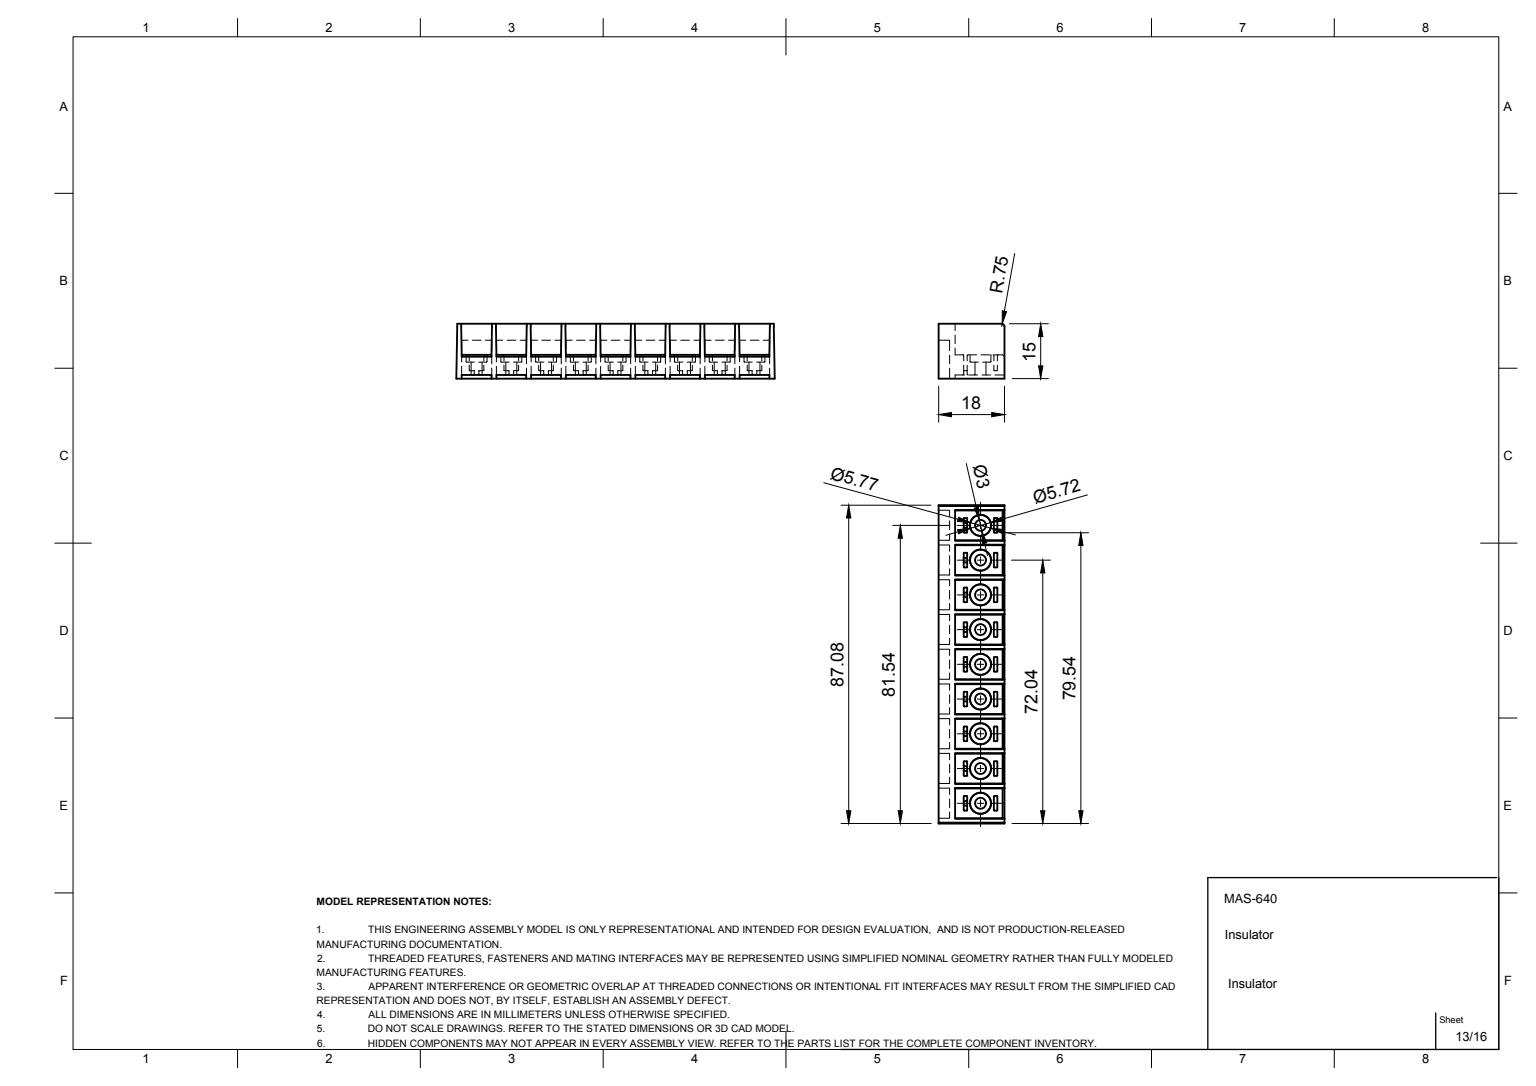
ISO-10303-21;
HEADER;
FILE_DESCRIPTION((''),'2;1');
FILE_NAME('Insulator.step','2026-10-09T10:33:02-07:00',(''),(''),'','','');
FILE_SCHEMA (('AUTOMOTIVE_DESIGN { 1 0 10303 214 3 1 1 }'));
ENDSEC;
DATA;
#10=MECHANICAL_DESIGN_GEOMETRIC_PRESENTATION_REPRESENTATION('',(#842),#86330);
#11=SPHERICAL_SURFACE('',#34725,0.125) ;
#12=SPHERICAL_SURFACE('',#34726,0.125) ;
#13=SPHERICAL_SURFACE('',#34730,0.125) ;
#14=SPHERICAL_SURFACE('',#34731,0.125) ;
#15=SPHERICAL_SURFACE('',#34736,0.125) ;
#16=SPHERICAL_SURFACE('',#34739,0.125) ;
#17=SPHERICAL_SURFACE('',#34750,0.124999999999993) ;
#18=SPHERICAL_SURFACE('',#34751,0.125000000000011) ;
#19=SPHERICAL_SURFACE('',#34781,0.125) ;
#20=SPHERICAL_SURFACE('',#34783,0.125) ;
#21=SPHERICAL_SURFACE('',#34787,0.125) ;
#22=SPHERICAL_SURFACE('',#34789,0.125) ;
#23=SPHERICAL_SURFACE('',#34794,0.125) ;
#24=SPHERICAL_SURFACE('',#34798,0.125) ;
#25=SPHERICAL_SURFACE('',#34810,0.124999999999993) ;
#26=SPHERICAL_SURFACE('',#34811,0.125000000000011) ;
#27=SPHERICAL_SURFACE('',#34841,0.125) ;
#28=SPHERICAL_SURFACE('',#34843,0.125) ;
#29=SPHERICAL_SURFACE('',#34847,0.125) ;
#30=SPHERICAL_SURFACE('',#34849,0.125) ;
#31=SPHERICAL_SURFACE('',#34854,0.125) ;
#32=SPHERICAL_SURFACE('',#34858,0.125) ;
#33=SPHERICAL_SURFACE('',#34870,0.124999999999993) ;
#34=SPHERICAL_SURFACE('',#34871,0.125000000000011) ;
#35=SPHERICAL_SURFACE('',#34901,0.125) ;
#36=SPHERICAL_SURFACE('',#34903,0.125) ;
#37=SPHERICAL_SURFACE('',#34907,0.125) ;
#38=SPHERICAL_SURFACE('',#34909,0.125) ;
#39=SPHERICAL_SURFACE('',#34914,0.125) ;
#40=SPHERICAL_SURFACE('',#34918,0.125) ;
#41=SPHERICAL_SURFACE('',#34930,0.124999999999993) ;
#42=SPHERICAL_SURFACE('',#34931,0.125000000000011) ;
#43=SPHERICAL_SURFACE('',#34961,0.125) ;
#44=SPHERICAL_SURFACE('',#34963,0.125) ;
#45=SPHERICAL_SURFACE('',#34967,0.125) ;
#46=SPHERICAL_SURFACE('',#34969,0.125) ;
#47=SPHERICAL_SURFACE('',#34974,0.125) ;
#48=SPHERICAL_SURFACE('',#34978,0.125) ;
#49=SPHERICAL_SURFACE('',#34990,0.124999999999993) ;
#50=SPHERICAL_SURFACE('',#34991,0.125000000000011) ;
#51=SPHERICAL_SURFACE('',#35021,0.125) ;
#52=SPHERICAL_SURFACE('',#35023,0.125) ;
#53=SPHERICAL_SURFACE('',#35027,0.125) ;
#54=SPHERICAL_SURFACE('',#35029,0.125) ;
#55=SPHERICAL_SURFACE('',#35034,0.125) ;
#56=SPHERICAL_SURFACE('',#35038,0.125) ;
#57=SPHERICAL_SURFACE('',#35050,0.124999999999993) ;
#58=SPHERICAL_SURFACE('',#35051,0.125000000000011) ;
#59=SPHERICAL_SURFACE('',#35081,0.125) ;
#60=SPHERICAL_SURFACE('',#35083,0.125) ;
#61=SPHERICAL_SURFACE('',#35087,0.125) ;
#62=SPHERICAL_SURFACE('',#35089,0.125) ;
#63=SPHERICAL_SURFACE('',#35094,0.125) ;
#64=SPHERICAL_SURFACE('',#35098,0.125) ;
#65=SPHERICAL_SURFACE('',#35110,0.124999999999993) ;
#66=SPHERICAL_SURFACE('',#35111,0.125000000000011) ;
#67=SPHERICAL_SURFACE('',#35141,0.125) ;
#68=SPHERICAL_SURFACE('',#35143,0.125) ;
#69=SPHERICAL_SURFACE('',#35147,0.125) ;
#70=SPHERICAL_SURFACE('',#35149,0.125) ;
#71=SPHERICAL_SURFACE('',#35154,0.125) ;
#72=SPHERICAL_SURFACE('',#35158,0.125) ;
#73=SPHERICAL_SURFACE('',#35170,0.124999999999993) ;
#74=SPHERICAL_SURFACE('',#35171,0.125000000000011) ;
#75=SPHERICAL_SURFACE('',#35201,0.125) ;
#76=SPHERICAL_SURFACE('',#35203,0.125) ;
#77=SPHERICAL_SURFACE('',#35207,0.125) ;
#78=SPHERICAL_SURFACE('',#35209,0.125) ;
#79=SPHERICAL_SURFACE('',#35214,0.125) ;
#80=SPHERICAL_SURFACE('',#35218,0.125) ;
#81=SPHERICAL_SURFACE('',#35230,0.124999999999993) ;
#82=SPHERICAL_SURFACE('',#35231,0.125000000000011) ;
#130=ELLIPSE('',#35261,0.75011424965518,0.750000004857936) ;
#131=ELLIPSE('',#35262,0.750114249654022,0.750000004857117) ;
#132=ELLIPSE('',#35265,0.750114249653564,0.750000004856577) ;
#133=ELLIPSE('',#35266,0.75011424965434,0.750000004857177) ;
#134=ELLIPSE('',#35268,0.750114249655181,0.750000004857937) ;
#135=ELLIPSE('',#35269,0.750114249654116,0.750000004857023) ;
#136=ELLIPSE('',#35271,0.75011424965372,0.750000004856674) ;
#137=ELLIPSE('',#35272,0.75011424965532,0.750000004858217) ;
#138=ELLIPSE('',#35274,0.750114249654022,0.750000004857117) ;
#139=ELLIPSE('',#35275,0.750114249656223,0.750000004858968) ;
#140=ELLIPSE('',#35277,0.750114249654019,0.750000004856718) ;
#141=ELLIPSE('',#35278,0.750114249655222,0.750000004857992) ;
#142=ELLIPSE('',#35280,0.750114249654021,0.750000004856918) ;
#143=ELLIPSE('',#35281,0.750114249656024,0.750000004858698) ;
#144=ELLIPSE('',#35283,0.750114249655273,0.75000000485804) ;
#145=ELLIPSE('',#35284,0.750114249653565,0.75000000485638) ;
#146=ELLIPSE('',#35286,0.750114249654481,0.750000004857962) ;
#147=ELLIPSE('',#35287,0.750114249650677,0.750000004854032) ;
#148=ELLIPSE('',#35289,0.750114249654021,0.750000004856918) ;
#149=ELLIPSE('',#35291,0.750114249654338,0.750000004857176) ;
#239=TOROIDAL_SURFACE('',#33756,1.625,0.125) ;
#240=TOROIDAL_SURFACE('',#33767,1.625,0.125) ;
#241=TOROIDAL_SURFACE('',#33778,1.625,0.125) ;
#242=TOROIDAL_SURFACE('',#33789,1.625,0.125) ;
#243=TOROIDAL_SURFACE('',#33800,1.625,0.125) ;
#244=TOROIDAL_SURFACE('',#33811,1.625,0.125) ;
#245=TOROIDAL_SURFACE('',#33822,1.625,0.125) ;
#246=TOROIDAL_SURFACE('',#33833,1.625,0.125) ;
#247=TOROIDAL_SURFACE('',#33844,1.625,0.125) ;
#248=TOROIDAL_SURFACE('',#33874,0.375,0.25) ;
#249=TOROIDAL_SURFACE('',#33879,0.375,0.25) ;
#250=TOROIDAL_SURFACE('',#33884,0.375,0.25) ;
#251=TOROIDAL_SURFACE('',#33889,0.375,0.25) ;
#252=TOROIDAL_SURFACE('',#33902,0.375,0.25) ;
#253=TOROIDAL_SURFACE('',#33907,0.375,0.25) ;
#254=TOROIDAL_SURFACE('',#33912,0.375,0.25) ;
#255=TOROIDAL_SURFACE('',#33917,0.375,0.25) ;
#256=TOROIDAL_SURFACE('',#33930,0.375,0.25) ;
#257=TOROIDAL_SURFACE('',#33935,0.375,0.25) ;
#258=TOROIDAL_SURFACE('',#33940,0.375,0.25) ;
#259=TOROIDAL_SURFACE('',#33945,0.375,0.25) ;
#260=TOROIDAL_SURFACE('',#33958,0.375,0.25) ;
#261=TOROIDAL_SURFACE('',#33963,0.375,0.25) ;
#262=TOROIDAL_SURFACE('',#33968,0.375,0.25) ;
#263=TOROIDAL_SURFACE('',#33973,0.375,0.25) ;
#264=TOROIDAL_SURFACE('',#33986,0.375,0.25) ;
#265=TOROIDAL_SURFACE('',#33991,0.375,0.25) ;
#266=TOROIDAL_SURFACE('',#33996,0.375,0.25) ;
#267=TOROIDAL_SURFACE('',#34001,0.375,0.25) ;
#268=TOROIDAL_SURFACE('',#34014,0.375,0.25) ;
#269=TOROIDAL_SURFACE('',#34019,0.375,0.25) ;
#270=TOROIDAL_SURFACE('',#34024,0.375,0.25) ;
#271=TOROIDAL_SURFACE('',#34029,0.375,0.25) ;
#272=TOROIDAL_SURFACE('',#34042,0.375,0.25) ;
#273=TOROIDAL_SURFACE('',#34047,0.375,0.25) ;
#274=TOROIDAL_SURFACE('',#34052,0.375,0.25) ;
#275=TOROIDAL_SURFACE('',#34057,0.375,0.25) ;
#276=TOROIDAL_SURFACE('',#34070,0.375,0.25) ;
#277=TOROIDAL_SURFACE('',#34075,0.375,0.25) ;
#278=TOROIDAL_SURFACE('',#34080,0.375,0.25) ;
#279=TOROIDAL_SURFACE('',#34085,0.375,0.25) ;
#280=TOROIDAL_SURFACE('',#34098,0.375,0.25) ;
#281=TOROIDAL_SURFACE('',#34103,0.375,0.25) ;
#282=TOROIDAL_SURFACE('',#34108,0.375,0.25) ;
#283=TOROIDAL_SURFACE('',#34113,0.375,0.25) ;
#284=TOROIDAL_SURFACE('',#34126,0.375,0.25) ;
#285=TOROIDAL_SURFACE('',#34132,0.375,0.25) ;
#286=TOROIDAL_SURFACE('',#34138,0.375,0.25) ;
#287=TOROIDAL_SURFACE('',#34144,0.375,0.25) ;
#288=TOROIDAL_SURFACE('',#34156,0.375,0.25) ;
#289=TOROIDAL_SURFACE('',#34162,0.375,0.25) ;
#290=TOROIDAL_SURFACE('',#34168,0.375,0.25) ;
#291=TOROIDAL_SURFACE('',#34174,0.375,0.25) ;
#292=TOROIDAL_SURFACE('',#34186,0.375,0.25) ;
#293=TOROIDAL_SURFACE('',#34192,0.375,0.25) ;
#294=TOROIDAL_SURFACE('',#34198,0.375,0.25) ;
#295=TOROIDAL_SURFACE('',#34204,0.375,0.25) ;
#296=TOROIDAL_SURFACE('',#34216,0.375,0.25) ;
#297=TOROIDAL_SURFACE('',#34222,0.375,0.25) ;
#298=TOROIDAL_SURFACE('',#34228,0.375,0.25) ;
#299=TOROIDAL_SURFACE('',#34234,0.375,0.25) ;
#300=TOROIDAL_SURFACE('',#34246,0.375,0.25) ;
#301=TOROIDAL_SURFACE('',#34252,0.375,0.25) ;
#302=TOROIDAL_SURFACE('',#34258,0.375,0.25) ;
#303=TOROIDAL_SURFACE('',#34264,0.375,0.25) ;
#304=TOROIDAL_SURFACE('',#34276,0.375,0.25) ;
#305=TOROIDAL_SURFACE('',#34282,0.375,0.25) ;
#306=TOROIDAL_SURFACE('',#34288,0.375,0.25) ;
#307=TOROIDAL_SURFACE('',#34294,0.375,0.25) ;
#308=TOROIDAL_SURFACE('',#34306,0.375,0.25) ;
#309=TOROIDAL_SURFACE('',#34312,0.375,0.25) ;
#310=TOROIDAL_SURFACE('',#34318,0.375,0.25) ;
#311=TOROIDAL_SURFACE('',#34324,0.375,0.25) ;
#312=TOROIDAL_SURFACE('',#34336,0.375,0.25) ;
#313=TOROIDAL_SURFACE('',#34342,0.375,0.25) ;
#314=TOROIDAL_SURFACE('',#34348,0.375,0.25) ;
#315=TOROIDAL_SURFACE('',#34354,0.375,0.25) ;
#316=TOROIDAL_SURFACE('',#34366,0.375,0.25) ;
#317=TOROIDAL_SURFACE('',#34372,0.375,0.25) ;
#318=TOROIDAL_SURFACE('',#34378,0.375,0.25) ;
#319=TOROIDAL_SURFACE('',#34384,0.375,0.25) ;
#320=TOROIDAL_SURFACE('',#34398,0.375,0.25) ;
#321=TOROIDAL_SURFACE('',#34404,0.375,0.25) ;
#322=TOROIDAL_SURFACE('',#34410,0.375,0.25) ;
#323=TOROIDAL_SURFACE('',#34416,0.375,0.25) ;
#324=TOROIDAL_SURFACE('',#34430,0.375,0.25) ;
#325=TOROIDAL_SURFACE('',#34436,0.375,0.25) ;
#326=TOROIDAL_SURFACE('',#34442,0.375,0.25) ;
#327=TOROIDAL_SURFACE('',#34448,0.375,0.25) ;
#328=TOROIDAL_SURFACE('',#34462,0.375,0.25) ;
#329=TOROIDAL_SURFACE('',#34468,0.375,0.25) ;
#330=TOROIDAL_SURFACE('',#34474,0.375,0.25) ;
#331=TOROIDAL_SURFACE('',#34480,0.375,0.25) ;
#332=TOROIDAL_SURFACE('',#34494,0.375,0.25) ;
#333=TOROIDAL_SURFACE('',#34500,0.375,0.25) ;
#334=TOROIDAL_SURFACE('',#34506,0.375,0.25) ;
#335=TOROIDAL_SURFACE('',#34512,0.375,0.25) ;
#336=TOROIDAL_SURFACE('',#34526,0.375,0.25) ;
#337=TOROIDAL_SURFACE('',#34532,0.375,0.25) ;
#338=TOROIDAL_SURFACE('',#34538,0.375,0.25) ;
#339=TOROIDAL_SURFACE('',#34544,0.375,0.25) ;
#340=TOROIDAL_SURFACE('',#34558,0.375,0.25) ;
#341=TOROIDAL_SURFACE('',#34564,0.375,0.25) ;
#342=TOROIDAL_SURFACE('',#34570,0.375,0.25) ;
#343=TOROIDAL_SURFACE('',#34576,0.375,0.25) ;
#344=TOROIDAL_SURFACE('',#34590,0.375,0.25) ;
#345=TOROIDAL_SURFACE('',#34596,0.375,0.25) ;
#346=TOROIDAL_SURFACE('',#34602,0.375,0.25) ;
#347=TOROIDAL_SURFACE('',#34608,0.375,0.25) ;
#348=TOROIDAL_SURFACE('',#34622,0.375,0.25) ;
#349=TOROIDAL_SURFACE('',#34628,0.375,0.25) ;
#350=TOROIDAL_SURFACE('',#34634,0.375,0.25) ;
#351=TOROIDAL_SURFACE('',#34640,0.375,0.25) ;
#352=TOROIDAL_SURFACE('',#34658,0.375,0.25) ;
#353=TOROIDAL_SURFACE('',#34663,0.375,0.25) ;
#354=TOROIDAL_SURFACE('',#34668,0.375,0.25) ;
#355=TOROIDAL_SURFACE('',#34673,0.375,0.25) ;
#356=TOROIDAL_SURFACE('',#34701,0.188499999999969,0.124999999999993) ;
#357=TOROIDAL_SURFACE('',#34706,0.188499999999987,0.124999999999993) ;
#358=TOROIDAL_SURFACE('',#34709,0.188499999999987,0.124999999999993) ;
#359=TOROIDAL_SURFACE('',#34716,0.188499999999987,0.124999999999993) ;
#360=TOROIDAL_SURFACE('',#34757,0.188499999999969,0.124999999999993) ;
#361=TOROIDAL_SURFACE('',#34762,0.188499999999987,0.124999999999993) ;
#362=TOROIDAL_SURFACE('',#34765,0.188499999999987,0.124999999999993) ;
#363=TOROIDAL_SURFACE('',#34772,0.188499999999987,0.124999999999993) ;
#364=TOROIDAL_SURFACE('',#34817,0.188499999999969,0.124999999999993) ;
#365=TOROIDAL_SURFACE('',#34822,0.188499999999987,0.124999999999993) ;
#366=TOROIDAL_SURFACE('',#34825,0.188499999999987,0.124999999999993) ;
#367=TOROIDAL_SURFACE('',#34832,0.188499999999987,0.124999999999993) ;
#368=TOROIDAL_SURFACE('',#34877,0.188499999999969,0.124999999999993) ;
#369=TOROIDAL_SURFACE('',#34882,0.188499999999987,0.124999999999993) ;
#370=TOROIDAL_SURFACE('',#34885,0.188499999999987,0.124999999999993) ;
#371=TOROIDAL_SURFACE('',#34892,0.188499999999987,0.124999999999993) ;
#372=TOROIDAL_SURFACE('',#34937,0.188499999999969,0.124999999999993) ;
#373=TOROIDAL_SURFACE('',#34942,0.188499999999987,0.124999999999993) ;
#374=TOROIDAL_SURFACE('',#34945,0.188499999999987,0.124999999999993) ;
#375=TOROIDAL_SURFACE('',#34952,0.188499999999987,0.124999999999993) ;
#376=TOROIDAL_SURFACE('',#34997,0.188499999999969,0.124999999999993) ;
#377=TOROIDAL_SURFACE('',#35002,0.188499999999987,0.124999999999993) ;
#378=TOROIDAL_SURFACE('',#35005,0.188499999999987,0.124999999999993) ;
#379=TOROIDAL_SURFACE('',#35012,0.188499999999987,0.124999999999993) ;
#380=TOROIDAL_SURFACE('',#35057,0.188499999999969,0.124999999999993) ;
#381=TOROIDAL_SURFACE('',#35062,0.188499999999987,0.124999999999993) ;
#382=TOROIDAL_SURFACE('',#35065,0.188499999999987,0.124999999999993) ;
#383=TOROIDAL_SURFACE('',#35072,0.188499999999987,0.124999999999993) ;
#384=TOROIDAL_SURFACE('',#35117,0.188499999999969,0.124999999999993) ;
#385=TOROIDAL_SURFACE('',#35122,0.188499999999987,0.124999999999993) ;
#386=TOROIDAL_SURFACE('',#35125,0.188499999999987,0.124999999999993) ;
#387=TOROIDAL_SURFACE('',#35132,0.188499999999987,0.124999999999993) ;
#388=TOROIDAL_SURFACE('',#35177,0.188499999999969,0.124999999999993) ;
#389=TOROIDAL_SURFACE('',#35182,0.188499999999987,0.124999999999993) ;
#390=TOROIDAL_SURFACE('',#35185,0.188499999999987,0.124999999999993) ;
#391=TOROIDAL_SURFACE('',#35192,0.188499999999987,0.124999999999993) ;
#392=TOROIDAL_SURFACE('',#35330,2.9825,0.125) ;
#393=TOROIDAL_SURFACE('',#35336,2.7325,0.125) ;
#394=TOROIDAL_SURFACE('',#35342,2.9825,0.125) ;
#395=TOROIDAL_SURFACE('',#35348,2.7325,0.125) ;
#396=TOROIDAL_SURFACE('',#35354,2.9825,0.125) ;
#397=TOROIDAL_SURFACE('',#35360,2.7325,0.125) ;
#398=TOROIDAL_SURFACE('',#35366,2.9825,0.125) ;
#399=TOROIDAL_SURFACE('',#35372,2.7325,0.125) ;
#400=TOROIDAL_SURFACE('',#35378,2.9825,0.125) ;
#401=TOROIDAL_SURFACE('',#35384,2.7325,0.125) ;
#402=TOROIDAL_SURFACE('',#35390,2.9825,0.125) ;
#403=TOROIDAL_SURFACE('',#35396,2.7325,0.125) ;
#404=TOROIDAL_SURFACE('',#35402,2.9825,0.125) ;
#405=TOROIDAL_SURFACE('',#35408,2.7325,0.125) ;
#406=TOROIDAL_SURFACE('',#35414,2.9825,0.125) ;
#407=TOROIDAL_SURFACE('',#35420,2.7325,0.125) ;
#408=TOROIDAL_SURFACE('',#35424,2.9825,0.125) ;
#409=TOROIDAL_SURFACE('',#35430,2.7325,0.125) ;
#818=SHAPE_REPRESENTATION_RELATIONSHIP('SRR','None',#86461,#830) ;
#830=ADVANCED_BREP_SHAPE_REPRESENTATION('',(#854),#86315) ;
#842=STYLED_ITEM('',(#86583),#854) ;
#854=MANIFOLD_SOLID_BREP('Body1',#32641) ;
#1115=FACE_BOUND('',#4823,.T.) ;
#1116=FACE_BOUND('',#4824,.T.) ;
#1117=FACE_BOUND('',#4828,.T.) ;
#1118=FACE_BOUND('',#4829,.T.) ;
#1119=FACE_BOUND('',#4833,.T.) ;
#1120=FACE_BOUND('',#4834,.T.) ;
#1121=FACE_BOUND('',#4838,.T.) ;
#1122=FACE_BOUND('',#4839,.T.) ;
#1123=FACE_BOUND('',#4843,.T.) ;
#1124=FACE_BOUND('',#4844,.T.) ;
#1125=FACE_BOUND('',#4848,.T.) ;
#1126=FACE_BOUND('',#4849,.T.) ;
#1127=FACE_BOUND('',#4853,.T.) ;
#1128=FACE_BOUND('',#4854,.T.) ;
#1129=FACE_BOUND('',#4858,.T.) ;
#1130=FACE_BOUND('',#4859,.T.) ;
#1131=FACE_BOUND('',#4862,.T.) ;
#1132=FACE_BOUND('',#4863,.T.) ;
#1133=FACE_BOUND('',#4866,.T.) ;
#1134=FACE_BOUND('',#4868,.T.) ;
#1135=FACE_BOUND('',#4870,.T.) ;
#1136=FACE_BOUND('',#4872,.T.) ;
#1137=FACE_BOUND('',#4874,.T.) ;
#1138=FACE_BOUND('',#4876,.T.) ;
#1139=FACE_BOUND('',#4878,.T.) ;
#1140=FACE_BOUND('',#4880,.T.) ;
#1141=FACE_BOUND('',#5194,.T.) ;
#1142=FACE_BOUND('',#5195,.T.) ;
#1143=FACE_BOUND('',#5196,.T.) ;
#1144=FACE_BOUND('',#5217,.T.) ;
#1145=FACE_BOUND('',#5565,.T.) ;
#1146=FACE_BOUND('',#5566,.T.) ;
#1147=FACE_BOUND('',#5567,.T.) ;
#1148=FACE_BOUND('',#5574,.T.) ;
#1149=FACE_BOUND('',#5575,.T.) ;
#1150=FACE_BOUND('',#5576,.T.) ;
#1151=FACE_BOUND('',#5583,.T.) ;
#1152=FACE_BOUND('',#5584,.T.) ;
#1153=FACE_BOUND('',#5585,.T.) ;
#1154=FACE_BOUND('',#5592,.T.) ;
#1155=FACE_BOUND('',#5593,.T.) ;
#1156=FACE_BOUND('',#5594,.T.) ;
#1157=FACE_BOUND('',#5601,.T.) ;
#1158=FACE_BOUND('',#5602,.T.) ;
#1159=FACE_BOUND('',#5603,.T.) ;
#1160=FACE_BOUND('',#5610,.T.) ;
#1161=FACE_BOUND('',#5611,.T.) ;
#1162=FACE_BOUND('',#5612,.T.) ;
#1163=FACE_BOUND('',#5619,.T.) ;
#1164=FACE_BOUND('',#5620,.T.) ;
#1165=FACE_BOUND('',#5621,.T.) ;
#1166=FACE_BOUND('',#5628,.T.) ;
#1167=FACE_BOUND('',#5629,.T.) ;
#1168=FACE_BOUND('',#5630,.T.) ;
#1899=PLANE('',#33719) ;
#1900=PLANE('',#33720) ;
#1901=PLANE('',#33721) ;
#1902=PLANE('',#33722) ;
#1903=PLANE('',#33723) ;
#1904=PLANE('',#33724) ;
#1905=PLANE('',#33725) ;
#1906=PLANE('',#33726) ;
#1907=PLANE('',#33727) ;
#1908=PLANE('',#33728) ;
#1909=PLANE('',#33729) ;
#1910=PLANE('',#33730) ;
#1911=PLANE('',#33731) ;
#1912=PLANE('',#33732) ;
#1913=PLANE('',#33733) ;
#1914=PLANE('',#33734) ;
#1915=PLANE('',#33735) ;
#1916=PLANE('',#33736) ;
#1917=PLANE('',#33737) ;
#1918=PLANE('',#33738) ;
#1919=PLANE('',#33739) ;
#1920=PLANE('',#33740) ;
#1921=PLANE('',#33741) ;
#1922=PLANE('',#33742) ;
#1923=PLANE('',#33743) ;
#1924=PLANE('',#33744) ;
#1925=PLANE('',#33745) ;
#1926=PLANE('',#33746) ;
#1927=PLANE('',#33747) ;
#1928=PLANE('',#33748) ;
#1929=PLANE('',#33749) ;
#1930=PLANE('',#33750) ;
#1931=PLANE('',#33751) ;
#1932=PLANE('',#33752) ;
#1933=PLANE('',#33753) ;
#1934=PLANE('',#33754) ;
#1935=PLANE('',#33755) ;
#1936=PLANE('',#33762) ;
#1937=PLANE('',#33773) ;
#1938=PLANE('',#33784) ;
#1939=PLANE('',#33795) ;
#1940=PLANE('',#33806) ;
#1941=PLANE('',#33817) ;
#1942=PLANE('',#33828) ;
#1943=PLANE('',#33839) ;
#1944=PLANE('',#33848) ;
#1945=PLANE('',#33855) ;
#1946=PLANE('',#33857) ;
#1947=PLANE('',#33859) ;
#1948=PLANE('',#33861) ;
#1949=PLANE('',#33863) ;
#1950=PLANE('',#33865) ;
#1951=PLANE('',#33867) ;
#1952=PLANE('',#33869) ;
#1953=PLANE('',#33893) ;
#1954=PLANE('',#33898) ;
#1955=PLANE('',#33921) ;
#1956=PLANE('',#33926) ;
#1957=PLANE('',#33949) ;
#1958=PLANE('',#33954) ;
#1959=PLANE('',#33977) ;
#1960=PLANE('',#33982) ;
#1961=PLANE('',#34005) ;
#1962=PLANE('',#34010) ;
#1963=PLANE('',#34033) ;
#1964=PLANE('',#34038) ;
#1965=PLANE('',#34061) ;
#1966=PLANE('',#34066) ;
#1967=PLANE('',#34089) ;
#1968=PLANE('',#34094) ;
#1969=PLANE('',#34117) ;
#1970=PLANE('',#34122) ;
#1971=PLANE('',#34149) ;
#1972=PLANE('',#34152) ;
#1973=PLANE('',#34179) ;
#1974=PLANE('',#34182) ;
#1975=PLANE('',#34209) ;
#1976=PLANE('',#34212) ;
#1977=PLANE('',#34239) ;
#1978=PLANE('',#34242) ;
#1979=PLANE('',#34269) ;
#1980=PLANE('',#34272) ;
#1981=PLANE('',#34299) ;
#1982=PLANE('',#34302) ;
#1983=PLANE('',#34329) ;
#1984=PLANE('',#34332) ;
#1985=PLANE('',#34359) ;
#1986=PLANE('',#34362) ;
#1987=PLANE('',#34389) ;
#1988=PLANE('',#34394) ;
#1989=PLANE('',#34421) ;
#1990=PLANE('',#34426) ;
#1991=PLANE('',#34453) ;
#1992=PLANE('',#34458) ;
#1993=PLANE('',#34485) ;
#1994=PLANE('',#34490) ;
#1995=PLANE('',#34517) ;
#1996=PLANE('',#34522) ;
#1997=PLANE('',#34549) ;
#1998=PLANE('',#34554) ;
#1999=PLANE('',#34581) ;
#2000=PLANE('',#34586) ;
#2001=PLANE('',#34613) ;
#2002=PLANE('',#34618) ;
#2003=PLANE('',#34645) ;
#2004=PLANE('',#34648) ;
#2005=PLANE('',#34649) ;
#2006=PLANE('',#34677) ;
#2007=PLANE('',#34682) ;
#2008=PLANE('',#34683) ;
#2009=PLANE('',#34688) ;
#2010=PLANE('',#34693) ;
#2011=PLANE('',#34694) ;
#2012=PLANE('',#34732) ;
#2013=PLANE('',#34733) ;
#2014=PLANE('',#34734) ;
#2015=PLANE('',#34735) ;
#2016=PLANE('',#34790) ;
#2017=PLANE('',#34791) ;
#2018=PLANE('',#34792) ;
#2019=PLANE('',#34793) ;
#2020=PLANE('',#34850) ;
#2021=PLANE('',#34851) ;
#2022=PLANE('',#34852) ;
#2023=PLANE('',#34853) ;
#2024=PLANE('',#34910) ;
#2025=PLANE('',#34911) ;
#2026=PLANE('',#34912) ;
#2027=PLANE('',#34913) ;
#2028=PLANE('',#34970) ;
#2029=PLANE('',#34971) ;
#2030=PLANE('',#34972) ;
#2031=PLANE('',#34973) ;
#2032=PLANE('',#35030) ;
#2033=PLANE('',#35031) ;
#2034=PLANE('',#35032) ;
#2035=PLANE('',#35033) ;
#2036=PLANE('',#35090) ;
#2037=PLANE('',#35091) ;
#2038=PLANE('',#35092) ;
#2039=PLANE('',#35093) ;
#2040=PLANE('',#35150) ;
#2041=PLANE('',#35151) ;
#2042=PLANE('',#35152) ;
#2043=PLANE('',#35153) ;
#2044=PLANE('',#35210) ;
#2045=PLANE('',#35211) ;
#2046=PLANE('',#35212) ;
#2047=PLANE('',#35213) ;
#2048=PLANE('',#35232) ;
#2049=PLANE('',#35233) ;
#2050=PLANE('',#35234) ;
#2051=PLANE('',#35235) ;
#2052=PLANE('',#35236) ;
#2053=PLANE('',#35237) ;
#2054=PLANE('',#35238) ;
#2055=PLANE('',#35239) ;
#2056=PLANE('',#35240) ;
#2057=PLANE('',#35241) ;
#2058=PLANE('',#35242) ;
#2059=PLANE('',#35243) ;
#2060=PLANE('',#35244) ;
#2061=PLANE('',#35245) ;
#2062=PLANE('',#35246) ;
#2063=PLANE('',#35247) ;
#2064=PLANE('',#35248) ;
#2065=PLANE('',#35249) ;
#2066=PLANE('',#35250) ;
#2067=PLANE('',#35251) ;
#2068=PLANE('',#35252) ;
#2069=PLANE('',#35253) ;
#2070=PLANE('',#35254) ;
#2071=PLANE('',#35255) ;
#2072=PLANE('',#35256) ;
#2073=PLANE('',#35257) ;
#2074=PLANE('',#35258) ;
#2075=PLANE('',#35259) ;
#2076=PLANE('',#35263) ;
#2077=PLANE('',#35288) ;
#2078=PLANE('',#35292) ;
#2079=PLANE('',#35293) ;
#2080=PLANE('',#35294) ;
#2081=PLANE('',#35295) ;
#2082=PLANE('',#35296) ;
#2083=PLANE('',#35297) ;
#2084=PLANE('',#35298) ;
#2085=PLANE('',#35299) ;
#2086=PLANE('',#35300) ;
#2087=PLANE('',#35301) ;
#2088=PLANE('',#35302) ;
#2089=PLANE('',#35303) ;
#2090=PLANE('',#35304) ;
#2091=PLANE('',#35305) ;
#2092=PLANE('',#35306) ;
#2093=PLANE('',#35307) ;
#2094=PLANE('',#35308) ;
#2095=PLANE('',#35309) ;
#2096=PLANE('',#35310) ;
#2097=PLANE('',#35311) ;
#2098=PLANE('',#35312) ;
#2099=PLANE('',#35313) ;
#2100=PLANE('',#35314) ;
#2101=PLANE('',#35315) ;
#2102=PLANE('',#35316) ;
#2103=PLANE('',#35317) ;
#2104=PLANE('',#35318) ;
#2105=PLANE('',#35319) ;
#2106=PLANE('',#35320) ;
#2107=PLANE('',#35321) ;
#2108=PLANE('',#35322) ;
#2109=PLANE('',#35323) ;
#2110=PLANE('',#35324) ;
#2111=PLANE('',#35325) ;
#2112=PLANE('',#35326) ;
#2113=PLANE('',#35327) ;
#2114=PLANE('',#35328) ;
#2115=PLANE('',#35338) ;
#2116=PLANE('',#35340) ;
#2117=PLANE('',#35350) ;
#2118=PLANE('',#35352) ;
#2119=PLANE('',#35362) ;
#2120=PLANE('',#35364) ;
#2121=PLANE('',#35374) ;
#2122=PLANE('',#35376) ;
#2123=PLANE('',#35386) ;
#2124=PLANE('',#35388) ;
#2125=PLANE('',#35398) ;
#2126=PLANE('',#35400) ;
#2127=PLANE('',#35410) ;
#2128=PLANE('',#35412) ;
#2129=PLANE('',#35422) ;
#2130=PLANE('',#35432) ;
#2131=PLANE('',#35433) ;
#2132=PLANE('',#35435) ;
#2133=PLANE('',#35437) ;
#2134=PLANE('',#35440) ;
#2135=PLANE('',#35442) ;
#2136=PLANE('',#35445) ;
#2137=PLANE('',#35447) ;
#2138=PLANE('',#35450) ;
#2139=PLANE('',#35452) ;
#2140=PLANE('',#35455) ;
#2141=PLANE('',#35457) ;
#2142=PLANE('',#35460) ;
#2143=PLANE('',#35462) ;
#2144=PLANE('',#35465) ;
#2145=PLANE('',#35467) ;
#2146=PLANE('',#35470) ;
#2147=PLANE('',#35472) ;
#2780=FACE_OUTER_BOUND('',#4783,.T.) ;
#2781=FACE_OUTER_BOUND('',#4784,.T.) ;
#2782=FACE_OUTER_BOUND('',#4785,.T.) ;
#2783=FACE_OUTER_BOUND('',#4786,.T.) ;
#2784=FACE_OUTER_BOUND('',#4787,.T.) ;
#2785=FACE_OUTER_BOUND('',#4788,.T.) ;
#2786=FACE_OUTER_BOUND('',#4789,.T.) ;
#2787=FACE_OUTER_BOUND('',#4790,.T.) ;
#2788=FACE_OUTER_BOUND('',#4791,.T.) ;
#2789=FACE_OUTER_BOUND('',#4792,.T.) ;
#2790=FACE_OUTER_BOUND('',#4793,.T.) ;
#2791=FACE_OUTER_BOUND('',#4794,.T.) ;
#2792=FACE_OUTER_BOUND('',#4795,.T.) ;
#2793=FACE_OUTER_BOUND('',#4796,.T.) ;
#2794=FACE_OUTER_BOUND('',#4797,.T.) ;
#2795=FACE_OUTER_BOUND('',#4798,.T.) ;
#2796=FACE_OUTER_BOUND('',#4799,.T.) ;
#2797=FACE_OUTER_BOUND('',#4800,.T.) ;
#2798=FACE_OUTER_BOUND('',#4801,.T.) ;
#2799=FACE_OUTER_BOUND('',#4802,.T.) ;
#2800=FACE_OUTER_BOUND('',#4803,.T.) ;
#2801=FACE_OUTER_BOUND('',#4804,.T.) ;
#2802=FACE_OUTER_BOUND('',#4805,.T.) ;
#2803=FACE_OUTER_BOUND('',#4806,.T.) ;
#2804=FACE_OUTER_BOUND('',#4807,.T.) ;
#2805=FACE_OUTER_BOUND('',#4808,.T.) ;
#2806=FACE_OUTER_BOUND('',#4809,.T.) ;
#2807=FACE_OUTER_BOUND('',#4810,.T.) ;
#2808=FACE_OUTER_BOUND('',#4811,.T.) ;
#2809=FACE_OUTER_BOUND('',#4812,.T.) ;
#2810=FACE_OUTER_BOUND('',#4813,.T.) ;
#2811=FACE_OUTER_BOUND('',#4814,.T.) ;
#2812=FACE_OUTER_BOUND('',#4815,.T.) ;
#2813=FACE_OUTER_BOUND('',#4816,.T.) ;
#2814=FACE_OUTER_BOUND('',#4817,.T.) ;
#2815=FACE_OUTER_BOUND('',#4818,.T.) ;
#2816=FACE_OUTER_BOUND('',#4819,.T.) ;
#2817=FACE_OUTER_BOUND('',#4820,.T.) ;
#2818=FACE_OUTER_BOUND('',#4821,.T.) ;
#2819=FACE_OUTER_BOUND('',#4822,.T.) ;
#2820=FACE_OUTER_BOUND('',#4825,.T.) ;
#2821=FACE_OUTER_BOUND('',#4826,.T.) ;
#2822=FACE_OUTER_BOUND('',#4827,.T.) ;
#2823=FACE_OUTER_BOUND('',#4830,.T.) ;
#2824=FACE_OUTER_BOUND('',#4831,.T.) ;
#2825=FACE_OUTER_BOUND('',#4832,.T.) ;
#2826=FACE_OUTER_BOUND('',#4835,.T.) ;
#2827=FACE_OUTER_BOUND('',#4836,.T.) ;
#2828=FACE_OUTER_BOUND('',#4837,.T.) ;
#2829=FACE_OUTER_BOUND('',#4840,.T.) ;
#2830=FACE_OUTER_BOUND('',#4841,.T.) ;
#2831=FACE_OUTER_BOUND('',#4842,.T.) ;
#2832=FACE_OUTER_BOUND('',#4845,.T.) ;
#2833=FACE_OUTER_BOUND('',#4846,.T.) ;
#2834=FACE_OUTER_BOUND('',#4847,.T.) ;
#2835=FACE_OUTER_BOUND('',#4850,.T.) ;
#2836=FACE_OUTER_BOUND('',#4851,.T.) ;
#2837=FACE_OUTER_BOUND('',#4852,.T.) ;
#2838=FACE_OUTER_BOUND('',#4855,.T.) ;
#2839=FACE_OUTER_BOUND('',#4856,.T.) ;
#2840=FACE_OUTER_BOUND('',#4857,.T.) ;
#2841=FACE_OUTER_BOUND('',#4860,.T.) ;
#2842=FACE_OUTER_BOUND('',#4861,.T.) ;
#2843=FACE_OUTER_BOUND('',#4864,.T.) ;
#2844=FACE_OUTER_BOUND('',#4865,.T.) ;
#2845=FACE_OUTER_BOUND('',#4867,.T.) ;
#2846=FACE_OUTER_BOUND('',#4869,.T.) ;
#2847=FACE_OUTER_BOUND('',#4871,.T.) ;
#2848=FACE_OUTER_BOUND('',#4873,.T.) ;
#2849=FACE_OUTER_BOUND('',#4875,.T.) ;
#2850=FACE_OUTER_BOUND('',#4877,.T.) ;
#2851=FACE_OUTER_BOUND('',#4879,.T.) ;
#2852=FACE_OUTER_BOUND('',#4881,.T.) ;
#2853=FACE_OUTER_BOUND('',#4882,.T.) ;
#2854=FACE_OUTER_BOUND('',#4883,.T.) ;
#2855=FACE_OUTER_BOUND('',#4884,.T.) ;
#2856=FACE_OUTER_BOUND('',#4885,.T.) ;
#2857=FACE_OUTER_BOUND('',#4886,.T.) ;
#2858=FACE_OUTER_BOUND('',#4887,.T.) ;
#2859=FACE_OUTER_BOUND('',#4888,.T.) ;
#2860=FACE_OUTER_BOUND('',#4889,.T.) ;
#2861=FACE_OUTER_BOUND('',#4890,.T.) ;
#2862=FACE_OUTER_BOUND('',#4891,.T.) ;
#2863=FACE_OUTER_BOUND('',#4892,.T.) ;
#2864=FACE_OUTER_BOUND('',#4893,.T.) ;
#2865=FACE_OUTER_BOUND('',#4894,.T.) ;
#2866=FACE_OUTER_BOUND('',#4895,.T.) ;
#2867=FACE_OUTER_BOUND('',#4896,.T.) ;
#2868=FACE_OUTER_BOUND('',#4897,.T.) ;
#2869=FACE_OUTER_BOUND('',#4898,.T.) ;
#2870=FACE_OUTER_BOUND('',#4899,.T.) ;
#2871=FACE_OUTER_BOUND('',#4900,.T.) ;
#2872=FACE_OUTER_BOUND('',#4901,.T.) ;
#2873=FACE_OUTER_BOUND('',#4902,.T.) ;
#2874=FACE_OUTER_BOUND('',#4903,.T.) ;
#2875=FACE_OUTER_BOUND('',#4904,.T.) ;
#2876=FACE_OUTER_BOUND('',#4905,.T.) ;
#2877=FACE_OUTER_BOUND('',#4906,.T.) ;
#2878=FACE_OUTER_BOUND('',#4907,.T.) ;
#2879=FACE_OUTER_BOUND('',#4908,.T.) ;
#2880=FACE_OUTER_BOUND('',#4909,.T.) ;
#2881=FACE_OUTER_BOUND('',#4910,.T.) ;
#2882=FACE_OUTER_BOUND('',#4911,.T.) ;
#2883=FACE_OUTER_BOUND('',#4912,.T.) ;
#2884=FACE_OUTER_BOUND('',#4913,.T.) ;
#2885=FACE_OUTER_BOUND('',#4914,.T.) ;
#2886=FACE_OUTER_BOUND('',#4915,.T.) ;
#2887=FACE_OUTER_BOUND('',#4916,.T.) ;
#2888=FACE_OUTER_BOUND('',#4917,.T.) ;
#2889=FACE_OUTER_BOUND('',#4918,.T.) ;
#2890=FACE_OUTER_BOUND('',#4919,.T.) ;
#2891=FACE_OUTER_BOUND('',#4920,.T.) ;
#2892=FACE_OUTER_BOUND('',#4921,.T.) ;
#2893=FACE_OUTER_BOUND('',#4922,.T.) ;
#2894=FACE_OUTER_BOUND('',#4923,.T.) ;
#2895=FACE_OUTER_BOUND('',#4924,.T.) ;
#2896=FACE_OUTER_BOUND('',#4925,.T.) ;
#2897=FACE_OUTER_BOUND('',#4926,.T.) ;
#2898=FACE_OUTER_BOUND('',#4927,.T.) ;
#2899=FACE_OUTER_BOUND('',#4928,.T.) ;
#2900=FACE_OUTER_BOUND('',#4929,.T.) ;
#2901=FACE_OUTER_BOUND('',#4930,.T.) ;
#2902=FACE_OUTER_BOUND('',#4931,.T.) ;
#2903=FACE_OUTER_BOUND('',#4932,.T.) ;
#2904=FACE_OUTER_BOUND('',#4933,.T.) ;
#2905=FACE_OUTER_BOUND('',#4934,.T.) ;
#2906=FACE_OUTER_BOUND('',#4935,.T.) ;
#2907=FACE_OUTER_BOUND('',#4936,.T.) ;
#2908=FACE_OUTER_BOUND('',#4937,.T.) ;
#2909=FACE_OUTER_BOUND('',#4938,.T.) ;
#2910=FACE_OUTER_BOUND('',#4939,.T.) ;
#2911=FACE_OUTER_BOUND('',#4940,.T.) ;
#2912=FACE_OUTER_BOUND('',#4941,.T.) ;
#2913=FACE_OUTER_BOUND('',#4942,.T.) ;
#2914=FACE_OUTER_BOUND('',#4943,.T.) ;
#2915=FACE_OUTER_BOUND('',#4944,.T.) ;
#2916=FACE_OUTER_BOUND('',#4945,.T.) ;
#2917=FACE_OUTER_BOUND('',#4946,.T.) ;
#2918=FACE_OUTER_BOUND('',#4947,.T.) ;
#2919=FACE_OUTER_BOUND('',#4948,.T.) ;
#2920=FACE_OUTER_BOUND('',#4949,.T.) ;
#2921=FACE_OUTER_BOUND('',#4950,.T.) ;
#2922=FACE_OUTER_BOUND('',#4951,.T.) ;
#2923=FACE_OUTER_BOUND('',#4952,.T.) ;
#2924=FACE_OUTER_BOUND('',#4953,.T.) ;
#2925=FACE_OUTER_BOUND('',#4954,.T.) ;
#2926=FACE_OUTER_BOUND('',#4955,.T.) ;
#2927=FACE_OUTER_BOUND('',#4956,.T.) ;
#2928=FACE_OUTER_BOUND('',#4957,.T.) ;
#2929=FACE_OUTER_BOUND('',#4958,.T.) ;
#2930=FACE_OUTER_BOUND('',#4959,.T.) ;
#2931=FACE_OUTER_BOUND('',#4960,.T.) ;
#2932=FACE_OUTER_BOUND('',#4961,.T.) ;
#2933=FACE_OUTER_BOUND('',#4962,.T.) ;
#2934=FACE_OUTER_BOUND('',#4963,.T.) ;
#2935=FACE_OUTER_BOUND('',#4964,.T.) ;
#2936=FACE_OUTER_BOUND('',#4965,.T.) ;
#2937=FACE_OUTER_BOUND('',#4966,.T.) ;
#2938=FACE_OUTER_BOUND('',#4967,.T.) ;
#2939=FACE_OUTER_BOUND('',#4968,.T.) ;
#2940=FACE_OUTER_BOUND('',#4969,.T.) ;
#2941=FACE_OUTER_BOUND('',#4970,.T.) ;
#2942=FACE_OUTER_BOUND('',#4971,.T.) ;
#2943=FACE_OUTER_BOUND('',#4972,.T.) ;
#2944=FACE_OUTER_BOUND('',#4973,.T.) ;
#2945=FACE_OUTER_BOUND('',#4974,.T.) ;
#2946=FACE_OUTER_BOUND('',#4975,.T.) ;
#2947=FACE_OUTER_BOUND('',#4976,.T.) ;
#2948=FACE_OUTER_BOUND('',#4977,.T.) ;
#2949=FACE_OUTER_BOUND('',#4978,.T.) ;
#2950=FACE_OUTER_BOUND('',#4979,.T.) ;
#2951=FACE_OUTER_BOUND('',#4980,.T.) ;
#2952=FACE_OUTER_BOUND('',#4981,.T.) ;
#2953=FACE_OUTER_BOUND('',#4982,.T.) ;
#2954=FACE_OUTER_BOUND('',#4983,.T.) ;
#2955=FACE_OUTER_BOUND('',#4984,.T.) ;
#2956=FACE_OUTER_BOUND('',#4985,.T.) ;
#2957=FACE_OUTER_BOUND('',#4986,.T.) ;
#2958=FACE_OUTER_BOUND('',#4987,.T.) ;
#2959=FACE_OUTER_BOUND('',#4988,.T.) ;
#2960=FACE_OUTER_BOUND('',#4989,.T.) ;
#2961=FACE_OUTER_BOUND('',#4990,.T.) ;
#2962=FACE_OUTER_BOUND('',#4991,.T.) ;
#2963=FACE_OUTER_BOUND('',#4992,.T.) ;
#2964=FACE_OUTER_BOUND('',#4993,.T.) ;
#2965=FACE_OUTER_BOUND('',#4994,.T.) ;
#2966=FACE_OUTER_BOUND('',#4995,.T.) ;
#2967=FACE_OUTER_BOUND('',#4996,.T.) ;
#2968=FACE_OUTER_BOUND('',#4997,.T.) ;
#2969=FACE_OUTER_BOUND('',#4998,.T.) ;
#2970=FACE_OUTER_BOUND('',#4999,.T.) ;
#2971=FACE_OUTER_BOUND('',#5000,.T.) ;
#2972=FACE_OUTER_BOUND('',#5001,.T.) ;
#2973=FACE_OUTER_BOUND('',#5002,.T.) ;
#2974=FACE_OUTER_BOUND('',#5003,.T.) ;
#2975=FACE_OUTER_BOUND('',#5004,.T.) ;
#2976=FACE_OUTER_BOUND('',#5005,.T.) ;
#2977=FACE_OUTER_BOUND('',#5006,.T.) ;
#2978=FACE_OUTER_BOUND('',#5007,.T.) ;
#2979=FACE_OUTER_BOUND('',#5008,.T.) ;
#2980=FACE_OUTER_BOUND('',#5009,.T.) ;
#2981=FACE_OUTER_BOUND('',#5010,.T.) ;
#2982=FACE_OUTER_BOUND('',#5011,.T.) ;
#2983=FACE_OUTER_BOUND('',#5012,.T.) ;
#2984=FACE_OUTER_BOUND('',#5013,.T.) ;
#2985=FACE_OUTER_BOUND('',#5014,.T.) ;
#2986=FACE_OUTER_BOUND('',#5015,.T.) ;
#2987=FACE_OUTER_BOUND('',#5016,.T.) ;
#2988=FACE_OUTER_BOUND('',#5017,.T.) ;
#2989=FACE_OUTER_BOUND('',#5018,.T.) ;
#2990=FACE_OUTER_BOUND('',#5019,.T.) ;
#2991=FACE_OUTER_BOUND('',#5020,.T.) ;
#2992=FACE_OUTER_BOUND('',#5021,.T.) ;
#2993=FACE_OUTER_BOUND('',#5022,.T.) ;
#2994=FACE_OUTER_BOUND('',#5023,.T.) ;
#2995=FACE_OUTER_BOUND('',#5024,.T.) ;
#2996=FACE_OUTER_BOUND('',#5025,.T.) ;
#2997=FACE_OUTER_BOUND('',#5026,.T.) ;
#2998=FACE_OUTER_BOUND('',#5027,.T.) ;
#2999=FACE_OUTER_BOUND('',#5028,.T.) ;
#3000=FACE_OUTER_BOUND('',#5029,.T.) ;
#3001=FACE_OUTER_BOUND('',#5030,.T.) ;
#3002=FACE_OUTER_BOUND('',#5031,.T.) ;
#3003=FACE_OUTER_BOUND('',#5032,.T.) ;
#3004=FACE_OUTER_BOUND('',#5033,.T.) ;
#3005=FACE_OUTER_BOUND('',#5034,.T.) ;
#3006=FACE_OUTER_BOUND('',#5035,.T.) ;
#3007=FACE_OUTER_BOUND('',#5036,.T.) ;
#3008=FACE_OUTER_BOUND('',#5037,.T.) ;
#3009=FACE_OUTER_BOUND('',#5038,.T.) ;
#3010=FACE_OUTER_BOUND('',#5039,.T.) ;
#3011=FACE_OUTER_BOUND('',#5040,.T.) ;
#3012=FACE_OUTER_BOUND('',#5041,.T.) ;
#3013=FACE_OUTER_BOUND('',#5042,.T.) ;
#3014=FACE_OUTER_BOUND('',#5043,.T.) ;
#3015=FACE_OUTER_BOUND('',#5044,.T.) ;
#3016=FACE_OUTER_BOUND('',#5045,.T.) ;
#3017=FACE_OUTER_BOUND('',#5046,.T.) ;
#3018=FACE_OUTER_BOUND('',#5047,.T.) ;
#3019=FACE_OUTER_BOUND('',#5048,.T.) ;
#3020=FACE_OUTER_BOUND('',#5049,.T.) ;
#3021=FACE_OUTER_BOUND('',#5050,.T.) ;
#3022=FACE_OUTER_BOUND('',#5051,.T.) ;
#3023=FACE_OUTER_BOUND('',#5052,.T.) ;
#3024=FACE_OUTER_BOUND('',#5053,.T.) ;
#3025=FACE_OUTER_BOUND('',#5054,.T.) ;
#3026=FACE_OUTER_BOUND('',#5055,.T.) ;
#3027=FACE_OUTER_BOUND('',#5056,.T.) ;
#3028=FACE_OUTER_BOUND('',#5057,.T.) ;
#3029=FACE_OUTER_BOUND('',#5058,.T.) ;
#3030=FACE_OUTER_BOUND('',#5059,.T.) ;
#3031=FACE_OUTER_BOUND('',#5060,.T.) ;
#3032=FACE_OUTER_BOUND('',#5061,.T.) ;
#3033=FACE_OUTER_BOUND('',#5062,.T.) ;
#3034=FACE_OUTER_BOUND('',#5063,.T.) ;
#3035=FACE_OUTER_BOUND('',#5064,.T.) ;
#3036=FACE_OUTER_BOUND('',#5065,.T.) ;
#3037=FACE_OUTER_BOUND('',#5066,.T.) ;
#3038=FACE_OUTER_BOUND('',#5067,.T.) ;
#3039=FACE_OUTER_BOUND('',#5068,.T.) ;
#3040=FACE_OUTER_BOUND('',#5069,.T.) ;
#3041=FACE_OUTER_BOUND('',#5070,.T.) ;
#3042=FACE_OUTER_BOUND('',#5071,.T.) ;
#3043=FACE_OUTER_BOUND('',#5072,.T.) ;
#3044=FACE_OUTER_BOUND('',#5073,.T.) ;
#3045=FACE_OUTER_BOUND('',#5074,.T.) ;
#3046=FACE_OUTER_BOUND('',#5075,.T.) ;
#3047=FACE_OUTER_BOUND('',#5076,.T.) ;
#3048=FACE_OUTER_BOUND('',#5077,.T.) ;
#3049=FACE_OUTER_BOUND('',#5078,.T.) ;
#3050=FACE_OUTER_BOUND('',#5079,.T.) ;
#3051=FACE_OUTER_BOUND('',#5080,.T.) ;
#3052=FACE_OUTER_BOUND('',#5081,.T.) ;
#3053=FACE_OUTER_BOUND('',#5082,.T.) ;
#3054=FACE_OUTER_BOUND('',#5083,.T.) ;
#3055=FACE_OUTER_BOUND('',#5084,.T.) ;
#3056=FACE_OUTER_BOUND('',#5085,.T.) ;
#3057=FACE_OUTER_BOUND('',#5086,.T.) ;
#3058=FACE_OUTER_BOUND('',#5087,.T.) ;
#3059=FACE_OUTER_BOUND('',#5088,.T.) ;
#3060=FACE_OUTER_BOUND('',#5089,.T.) ;
#3061=FACE_OUTER_BOUND('',#5090,.T.) ;
#3062=FACE_OUTER_BOUND('',#5091,.T.) ;
#3063=FACE_OUTER_BOUND('',#5092,.T.) ;
#3064=FACE_OUTER_BOUND('',#5093,.T.) ;
#3065=FACE_OUTER_BOUND('',#5094,.T.) ;
#3066=FACE_OUTER_BOUND('',#5095,.T.) ;
#3067=FACE_OUTER_BOUND('',#5096,.T.) ;
#3068=FACE_OUTER_BOUND('',#5097,.T.) ;
#3069=FACE_OUTER_BOUND('',#5098,.T.) ;
#3070=FACE_OUTER_BOUND('',#5099,.T.) ;
#3071=FACE_OUTER_BOUND('',#5100,.T.) ;
#3072=FACE_OUTER_BOUND('',#5101,.T.) ;
#3073=FACE_OUTER_BOUND('',#5102,.T.) ;
#3074=FACE_OUTER_BOUND('',#5103,.T.) ;
#3075=FACE_OUTER_BOUND('',#5104,.T.) ;
#3076=FACE_OUTER_BOUND('',#5105,.T.) ;
#3077=FACE_OUTER_BOUND('',#5106,.T.) ;
#3078=FACE_OUTER_BOUND('',#5107,.T.) ;
#3079=FACE_OUTER_BOUND('',#5108,.T.) ;
#3080=FACE_OUTER_BOUND('',#5109,.T.) ;
#3081=FACE_OUTER_BOUND('',#5110,.T.) ;
#3082=FACE_OUTER_BOUND('',#5111,.T.) ;
#3083=FACE_OUTER_BOUND('',#5112,.T.) ;
#3084=FACE_OUTER_BOUND('',#5113,.T.) ;
#3085=FACE_OUTER_BOUND('',#5114,.T.) ;
#3086=FACE_OUTER_BOUND('',#5115,.T.) ;
#3087=FACE_OUTER_BOUND('',#5116,.T.) ;
#3088=FACE_OUTER_BOUND('',#5117,.T.) ;
#3089=FACE_OUTER_BOUND('',#5118,.T.) ;
#3090=FACE_OUTER_BOUND('',#5119,.T.) ;
#3091=FACE_OUTER_BOUND('',#5120,.T.) ;
#3092=FACE_OUTER_BOUND('',#5121,.T.) ;
#3093=FACE_OUTER_BOUND('',#5122,.T.) ;
#3094=FACE_OUTER_BOUND('',#5123,.T.) ;
#3095=FACE_OUTER_BOUND('',#5124,.T.) ;
#3096=FACE_OUTER_BOUND('',#5125,.T.) ;
#3097=FACE_OUTER_BOUND('',#5126,.T.) ;
#3098=FACE_OUTER_BOUND('',#5127,.T.) ;
#3099=FACE_OUTER_BOUND('',#5128,.T.) ;
#3100=FACE_OUTER_BOUND('',#5129,.T.) ;
#3101=FACE_OUTER_BOUND('',#5130,.T.) ;
#3102=FACE_OUTER_BOUND('',#5131,.T.) ;
#3103=FACE_OUTER_BOUND('',#5132,.T.) ;
#3104=FACE_OUTER_BOUND('',#5133,.T.) ;
#3105=FACE_OUTER_BOUND('',#5134,.T.) ;
#3106=FACE_OUTER_BOUND('',#5135,.T.) ;
#3107=FACE_OUTER_BOUND('',#5136,.T.) ;
#3108=FACE_OUTER_BOUND('',#5137,.T.) ;
#3109=FACE_OUTER_BOUND('',#5138,.T.) ;
#3110=FACE_OUTER_BOUND('',#5139,.T.) ;
#3111=FACE_OUTER_BOUND('',#5140,.T.) ;
#3112=FACE_OUTER_BOUND('',#5141,.T.) ;
#3113=FACE_OUTER_BOUND('',#5142,.T.) ;
#3114=FACE_OUTER_BOUND('',#5143,.T.) ;
#3115=FACE_OUTER_BOUND('',#5144,.T.) ;
#3116=FACE_OUTER_BOUND('',#5145,.T.) ;
#3117=FACE_OUTER_BOUND('',#5146,.T.) ;
#3118=FACE_OUTER_BOUND('',#5147,.T.) ;
#3119=FACE_OUTER_BOUND('',#5148,.T.) ;
#3120=FACE_OUTER_BOUND('',#5149,.T.) ;
#3121=FACE_OUTER_BOUND('',#5150,.T.) ;
#3122=FACE_OUTER_BOUND('',#5151,.T.) ;
#3123=FACE_OUTER_BOUND('',#5152,.T.) ;
#3124=FACE_OUTER_BOUND('',#5153,.T.) ;
#3125=FACE_OUTER_BOUND('',#5154,.T.) ;
#3126=FACE_OUTER_BOUND('',#5155,.T.) ;
#3127=FACE_OUTER_BOUND('',#5156,.T.) ;
#3128=FACE_OUTER_BOUND('',#5157,.T.) ;
#3129=FACE_OUTER_BOUND('',#5158,.T.) ;
#3130=FACE_OUTER_BOUND('',#5159,.T.) ;
#3131=FACE_OUTER_BOUND('',#5160,.T.) ;
#3132=FACE_OUTER_BOUND('',#5161,.T.) ;
#3133=FACE_OUTER_BOUND('',#5162,.T.) ;
#3134=FACE_OUTER_BOUND('',#5163,.T.) ;
#3135=FACE_OUTER_BOUND('',#5164,.T.) ;
#3136=FACE_OUTER_BOUND('',#5165,.T.) ;
#3137=FACE_OUTER_BOUND('',#5166,.T.) ;
#3138=FACE_OUTER_BOUND('',#5167,.T.) ;
#3139=FACE_OUTER_BOUND('',#5168,.T.) ;
#3140=FACE_OUTER_BOUND('',#5169,.T.) ;
#3141=FACE_OUTER_BOUND('',#5170,.T.) ;
#3142=FACE_OUTER_BOUND('',#5171,.T.) ;
#3143=FACE_OUTER_BOUND('',#5172,.T.) ;
#3144=FACE_OUTER_BOUND('',#5173,.T.) ;
#3145=FACE_OUTER_BOUND('',#5174,.T.) ;
#3146=FACE_OUTER_BOUND('',#5175,.T.) ;
#3147=FACE_OUTER_BOUND('',#5176,.T.) ;
#3148=FACE_OUTER_BOUND('',#5177,.T.) ;
#3149=FACE_OUTER_BOUND('',#5178,.T.) ;
#3150=FACE_OUTER_BOUND('',#5179,.T.) ;
#3151=FACE_OUTER_BOUND('',#5180,.T.) ;
#3152=FACE_OUTER_BOUND('',#5181,.T.) ;
#3153=FACE_OUTER_BOUND('',#5182,.T.) ;
#3154=FACE_OUTER_BOUND('',#5183,.T.) ;
#3155=FACE_OUTER_BOUND('',#5184,.T.) ;
#3156=FACE_OUTER_BOUND('',#5185,.T.) ;
#3157=FACE_OUTER_BOUND('',#5186,.T.) ;
#3158=FACE_OUTER_BOUND('',#5187,.T.) ;
#3159=FACE_OUTER_BOUND('',#5188,.T.) ;
#3160=FACE_OUTER_BOUND('',#5189,.T.) ;
#3161=FACE_OUTER_BOUND('',#5190,.T.) ;
#3162=FACE_OUTER_BOUND('',#5191,.T.) ;
#3163=FACE_OUTER_BOUND('',#5192,.T.) ;
#3164=FACE_OUTER_BOUND('',#5193,.T.) ;
#3165=FACE_OUTER_BOUND('',#5197,.T.) ;
#3166=FACE_OUTER_BOUND('',#5198,.T.) ;
#3167=FACE_OUTER_BOUND('',#5199,.T.) ;
#3168=FACE_OUTER_BOUND('',#5200,.T.) ;
#3169=FACE_OUTER_BOUND('',#5201,.T.) ;
#3170=FACE_OUTER_BOUND('',#5202,.T.) ;
#3171=FACE_OUTER_BOUND('',#5203,.T.) ;
#3172=FACE_OUTER_BOUND('',#5204,.T.) ;
#3173=FACE_OUTER_BOUND('',#5205,.T.) ;
#3174=FACE_OUTER_BOUND('',#5206,.T.) ;
#3175=FACE_OUTER_BOUND('',#5207,.T.) ;
#3176=FACE_OUTER_BOUND('',#5208,.T.) ;
#3177=FACE_OUTER_BOUND('',#5209,.T.) ;
#3178=FACE_OUTER_BOUND('',#5210,.T.) ;
#3179=FACE_OUTER_BOUND('',#5211,.T.) ;
#3180=FACE_OUTER_BOUND('',#5212,.T.) ;
#3181=FACE_OUTER_BOUND('',#5213,.T.) ;
#3182=FACE_OUTER_BOUND('',#5214,.T.) ;
#3183=FACE_OUTER_BOUND('',#5215,.T.) ;
#3184=FACE_OUTER_BOUND('',#5216,.T.) ;
#3185=FACE_OUTER_BOUND('',#5218,.T.) ;
#3186=FACE_OUTER_BOUND('',#5219,.T.) ;
#3187=FACE_OUTER_BOUND('',#5220,.T.) ;
#3188=FACE_OUTER_BOUND('',#5221,.T.) ;
#3189=FACE_OUTER_BOUND('',#5222,.T.) ;
#3190=FACE_OUTER_BOUND('',#5223,.T.) ;
#3191=FACE_OUTER_BOUND('',#5224,.T.) ;
#3192=FACE_OUTER_BOUND('',#5225,.T.) ;
#3193=FACE_OUTER_BOUND('',#5226,.T.) ;
#3194=FACE_OUTER_BOUND('',#5227,.T.) ;
#3195=FACE_OUTER_BOUND('',#5228,.T.) ;
#3196=FACE_OUTER_BOUND('',#5229,.T.) ;
#3197=FACE_OUTER_BOUND('',#5230,.T.) ;
#3198=FACE_OUTER_BOUND('',#5231,.T.) ;
#3199=FACE_OUTER_BOUND('',#5232,.T.) ;
#3200=FACE_OUTER_BOUND('',#5233,.T.) ;
#3201=FACE_OUTER_BOUND('',#5234,.T.) ;
#3202=FACE_OUTER_BOUND('',#5235,.T.) ;
#3203=FACE_OUTER_BOUND('',#5236,.T.) ;
#3204=FACE_OUTER_BOUND('',#5237,.T.) ;
#3205=FACE_OUTER_BOUND('',#5238,.T.) ;
#3206=FACE_OUTER_BOUND('',#5239,.T.) ;
#3207=FACE_OUTER_BOUND('',#5240,.T.) ;
#3208=FACE_OUTER_BOUND('',#5241,.T.) ;
#3209=FACE_OUTER_BOUND('',#5242,.T.) ;
#3210=FACE_OUTER_BOUND('',#5243,.T.) ;
#3211=FACE_OUTER_BOUND('',#5244,.T.) ;
#3212=FACE_OUTER_BOUND('',#5245,.T.) ;
#3213=FACE_OUTER_BOUND('',#5246,.T.) ;
#3214=FACE_OUTER_BOUND('',#5247,.T.) ;
#3215=FACE_OUTER_BOUND('',#5248,.T.) ;
#3216=FACE_OUTER_BOUND('',#5249,.T.) ;
#3217=FACE_OUTER_BOUND('',#5250,.T.) ;
#3218=FACE_OUTER_BOUND('',#5251,.T.) ;
#3219=FACE_OUTER_BOUND('',#5252,.T.) ;
#3220=FACE_OUTER_BOUND('',#5253,.T.) ;
#3221=FACE_OUTER_BOUND('',#5254,.T.) ;
#3222=FACE_OUTER_BOUND('',#5255,.T.) ;
#3223=FACE_OUTER_BOUND('',#5256,.T.) ;
#3224=FACE_OUTER_BOUND('',#5257,.T.) ;
#3225=FACE_OUTER_BOUND('',#5258,.T.) ;
#3226=FACE_OUTER_BOUND('',#5259,.T.) ;
#3227=FACE_OUTER_BOUND('',#5260,.T.) ;
#3228=FACE_OUTER_BOUND('',#5261,.T.) ;
#3229=FACE_OUTER_BOUND('',#5262,.T.) ;
#3230=FACE_OUTER_BOUND('',#5263,.T.) ;
#3231=FACE_OUTER_BOUND('',#5264,.T.) ;
#3232=FACE_OUTER_BOUND('',#5265,.T.) ;
#3233=FACE_OUTER_BOUND('',#5266,.T.) ;
#3234=FACE_OUTER_BOUND('',#5267,.T.) ;
#3235=FACE_OUTER_BOUND('',#5268,.T.) ;
#3236=FACE_OUTER_BOUND('',#5269,.T.) ;
#3237=FACE_OUTER_BOUND('',#5270,.T.) ;
#3238=FACE_OUTER_BOUND('',#5271,.T.) ;
#3239=FACE_OUTER_BOUND('',#5272,.T.) ;
#3240=FACE_OUTER_BOUND('',#5273,.T.) ;
#3241=FACE_OUTER_BOUND('',#5274,.T.) ;
#3242=FACE_OUTER_BOUND('',#5275,.T.) ;
#3243=FACE_OUTER_BOUND('',#5276,.T.) ;
#3244=FACE_OUTER_BOUND('',#5277,.T.) ;
#3245=FACE_OUTER_BOUND('',#5278,.T.) ;
#3246=FACE_OUTER_BOUND('',#5279,.T.) ;
#3247=FACE_OUTER_BOUND('',#5280,.T.) ;
#3248=FACE_OUTER_BOUND('',#5281,.T.) ;
#3249=FACE_OUTER_BOUND('',#5282,.T.) ;
#3250=FACE_OUTER_BOUND('',#5283,.T.) ;
#3251=FACE_OUTER_BOUND('',#5284,.T.) ;
#3252=FACE_OUTER_BOUND('',#5285,.T.) ;
#3253=FACE_OUTER_BOUND('',#5286,.T.) ;
#3254=FACE_OUTER_BOUND('',#5287,.T.) ;
#3255=FACE_OUTER_BOUND('',#5288,.T.) ;
#3256=FACE_OUTER_BOUND('',#5289,.T.) ;
#3257=FACE_OUTER_BOUND('',#5290,.T.) ;
#3258=FACE_OUTER_BOUND('',#5291,.T.) ;
#3259=FACE_OUTER_BOUND('',#5292,.T.) ;
#3260=FACE_OUTER_BOUND('',#5293,.T.) ;
#3261=FACE_OUTER_BOUND('',#5294,.T.) ;
#3262=FACE_OUTER_BOUND('',#5295,.T.) ;
#3263=FACE_OUTER_BOUND('',#5296,.T.) ;
#3264=FACE_OUTER_BOUND('',#5297,.T.) ;
#3265=FACE_OUTER_BOUND('',#5298,.T.) ;
#3266=FACE_OUTER_BOUND('',#5299,.T.) ;
#3267=FACE_OUTER_BOUND('',#5300,.T.) ;
#3268=FACE_OUTER_BOUND('',#5301,.T.) ;
#3269=FACE_OUTER_BOUND('',#5302,.T.) ;
#3270=FACE_OUTER_BOUND('',#5303,.T.) ;
#3271=FACE_OUTER_BOUND('',#5304,.T.) ;
#3272=FACE_OUTER_BOUND('',#5305,.T.) ;
#3273=FACE_OUTER_BOUND('',#5306,.T.) ;
#3274=FACE_OUTER_BOUND('',#5307,.T.) ;
#3275=FACE_OUTER_BOUND('',#5308,.T.) ;
#3276=FACE_OUTER_BOUND('',#5309,.T.) ;
#3277=FACE_OUTER_BOUND('',#5310,.T.) ;
#3278=FACE_OUTER_BOUND('',#5311,.T.) ;
#3279=FACE_OUTER_BOUND('',#5312,.T.) ;
#3280=FACE_OUTER_BOUND('',#5313,.T.) ;
#3281=FACE_OUTER_BOUND('',#5314,.T.) ;
#3282=FACE_OUTER_BOUND('',#5315,.T.) ;
#3283=FACE_OUTER_BOUND('',#5316,.T.) ;
#3284=FACE_OUTER_BOUND('',#5317,.T.) ;
#3285=FACE_OUTER_BOUND('',#5318,.T.) ;
#3286=FACE_OUTER_BOUND('',#5319,.T.) ;
#3287=FACE_OUTER_BOUND('',#5320,.T.) ;
#3288=FACE_OUTER_BOUND('',#5321,.T.) ;
#3289=FACE_OUTER_BOUND('',#5322,.T.) ;
#3290=FACE_OUTER_BOUND('',#5323,.T.) ;
#3291=FACE_OUTER_BOUND('',#5324,.T.) ;
#3292=FACE_OUTER_BOUND('',#5325,.T.) ;
#3293=FACE_OUTER_BOUND('',#5326,.T.) ;
#3294=FACE_OUTER_BOUND('',#5327,.T.) ;
#3295=FACE_OUTER_BOUND('',#5328,.T.) ;
#3296=FACE_OUTER_BOUND('',#5329,.T.) ;
#3297=FACE_OUTER_BOUND('',#5330,.T.) ;
#3298=FACE_OUTER_BOUND('',#5331,.T.) ;
#3299=FACE_OUTER_BOUND('',#5332,.T.) ;
#3300=FACE_OUTER_BOUND('',#5333,.T.) ;
#3301=FACE_OUTER_BOUND('',#5334,.T.) ;
#3302=FACE_OUTER_BOUND('',#5335,.T.) ;
#3303=FACE_OUTER_BOUND('',#5336,.T.) ;
#3304=FACE_OUTER_BOUND('',#5337,.T.) ;
#3305=FACE_OUTER_BOUND('',#5338,.T.) ;
#3306=FACE_OUTER_BOUND('',#5339,.T.) ;
#3307=FACE_OUTER_BOUND('',#5340,.T.) ;
#3308=FACE_OUTER_BOUND('',#5341,.T.) ;
#3309=FACE_OUTER_BOUND('',#5342,.T.) ;
#3310=FACE_OUTER_BOUND('',#5343,.T.) ;
#3311=FACE_OUTER_BOUND('',#5344,.T.) ;
#3312=FACE_OUTER_BOUND('',#5345,.T.) ;
#3313=FACE_OUTER_BOUND('',#5346,.T.) ;
#3314=FACE_OUTER_BOUND('',#5347,.T.) ;
#3315=FACE_OUTER_BOUND('',#5348,.T.) ;
#3316=FACE_OUTER_BOUND('',#5349,.T.) ;
#3317=FACE_OUTER_BOUND('',#5350,.T.) ;
#3318=FACE_OUTER_BOUND('',#5351,.T.) ;
#3319=FACE_OUTER_BOUND('',#5352,.T.) ;
#3320=FACE_OUTER_BOUND('',#5353,.T.) ;
#3321=FACE_OUTER_BOUND('',#5354,.T.) ;
#3322=FACE_OUTER_BOUND('',#5355,.T.) ;
#3323=FACE_OUTER_BOUND('',#5356,.T.) ;
#3324=FACE_OUTER_BOUND('',#5357,.T.) ;
#3325=FACE_OUTER_BOUND('',#5358,.T.) ;
#3326=FACE_OUTER_BOUND('',#5359,.T.) ;
#3327=FACE_OUTER_BOUND('',#5360,.T.) ;
#3328=FACE_OUTER_BOUND('',#5361,.T.) ;
#3329=FACE_OUTER_BOUND('',#5362,.T.) ;
#3330=FACE_OUTER_BOUND('',#5363,.T.) ;
#3331=FACE_OUTER_BOUND('',#5364,.T.) ;
#3332=FACE_OUTER_BOUND('',#5365,.T.) ;
#3333=FACE_OUTER_BOUND('',#5366,.T.) ;
#3334=FACE_OUTER_BOUND('',#5367,.T.) ;
#3335=FACE_OUTER_BOUND('',#5368,.T.) ;
#3336=FACE_OUTER_BOUND('',#5369,.T.) ;
#3337=FACE_OUTER_BOUND('',#5370,.T.) ;
#3338=FACE_OUTER_BOUND('',#5371,.T.) ;
#3339=FACE_OUTER_BOUND('',#5372,.T.) ;
#3340=FACE_OUTER_BOUND('',#5373,.T.) ;
#3341=FACE_OUTER_BOUND('',#5374,.T.) ;
#3342=FACE_OUTER_BOUND('',#5375,.T.) ;
#3343=FACE_OUTER_BOUND('',#5376,.T.) ;
#3344=FACE_OUTER_BOUND('',#5377,.T.) ;
#3345=FACE_OUTER_BOUND('',#5378,.T.) ;
#3346=FACE_OUTER_BOUND('',#5379,.T.) ;
#3347=FACE_OUTER_BOUND('',#5380,.T.) ;
#3348=FACE_OUTER_BOUND('',#5381,.T.) ;
#3349=FACE_OUTER_BOUND('',#5382,.T.) ;
#3350=FACE_OUTER_BOUND('',#5383,.T.) ;
#3351=FACE_OUTER_BOUND('',#5384,.T.) ;
#3352=FACE_OUTER_BOUND('',#5385,.T.) ;
#3353=FACE_OUTER_BOUND('',#5386,.T.) ;
#3354=FACE_OUTER_BOUND('',#5387,.T.) ;
#3355=FACE_OUTER_BOUND('',#5388,.T.) ;
#3356=FACE_OUTER_BOUND('',#5389,.T.) ;
#3357=FACE_OUTER_BOUND('',#5390,.T.) ;
#3358=FACE_OUTER_BOUND('',#5391,.T.) ;
#3359=FACE_OUTER_BOUND('',#5392,.T.) ;
#3360=FACE_OUTER_BOUND('',#5393,.T.) ;
#3361=FACE_OUTER_BOUND('',#5394,.T.) ;
#3362=FACE_OUTER_BOUND('',#5395,.T.) ;
#3363=FACE_OUTER_BOUND('',#5396,.T.) ;
#3364=FACE_OUTER_BOUND('',#5397,.T.) ;
#3365=FACE_OUTER_BOUND('',#5398,.T.) ;
#3366=FACE_OUTER_BOUND('',#5399,.T.) ;
#3367=FACE_OUTER_BOUND('',#5400,.T.) ;
#3368=FACE_OUTER_BOUND('',#5401,.T.) ;
#3369=FACE_OUTER_BOUND('',#5402,.T.) ;
#3370=FACE_OUTER_BOUND('',#5403,.T.) ;
#3371=FACE_OUTER_BOUND('',#5404,.T.) ;
#3372=FACE_OUTER_BOUND('',#5405,.T.) ;
#3373=FACE_OUTER_BOUND('',#5406,.T.) ;
#3374=FACE_OUTER_BOUND('',#5407,.T.) ;
#3375=FACE_OUTER_BOUND('',#5408,.T.) ;
#3376=FACE_OUTER_BOUND('',#5409,.T.) ;
#3377=FACE_OUTER_BOUND('',#5410,.T.) ;
#3378=FACE_OUTER_BOUND('',#5411,.T.) ;
#3379=FACE_OUTER_BOUND('',#5412,.T.) ;
#3380=FACE_OUTER_BOUND('',#5413,.T.) ;
#3381=FACE_OUTER_BOUND('',#5414,.T.) ;
#3382=FACE_OUTER_BOUND('',#5415,.T.) ;
#3383=FACE_OUTER_BOUND('',#5416,.T.) ;
#3384=FACE_OUTER_BOUND('',#5417,.T.) ;
#3385=FACE_OUTER_BOUND('',#5418,.T.) ;
#3386=FACE_OUTER_BOUND('',#5419,.T.) ;
#3387=FACE_OUTER_BOUND('',#5420,.T.) ;
#3388=FACE_OUTER_BOUND('',#5421,.T.) ;
#3389=FACE_OUTER_BOUND('',#5422,.T.) ;
#3390=FACE_OUTER_BOUND('',#5423,.T.) ;
#3391=FACE_OUTER_BOUND('',#5424,.T.) ;
#3392=FACE_OUTER_BOUND('',#5425,.T.) ;
#3393=FACE_OUTER_BOUND('',#5426,.T.) ;
#3394=FACE_OUTER_BOUND('',#5427,.T.) ;
#3395=FACE_OUTER_BOUND('',#5428,.T.) ;
#3396=FACE_OUTER_BOUND('',#5429,.T.) ;
#3397=FACE_OUTER_BOUND('',#5430,.T.) ;
#3398=FACE_OUTER_BOUND('',#5431,.T.) ;
#3399=FACE_OUTER_BOUND('',#5432,.T.) ;
#3400=FACE_OUTER_BOUND('',#5433,.T.) ;
#3401=FACE_OUTER_BOUND('',#5434,.T.) ;
#3402=FACE_OUTER_BOUND('',#5435,.T.) ;
#3403=FACE_OUTER_BOUND('',#5436,.T.) ;
#3404=FACE_OUTER_BOUND('',#5437,.T.) ;
#3405=FACE_OUTER_BOUND('',#5438,.T.) ;
#3406=FACE_OUTER_BOUND('',#5439,.T.) ;
#3407=FACE_OUTER_BOUND('',#5440,.T.) ;
#3408=FACE_OUTER_BOUND('',#5441,.T.) ;
#3409=FACE_OUTER_BOUND('',#5442,.T.) ;
#3410=FACE_OUTER_BOUND('',#5443,.T.) ;
#3411=FACE_OUTER_BOUND('',#5444,.T.) ;
#3412=FACE_OUTER_BOUND('',#5445,.T.) ;
#3413=FACE_OUTER_BOUND('',#5446,.T.) ;
#3414=FACE_OUTER_BOUND('',#5447,.T.) ;
#3415=FACE_OUTER_BOUND('',#5448,.T.) ;
#3416=FACE_OUTER_BOUND('',#5449,.T.) ;
#3417=FACE_OUTER_BOUND('',#5450,.T.) ;
#3418=FACE_OUTER_BOUND('',#5451,.T.) ;
#3419=FACE_OUTER_BOUND('',#5452,.T.) ;
#3420=FACE_OUTER_BOUND('',#5453,.T.) ;
#3421=FACE_OUTER_BOUND('',#5454,.T.) ;
#3422=FACE_OUTER_BOUND('',#5455,.T.) ;
#3423=FACE_OUTER_BOUND('',#5456,.T.) ;
#3424=FACE_OUTER_BOUND('',#5457,.T.) ;
#3425=FACE_OUTER_BOUND('',#5458,.T.) ;
#3426=FACE_OUTER_BOUND('',#5459,.T.) ;
#3427=FACE_OUTER_BOUND('',#5460,.T.) ;
#3428=FACE_OUTER_BOUND('',#5461,.T.) ;
#3429=FACE_OUTER_BOUND('',#5462,.T.) ;
#3430=FACE_OUTER_BOUND('',#5463,.T.) ;
#3431=FACE_OUTER_BOUND('',#5464,.T.) ;
#3432=FACE_OUTER_BOUND('',#5465,.T.) ;
#3433=FACE_OUTER_BOUND('',#5466,.T.) ;
#3434=FACE_OUTER_BOUND('',#5467,.T.) ;
#3435=FACE_OUTER_BOUND('',#5468,.T.) ;
#3436=FACE_OUTER_BOUND('',#5469,.T.) ;
#3437=FACE_OUTER_BOUND('',#5470,.T.) ;
#3438=FACE_OUTER_BOUND('',#5471,.T.) ;
#3439=FACE_OUTER_BOUND('',#5472,.T.) ;
#3440=FACE_OUTER_BOUND('',#5473,.T.) ;
#3441=FACE_OUTER_BOUND('',#5474,.T.) ;
#3442=FACE_OUTER_BOUND('',#5475,.T.) ;
#3443=FACE_OUTER_BOUND('',#5476,.T.) ;
#3444=FACE_OUTER_BOUND('',#5477,.T.) ;
#3445=FACE_OUTER_BOUND('',#5478,.T.) ;
#3446=FACE_OUTER_BOUND('',#5479,.T.) ;
#3447=FACE_OUTER_BOUND('',#5480,.T.) ;
#3448=FACE_OUTER_BOUND('',#5481,.T.) ;
#3449=FACE_OUTER_BOUND('',#5482,.T.) ;
#3450=FACE_OUTER_BOUND('',#5483,.T.) ;
#3451=FACE_OUTER_BOUND('',#5484,.T.) ;
#3452=FACE_OUTER_BOUND('',#5485,.T.) ;
#3453=FACE_OUTER_BOUND('',#5486,.T.) ;
#3454=FACE_OUTER_BOUND('',#5487,.T.) ;
#3455=FACE_OUTER_BOUND('',#5488,.T.) ;
#3456=FACE_OUTER_BOUND('',#5489,.T.) ;
#3457=FACE_OUTER_BOUND('',#5490,.T.) ;
#3458=FACE_OUTER_BOUND('',#5491,.T.) ;
#3459=FACE_OUTER_BOUND('',#5492,.T.) ;
#3460=FACE_OUTER_BOUND('',#5493,.T.) ;
#3461=FACE_OUTER_BOUND('',#5494,.T.) ;
#3462=FACE_OUTER_BOUND('',#5495,.T.) ;
#3463=FACE_OUTER_BOUND('',#5496,.T.) ;
#3464=FACE_OUTER_BOUND('',#5497,.T.) ;
#3465=FACE_OUTER_BOUND('',#5498,.T.) ;
#3466=FACE_OUTER_BOUND('',#5499,.T.) ;
#3467=FACE_OUTER_BOUND('',#5500,.T.) ;
#3468=FACE_OUTER_BOUND('',#5501,.T.) ;
#3469=FACE_OUTER_BOUND('',#5502,.T.) ;
#3470=FACE_OUTER_BOUND('',#5503,.T.) ;
#3471=FACE_OUTER_BOUND('',#5504,.T.) ;
#3472=FACE_OUTER_BOUND('',#5505,.T.) ;
#3473=FACE_OUTER_BOUND('',#5506,.T.) ;
#3474=FACE_OUTER_BOUND('',#5507,.T.) ;
#3475=FACE_OUTER_BOUND('',#5508,.T.) ;
#3476=FACE_OUTER_BOUND('',#5509,.T.) ;
#3477=FACE_OUTER_BOUND('',#5510,.T.) ;
#3478=FACE_OUTER_BOUND('',#5511,.T.) ;
#3479=FACE_OUTER_BOUND('',#5512,.T.) ;
#3480=FACE_OUTER_BOUND('',#5513,.T.) ;
#3481=FACE_OUTER_BOUND('',#5514,.T.) ;
#3482=FACE_OUTER_BOUND('',#5515,.T.) ;
#3483=FACE_OUTER_BOUND('',#5516,.T.) ;
#3484=FACE_OUTER_BOUND('',#5517,.T.) ;
#3485=FACE_OUTER_BOUND('',#5518,.T.) ;
#3486=FACE_OUTER_BOUND('',#5519,.T.) ;
#3487=FACE_OUTER_BOUND('',#5520,.T.) ;
#3488=FACE_OUTER_BOUND('',#5521,.T.) ;
#3489=FACE_OUTER_BOUND('',#5522,.T.) ;
#3490=FACE_OUTER_BOUND('',#5523,.T.) ;
#3491=FACE_OUTER_BOUND('',#5524,.T.) ;
#3492=FACE_OUTER_BOUND('',#5525,.T.) ;
#3493=FACE_OUTER_BOUND('',#5526,.T.) ;
#3494=FACE_OUTER_BOUND('',#5527,.T.) ;
#3495=FACE_OUTER_BOUND('',#5528,.T.) ;
#3496=FACE_OUTER_BOUND('',#5529,.T.) ;
#3497=FACE_OUTER_BOUND('',#5530,.T.) ;
#3498=FACE_OUTER_BOUND('',#5531,.T.) ;
#3499=FACE_OUTER_BOUND('',#5532,.T.) ;
#3500=FACE_OUTER_BOUND('',#5533,.T.) ;
#3501=FACE_OUTER_BOUND('',#5534,.T.) ;
#3502=FACE_OUTER_BOUND('',#5535,.T.) ;
#3503=FACE_OUTER_BOUND('',#5536,.T.) ;
#3504=FACE_OUTER_BOUND('',#5537,.T.) ;
#3505=FACE_OUTER_BOUND('',#5538,.T.) ;
#3506=FACE_OUTER_BOUND('',#5539,.T.) ;
#3507=FACE_OUTER_BOUND('',#5540,.T.) ;
#3508=FACE_OUTER_BOUND('',#5541,.T.) ;
#3509=FACE_OUTER_BOUND('',#5542,.T.) ;
#3510=FACE_OUTER_BOUND('',#5543,.T.) ;
#3511=FACE_OUTER_BOUND('',#5544,.T.) ;
#3512=FACE_OUTER_BOUND('',#5545,.T.) ;
#3513=FACE_OUTER_BOUND('',#5546,.T.) ;
#3514=FACE_OUTER_BOUND('',#5547,.T.) ;
#3515=FACE_OUTER_BOUND('',#5548,.T.) ;
#3516=FACE_OUTER_BOUND('',#5549,.T.) ;
#3517=FACE_OUTER_BOUND('',#5550,.T.) ;
#3518=FACE_OUTER_BOUND('',#5551,.T.) ;
#3519=FACE_OUTER_BOUND('',#5552,.T.) ;
#3520=FACE_OUTER_BOUND('',#5553,.T.) ;
#3521=FACE_OUTER_BOUND('',#5554,.T.) ;
#3522=FACE_OUTER_BOUND('',#5555,.T.) ;
#3523=FACE_OUTER_BOUND('',#5556,.T.) ;
#3524=FACE_OUTER_BOUND('',#5557,.T.) ;
#3525=FACE_OUTER_BOUND('',#5558,.T.) ;
#3526=FACE_OUTER_BOUND('',#5559,.T.) ;
#3527=FACE_OUTER_BOUND('',#5560,.T.) ;
#3528=FACE_OUTER_BOUND('',#5561,.T.) ;
#3529=FACE_OUTER_BOUND('',#5562,.T.) ;
#3530=FACE_OUTER_BOUND('',#5563,.T.) ;
#3531=FACE_OUTER_BOUND('',#5564,.T.) ;
#3532=FACE_OUTER_BOUND('',#5568,.T.) ;
#3533=FACE_OUTER_BOUND('',#5569,.T.) ;
#3534=FACE_OUTER_BOUND('',#5570,.T.) ;
#3535=FACE_OUTER_BOUND('',#5571,.T.) ;
#3536=FACE_OUTER_BOUND('',#5572,.T.) ;
#3537=FACE_OUTER_BOUND('',#5573,.T.) ;
#3538=FACE_OUTER_BOUND('',#5577,.T.) ;
#3539=FACE_OUTER_BOUND('',#5578,.T.) ;
#3540=FACE_OUTER_BOUND('',#5579,.T.) ;
#3541=FACE_OUTER_BOUND('',#5580,.T.) ;
#3542=FACE_OUTER_BOUND('',#5581,.T.) ;
#3543=FACE_OUTER_BOUND('',#5582,.T.) ;
#3544=FACE_OUTER_BOUND('',#5586,.T.) ;
#3545=FACE_OUTER_BOUND('',#5587,.T.) ;
#3546=FACE_OUTER_BOUND('',#5588,.T.) ;
#3547=FACE_OUTER_BOUND('',#5589,.T.) ;
#3548=FACE_OUTER_BOUND('',#5590,.T.) ;
#3549=FACE_OUTER_BOUND('',#5591,.T.) ;
#3550=FACE_OUTER_BOUND('',#5595,.T.) ;
#3551=FACE_OUTER_BOUND('',#5596,.T.) ;
#3552=FACE_OUTER_BOUND('',#5597,.T.) ;
#3553=FACE_OUTER_BOUND('',#5598,.T.) ;
#3554=FACE_OUTER_BOUND('',#5599,.T.) ;
#3555=FACE_OUTER_BOUND('',#5600,.T.) ;
#3556=FACE_OUTER_BOUND('',#5604,.T.) ;
#3557=FACE_OUTER_BOUND('',#5605,.T.) ;
#3558=FACE_OUTER_BOUND('',#5606,.T.) ;
#3559=FACE_OUTER_BOUND('',#5607,.T.) ;
#3560=FACE_OUTER_BOUND('',#5608,.T.) ;
#3561=FACE_OUTER_BOUND('',#5609,.T.) ;
#3562=FACE_OUTER_BOUND('',#5613,.T.) ;
#3563=FACE_OUTER_BOUND('',#5614,.T.) ;
#3564=FACE_OUTER_BOUND('',#5615,.T.) ;
#3565=FACE_OUTER_BOUND('',#5616,.T.) ;
#3566=FACE_OUTER_BOUND('',#5617,.T.) ;
#3567=FACE_OUTER_BOUND('',#5618,.T.) ;
#3568=FACE_OUTER_BOUND('',#5622,.T.) ;
#3569=FACE_OUTER_BOUND('',#5623,.T.) ;
#3570=FACE_OUTER_BOUND('',#5624,.T.) ;
#3571=FACE_OUTER_BOUND('',#5625,.T.) ;
#3572=FACE_OUTER_BOUND('',#5626,.T.) ;
#3573=FACE_OUTER_BOUND('',#5627,.T.) ;
#3574=FACE_OUTER_BOUND('',#5631,.T.) ;
#3575=FACE_OUTER_BOUND('',#5632,.T.) ;
#3576=FACE_OUTER_BOUND('',#5633,.T.) ;
#3577=FACE_OUTER_BOUND('',#5634,.T.) ;
#3578=FACE_OUTER_BOUND('',#5635,.T.) ;
#3579=FACE_OUTER_BOUND('',#5636,.T.) ;
#3580=FACE_OUTER_BOUND('',#5637,.T.) ;
#3581=FACE_OUTER_BOUND('',#5638,.T.) ;
#3582=FACE_OUTER_BOUND('',#5639,.T.) ;
#3583=FACE_OUTER_BOUND('',#5640,.T.) ;
#3584=FACE_OUTER_BOUND('',#5641,.T.) ;
#3585=FACE_OUTER_BOUND('',#5642,.T.) ;
#3586=FACE_OUTER_BOUND('',#5643,.T.) ;
#3587=FACE_OUTER_BOUND('',#5644,.T.) ;
#3588=FACE_OUTER_BOUND('',#5645,.T.) ;
#3589=FACE_OUTER_BOUND('',#5646,.T.) ;
#3590=FACE_OUTER_BOUND('',#5647,.T.) ;
#3591=FACE_OUTER_BOUND('',#5648,.T.) ;
#3592=FACE_OUTER_BOUND('',#5649,.T.) ;
#3593=FACE_OUTER_BOUND('',#5650,.T.) ;
#3594=FACE_OUTER_BOUND('',#5651,.T.) ;
#3595=FACE_OUTER_BOUND('',#5652,.T.) ;
#3596=FACE_OUTER_BOUND('',#5653,.T.) ;
#3597=FACE_OUTER_BOUND('',#5654,.T.) ;
#3598=FACE_OUTER_BOUND('',#5655,.T.) ;
#3599=FACE_OUTER_BOUND('',#5656,.T.) ;
#3600=FACE_OUTER_BOUND('',#5657,.T.) ;
#3601=FACE_OUTER_BOUND('',#5658,.T.) ;
#3602=FACE_OUTER_BOUND('',#5659,.T.) ;
#3603=FACE_OUTER_BOUND('',#5660,.T.) ;
#3604=FACE_OUTER_BOUND('',#5661,.T.) ;
#3605=FACE_OUTER_BOUND('',#5662,.T.) ;
#3606=FACE_OUTER_BOUND('',#5663,.T.) ;
#3607=FACE_OUTER_BOUND('',#5664,.T.) ;
#3608=FACE_OUTER_BOUND('',#5665,.T.) ;
#3609=FACE_OUTER_BOUND('',#5666,.T.) ;
#3610=FACE_OUTER_BOUND('',#5667,.T.) ;
#3611=FACE_OUTER_BOUND('',#5668,.T.) ;
#3612=FACE_OUTER_BOUND('',#5669,.T.) ;
#3613=FACE_OUTER_BOUND('',#5670,.T.) ;
#3614=FACE_OUTER_BOUND('',#5671,.T.) ;
#3615=FACE_OUTER_BOUND('',#5672,.T.) ;
#3616=FACE_OUTER_BOUND('',#5673,.T.) ;
#3617=FACE_OUTER_BOUND('',#5674,.T.) ;
#3618=FACE_OUTER_BOUND('',#5675,.T.) ;
#3619=FACE_OUTER_BOUND('',#5676,.T.) ;
#3620=FACE_OUTER_BOUND('',#5677,.T.) ;
#3621=FACE_OUTER_BOUND('',#5678,.T.) ;
#3622=FACE_OUTER_BOUND('',#5679,.T.) ;
#3623=FACE_OUTER_BOUND('',#5680,.T.) ;
#4783=EDGE_LOOP('',(#23464,#23465,#23466,#23467)) ;
#4784=EDGE_LOOP('',(#23468,#23469,#23470,#23471)) ;
#4785=EDGE_LOOP('',(#23472,#23473,#23474,#23475)) ;
#4786=EDGE_LOOP('',(#23476,#23477,#23478,#23479)) ;
#4787=EDGE_LOOP('',(#23480,#23481,#23482,#23483)) ;
#4788=EDGE_LOOP('',(#23484,#23485,#23486,#23487)) ;
#4789=EDGE_LOOP('',(#23488,#23489,#23490,#23491)) ;
#4790=EDGE_LOOP('',(#23492,#23493,#23494,#23495)) ;
#4791=EDGE_LOOP('',(#23496,#23497,#23498,#23499)) ;
#4792=EDGE_LOOP('',(#23500,#23501,#23502,#23503)) ;
#4793=EDGE_LOOP('',(#23504,#23505,#23506,#23507)) ;
#4794=EDGE_LOOP('',(#23508,#23509,#23510,#23511)) ;
#4795=EDGE_LOOP('',(#23512,#23513,#23514,#23515)) ;
#4796=EDGE_LOOP('',(#23516,#23517,#23518,#23519)) ;
#4797=EDGE_LOOP('',(#23520,#23521,#23522,#23523)) ;
#4798=EDGE_LOOP('',(#23524,#23525,#23526,#23527)) ;
#4799=EDGE_LOOP('',(#23528,#23529,#23530,#23531)) ;
#4800=EDGE_LOOP('',(#23532,#23533,#23534,#23535)) ;
#4801=EDGE_LOOP('',(#23536,#23537,#23538,#23539)) ;
#4802=EDGE_LOOP('',(#23540,#23541,#23542,#23543)) ;
#4803=EDGE_LOOP('',(#23544,#23545,#23546,#23547)) ;
#4804=EDGE_LOOP('',(#23548,#23549,#23550,#23551)) ;
#4805=EDGE_LOOP('',(#23552,#23553,#23554,#23555)) ;
#4806=EDGE_LOOP('',(#23556,#23557,#23558,#23559)) ;
#4807=EDGE_LOOP('',(#23560,#23561,#23562,#23563)) ;
#4808=EDGE_LOOP('',(#23564,#23565,#23566,#23567)) ;
#4809=EDGE_LOOP('',(#23568,#23569,#23570,#23571)) ;
#4810=EDGE_LOOP('',(#23572,#23573,#23574,#23575)) ;
#4811=EDGE_LOOP('',(#23576,#23577,#23578,#23579)) ;
#4812=EDGE_LOOP('',(#23580,#23581,#23582,#23583)) ;
#4813=EDGE_LOOP('',(#23584,#23585,#23586,#23587)) ;
#4814=EDGE_LOOP('',(#23588,#23589,#23590,#23591)) ;
#4815=EDGE_LOOP('',(#23592,#23593,#23594,#23595)) ;
#4816=EDGE_LOOP('',(#23596,#23597,#23598,#23599)) ;
#4817=EDGE_LOOP('',(#23600,#23601,#23602,#23603)) ;
#4818=EDGE_LOOP('',(#23604,#23605,#23606,#23607)) ;
#4819=EDGE_LOOP('',(#23608,#23609,#23610,#23611,#23612,#23613,#23614,#23615,
#23616,#23617,#23618,#23619,#23620,#23621,#23622,#23623,#23624,#23625,#23626,
#23627,#23628,#23629,#23630,#23631,#23632,#23633,#23634,#23635,#23636,#23637,
#23638,#23639,#23640,#23641,#23642,#23643,#23644,#23645,#23646,#23647,#23648,
#23649,#23650,#23651,#23652,#23653,#23654,#23655,#23656,#23657,#23658,#23659,
#23660,#23661,#23662,#23663,#23664,#23665,#23666,#23667,#23668,#23669,#23670,
#23671,#23672,#23673,#23674,#23675,#23676,#23677,#23678,#23679,#23680,#23681,
#23682,#23683)) ;
#4820=EDGE_LOOP('',(#23684,#23685,#23686,#23687)) ;
#4821=EDGE_LOOP('',(#23688,#23689,#23690,#23691)) ;
#4822=EDGE_LOOP('',(#23692,#23693,#23694,#23695)) ;
#4823=EDGE_LOOP('',(#23696,#23697,#23698,#23699,#23700,#23701,#23702,#23703)) ;
#4824=EDGE_LOOP('',(#23704)) ;
#4825=EDGE_LOOP('',(#23705,#23706,#23707,#23708)) ;
#4826=EDGE_LOOP('',(#23709,#23710,#23711,#23712)) ;
#4827=EDGE_LOOP('',(#23713,#23714,#23715,#23716)) ;
#4828=EDGE_LOOP('',(#23717,#23718,#23719,#23720,#23721,#23722,#23723,#23724)) ;
#4829=EDGE_LOOP('',(#23725)) ;
#4830=EDGE_LOOP('',(#23726,#23727,#23728,#23729)) ;
#4831=EDGE_LOOP('',(#23730,#23731,#23732,#23733)) ;
#4832=EDGE_LOOP('',(#23734,#23735,#23736,#23737)) ;
#4833=EDGE_LOOP('',(#23738,#23739,#23740,#23741,#23742,#23743,#23744,#23745)) ;
#4834=EDGE_LOOP('',(#23746)) ;
#4835=EDGE_LOOP('',(#23747,#23748,#23749,#23750)) ;
#4836=EDGE_LOOP('',(#23751,#23752,#23753,#23754)) ;
#4837=EDGE_LOOP('',(#23755,#23756,#23757,#23758)) ;
#4838=EDGE_LOOP('',(#23759,#23760,#23761,#23762,#23763,#23764,#23765,#23766)) ;
#4839=EDGE_LOOP('',(#23767)) ;
#4840=EDGE_LOOP('',(#23768,#23769,#23770,#23771)) ;
#4841=EDGE_LOOP('',(#23772,#23773,#23774,#23775)) ;
#4842=EDGE_LOOP('',(#23776,#23777,#23778,#23779)) ;
#4843=EDGE_LOOP('',(#23780,#23781,#23782,#23783,#23784,#23785,#23786,#23787)) ;
#4844=EDGE_LOOP('',(#23788)) ;
#4845=EDGE_LOOP('',(#23789,#23790,#23791,#23792)) ;
#4846=EDGE_LOOP('',(#23793,#23794,#23795,#23796)) ;
#4847=EDGE_LOOP('',(#23797,#23798,#23799,#23800)) ;
#4848=EDGE_LOOP('',(#23801,#23802,#23803,#23804,#23805,#23806,#23807,#23808)) ;
#4849=EDGE_LOOP('',(#23809)) ;
#4850=EDGE_LOOP('',(#23810,#23811,#23812,#23813)) ;
#4851=EDGE_LOOP('',(#23814,#23815,#23816,#23817)) ;
#4852=EDGE_LOOP('',(#23818,#23819,#23820,#23821)) ;
#4853=EDGE_LOOP('',(#23822,#23823,#23824,#23825,#23826,#23827,#23828,#23829)) ;
#4854=EDGE_LOOP('',(#23830)) ;
#4855=EDGE_LOOP('',(#23831,#23832,#23833,#23834)) ;
#4856=EDGE_LOOP('',(#23835,#23836,#23837,#23838)) ;
#4857=EDGE_LOOP('',(#23839,#23840,#23841,#23842)) ;
#4858=EDGE_LOOP('',(#23843,#23844,#23845,#23846,#23847,#23848,#23849,#23850)) ;
#4859=EDGE_LOOP('',(#23851)) ;
#4860=EDGE_LOOP('',(#23852,#23853,#23854,#23855)) ;
#4861=EDGE_LOOP('',(#23856,#23857,#23858,#23859)) ;
#4862=EDGE_LOOP('',(#23860,#23861,#23862,#23863,#23864,#23865,#23866,#23867)) ;
#4863=EDGE_LOOP('',(#23868)) ;
#4864=EDGE_LOOP('',(#23869,#23870,#23871,#23872)) ;
#4865=EDGE_LOOP('',(#23873)) ;
#4866=EDGE_LOOP('',(#23874)) ;
#4867=EDGE_LOOP('',(#23875)) ;
#4868=EDGE_LOOP('',(#23876)) ;
#4869=EDGE_LOOP('',(#23877)) ;
#4870=EDGE_LOOP('',(#23878)) ;
#4871=EDGE_LOOP('',(#23879)) ;
#4872=EDGE_LOOP('',(#23880)) ;
#4873=EDGE_LOOP('',(#23881)) ;
#4874=EDGE_LOOP('',(#23882)) ;
#4875=EDGE_LOOP('',(#23883)) ;
#4876=EDGE_LOOP('',(#23884)) ;
#4877=EDGE_LOOP('',(#23885)) ;
#4878=EDGE_LOOP('',(#23886)) ;
#4879=EDGE_LOOP('',(#23887)) ;
#4880=EDGE_LOOP('',(#23888)) ;
#4881=EDGE_LOOP('',(#23889,#23890,#23891,#23892)) ;
#4882=EDGE_LOOP('',(#23893,#23894,#23895,#23896)) ;
#4883=EDGE_LOOP('',(#23897,#23898,#23899,#23900)) ;
#4884=EDGE_LOOP('',(#23901,#23902,#23903,#23904)) ;
#4885=EDGE_LOOP('',(#23905,#23906,#23907,#23908)) ;
#4886=EDGE_LOOP('',(#23909,#23910,#23911,#23912)) ;
#4887=EDGE_LOOP('',(#23913,#23914,#23915,#23916)) ;
#4888=EDGE_LOOP('',(#23917,#23918,#23919,#23920)) ;
#4889=EDGE_LOOP('',(#23921,#23922,#23923,#23924)) ;
#4890=EDGE_LOOP('',(#23925,#23926,#23927,#23928,#23929,#23930,#23931,#23932,
#23933,#23934)) ;
#4891=EDGE_LOOP('',(#23935,#23936,#23937,#23938)) ;
#4892=EDGE_LOOP('',(#23939,#23940,#23941,#23942)) ;
#4893=EDGE_LOOP('',(#23943,#23944,#23945,#23946)) ;
#4894=EDGE_LOOP('',(#23947,#23948,#23949,#23950)) ;
#4895=EDGE_LOOP('',(#23951,#23952,#23953,#23954)) ;
#4896=EDGE_LOOP('',(#23955,#23956,#23957,#23958)) ;
#4897=EDGE_LOOP('',(#23959,#23960,#23961,#23962)) ;
#4898=EDGE_LOOP('',(#23963,#23964,#23965,#23966)) ;
#4899=EDGE_LOOP('',(#23967,#23968,#23969,#23970)) ;
#4900=EDGE_LOOP('',(#23971,#23972,#23973,#23974)) ;
#4901=EDGE_LOOP('',(#23975,#23976,#23977,#23978)) ;
#4902=EDGE_LOOP('',(#23979,#23980,#23981,#23982,#23983,#23984,#23985,#23986,
#23987,#23988)) ;
#4903=EDGE_LOOP('',(#23989,#23990,#23991,#23992)) ;
#4904=EDGE_LOOP('',(#23993,#23994,#23995,#23996)) ;
#4905=EDGE_LOOP('',(#23997,#23998,#23999,#24000)) ;
#4906=EDGE_LOOP('',(#24001,#24002,#24003,#24004)) ;
#4907=EDGE_LOOP('',(#24005,#24006,#24007,#24008)) ;
#4908=EDGE_LOOP('',(#24009,#24010,#24011,#24012)) ;
#4909=EDGE_LOOP('',(#24013,#24014,#24015,#24016)) ;
#4910=EDGE_LOOP('',(#24017,#24018,#24019,#24020)) ;
#4911=EDGE_LOOP('',(#24021,#24022,#24023,#24024)) ;
#4912=EDGE_LOOP('',(#24025,#24026,#24027,#24028)) ;
#4913=EDGE_LOOP('',(#24029,#24030,#24031,#24032)) ;
#4914=EDGE_LOOP('',(#24033,#24034,#24035,#24036,#24037,#24038,#24039,#24040,
#24041,#24042)) ;
#4915=EDGE_LOOP('',(#24043,#24044,#24045,#24046)) ;
#4916=EDGE_LOOP('',(#24047,#24048,#24049,#24050)) ;
#4917=EDGE_LOOP('',(#24051,#24052,#24053,#24054)) ;
#4918=EDGE_LOOP('',(#24055,#24056,#24057,#24058)) ;
#4919=EDGE_LOOP('',(#24059,#24060,#24061,#24062)) ;
#4920=EDGE_LOOP('',(#24063,#24064,#24065,#24066)) ;
#4921=EDGE_LOOP('',(#24067,#24068,#24069,#24070)) ;
#4922=EDGE_LOOP('',(#24071,#24072,#24073,#24074)) ;
#4923=EDGE_LOOP('',(#24075,#24076,#24077,#24078)) ;
#4924=EDGE_LOOP('',(#24079,#24080,#24081,#24082)) ;
#4925=EDGE_LOOP('',(#24083,#24084,#24085,#24086)) ;
#4926=EDGE_LOOP('',(#24087,#24088,#24089,#24090,#24091,#24092,#24093,#24094,
#24095,#24096)) ;
#4927=EDGE_LOOP('',(#24097,#24098,#24099,#24100)) ;
#4928=EDGE_LOOP('',(#24101,#24102,#24103,#24104)) ;
#4929=EDGE_LOOP('',(#24105,#24106,#24107,#24108)) ;
#4930=EDGE_LOOP('',(#24109,#24110,#24111,#24112)) ;
#4931=EDGE_LOOP('',(#24113,#24114,#24115,#24116)) ;
#4932=EDGE_LOOP('',(#24117,#24118,#24119,#24120)) ;
#4933=EDGE_LOOP('',(#24121,#24122,#24123,#24124)) ;
#4934=EDGE_LOOP('',(#24125,#24126,#24127,#24128)) ;
#4935=EDGE_LOOP('',(#24129,#24130,#24131,#24132)) ;
#4936=EDGE_LOOP('',(#24133,#24134,#24135,#24136)) ;
#4937=EDGE_LOOP('',(#24137,#24138,#24139,#24140)) ;
#4938=EDGE_LOOP('',(#24141,#24142,#24143,#24144,#24145,#24146,#24147,#24148,
#24149,#24150)) ;
#4939=EDGE_LOOP('',(#24151,#24152,#24153,#24154)) ;
#4940=EDGE_LOOP('',(#24155,#24156,#24157,#24158)) ;
#4941=EDGE_LOOP('',(#24159,#24160,#24161,#24162)) ;
#4942=EDGE_LOOP('',(#24163,#24164,#24165,#24166)) ;
#4943=EDGE_LOOP('',(#24167,#24168,#24169,#24170)) ;
#4944=EDGE_LOOP('',(#24171,#24172,#24173,#24174)) ;
#4945=EDGE_LOOP('',(#24175,#24176,#24177,#24178)) ;
#4946=EDGE_LOOP('',(#24179,#24180,#24181,#24182)) ;
#4947=EDGE_LOOP('',(#24183,#24184,#24185,#24186)) ;
#4948=EDGE_LOOP('',(#24187,#24188,#24189,#24190)) ;
#4949=EDGE_LOOP('',(#24191,#24192,#24193,#24194)) ;
#4950=EDGE_LOOP('',(#24195,#24196,#24197,#24198,#24199,#24200,#24201,#24202,
#24203,#24204)) ;
#4951=EDGE_LOOP('',(#24205,#24206,#24207,#24208)) ;
#4952=EDGE_LOOP('',(#24209,#24210,#24211,#24212)) ;
#4953=EDGE_LOOP('',(#24213,#24214,#24215,#24216)) ;
#4954=EDGE_LOOP('',(#24217,#24218,#24219,#24220)) ;
#4955=EDGE_LOOP('',(#24221,#24222,#24223,#24224)) ;
#4956=EDGE_LOOP('',(#24225,#24226,#24227,#24228)) ;
#4957=EDGE_LOOP('',(#24229,#24230,#24231,#24232)) ;
#4958=EDGE_LOOP('',(#24233,#24234,#24235,#24236)) ;
#4959=EDGE_LOOP('',(#24237,#24238,#24239,#24240)) ;
#4960=EDGE_LOOP('',(#24241,#24242,#24243,#24244)) ;
#4961=EDGE_LOOP('',(#24245,#24246,#24247,#24248)) ;
#4962=EDGE_LOOP('',(#24249,#24250,#24251,#24252,#24253,#24254,#24255,#24256,
#24257,#24258)) ;
#4963=EDGE_LOOP('',(#24259,#24260,#24261,#24262)) ;
#4964=EDGE_LOOP('',(#24263,#24264,#24265,#24266)) ;
#4965=EDGE_LOOP('',(#24267,#24268,#24269,#24270)) ;
#4966=EDGE_LOOP('',(#24271,#24272,#24273,#24274)) ;
#4967=EDGE_LOOP('',(#24275,#24276,#24277,#24278)) ;
#4968=EDGE_LOOP('',(#24279,#24280,#24281,#24282)) ;
#4969=EDGE_LOOP('',(#24283,#24284,#24285,#24286)) ;
#4970=EDGE_LOOP('',(#24287,#24288,#24289,#24290)) ;
#4971=EDGE_LOOP('',(#24291,#24292,#24293,#24294)) ;
#4972=EDGE_LOOP('',(#24295,#24296,#24297,#24298)) ;
#4973=EDGE_LOOP('',(#24299,#24300,#24301,#24302)) ;
#4974=EDGE_LOOP('',(#24303,#24304,#24305,#24306,#24307,#24308,#24309,#24310,
#24311,#24312)) ;
#4975=EDGE_LOOP('',(#24313,#24314,#24315,#24316)) ;
#4976=EDGE_LOOP('',(#24317,#24318,#24319,#24320)) ;
#4977=EDGE_LOOP('',(#24321,#24322,#24323,#24324)) ;
#4978=EDGE_LOOP('',(#24325,#24326,#24327,#24328)) ;
#4979=EDGE_LOOP('',(#24329,#24330,#24331,#24332)) ;
#4980=EDGE_LOOP('',(#24333,#24334,#24335,#24336)) ;
#4981=EDGE_LOOP('',(#24337,#24338,#24339,#24340)) ;
#4982=EDGE_LOOP('',(#24341,#24342,#24343,#24344)) ;
#4983=EDGE_LOOP('',(#24345,#24346,#24347,#24348)) ;
#4984=EDGE_LOOP('',(#24349,#24350,#24351,#24352)) ;
#4985=EDGE_LOOP('',(#24353,#24354,#24355,#24356)) ;
#4986=EDGE_LOOP('',(#24357,#24358,#24359,#24360,#24361,#24362,#24363,#24364,
#24365,#24366)) ;
#4987=EDGE_LOOP('',(#24367,#24368,#24369,#24370)) ;
#4988=EDGE_LOOP('',(#24371,#24372,#24373,#24374)) ;
#4989=EDGE_LOOP('',(#24375,#24376,#24377,#24378)) ;
#4990=EDGE_LOOP('',(#24379,#24380,#24381,#24382)) ;
#4991=EDGE_LOOP('',(#24383,#24384,#24385,#24386)) ;
#4992=EDGE_LOOP('',(#24387,#24388,#24389,#24390)) ;
#4993=EDGE_LOOP('',(#24391,#24392,#24393,#24394)) ;
#4994=EDGE_LOOP('',(#24395,#24396,#24397,#24398)) ;
#4995=EDGE_LOOP('',(#24399,#24400,#24401,#24402)) ;
#4996=EDGE_LOOP('',(#24403,#24404,#24405,#24406)) ;
#4997=EDGE_LOOP('',(#24407,#24408,#24409,#24410)) ;
#4998=EDGE_LOOP('',(#24411,#24412,#24413,#24414)) ;
#4999=EDGE_LOOP('',(#24415,#24416,#24417,#24418)) ;
#5000=EDGE_LOOP('',(#24419,#24420,#24421,#24422)) ;
#5001=EDGE_LOOP('',(#24423,#24424,#24425,#24426)) ;
#5002=EDGE_LOOP('',(#24427,#24428,#24429,#24430)) ;
#5003=EDGE_LOOP('',(#24431,#24432,#24433,#24434)) ;
#5004=EDGE_LOOP('',(#24435,#24436,#24437,#24438)) ;
#5005=EDGE_LOOP('',(#24439,#24440,#24441,#24442)) ;
#5006=EDGE_LOOP('',(#24443,#24444,#24445,#24446)) ;
#5007=EDGE_LOOP('',(#24447,#24448,#24449,#24450)) ;
#5008=EDGE_LOOP('',(#24451,#24452,#24453,#24454)) ;
#5009=EDGE_LOOP('',(#24455,#24456,#24457,#24458)) ;
#5010=EDGE_LOOP('',(#24459,#24460,#24461,#24462)) ;
#5011=EDGE_LOOP('',(#24463,#24464,#24465,#24466)) ;
#5012=EDGE_LOOP('',(#24467,#24468,#24469,#24470)) ;
#5013=EDGE_LOOP('',(#24471,#24472,#24473,#24474)) ;
#5014=EDGE_LOOP('',(#24475,#24476,#24477,#24478)) ;
#5015=EDGE_LOOP('',(#24479,#24480,#24481,#24482)) ;
#5016=EDGE_LOOP('',(#24483,#24484,#24485,#24486)) ;
#5017=EDGE_LOOP('',(#24487,#24488,#24489,#24490)) ;
#5018=EDGE_LOOP('',(#24491,#24492,#24493,#24494)) ;
#5019=EDGE_LOOP('',(#24495,#24496,#24497,#24498)) ;
#5020=EDGE_LOOP('',(#24499,#24500,#24501,#24502)) ;
#5021=EDGE_LOOP('',(#24503,#24504,#24505,#24506)) ;
#5022=EDGE_LOOP('',(#24507,#24508,#24509,#24510)) ;
#5023=EDGE_LOOP('',(#24511,#24512,#24513,#24514)) ;
#5024=EDGE_LOOP('',(#24515,#24516,#24517,#24518)) ;
#5025=EDGE_LOOP('',(#24519,#24520,#24521,#24522)) ;
#5026=EDGE_LOOP('',(#24523,#24524,#24525,#24526)) ;
#5027=EDGE_LOOP('',(#24527,#24528,#24529,#24530)) ;
#5028=EDGE_LOOP('',(#24531,#24532,#24533,#24534)) ;
#5029=EDGE_LOOP('',(#24535,#24536,#24537,#24538)) ;
#5030=EDGE_LOOP('',(#24539,#24540,#24541,#24542)) ;
#5031=EDGE_LOOP('',(#24543,#24544,#24545,#24546)) ;
#5032=EDGE_LOOP('',(#24547,#24548,#24549,#24550)) ;
#5033=EDGE_LOOP('',(#24551,#24552,#24553,#24554)) ;
#5034=EDGE_LOOP('',(#24555,#24556,#24557,#24558)) ;
#5035=EDGE_LOOP('',(#24559,#24560,#24561,#24562)) ;
#5036=EDGE_LOOP('',(#24563,#24564,#24565,#24566)) ;
#5037=EDGE_LOOP('',(#24567,#24568,#24569,#24570)) ;
#5038=EDGE_LOOP('',(#24571,#24572,#24573,#24574)) ;
#5039=EDGE_LOOP('',(#24575,#24576,#24577,#24578)) ;
#5040=EDGE_LOOP('',(#24579,#24580,#24581,#24582)) ;
#5041=EDGE_LOOP('',(#24583,#24584,#24585,#24586)) ;
#5042=EDGE_LOOP('',(#24587,#24588,#24589,#24590)) ;
#5043=EDGE_LOOP('',(#24591,#24592,#24593,#24594)) ;
#5044=EDGE_LOOP('',(#24595,#24596,#24597,#24598)) ;
#5045=EDGE_LOOP('',(#24599,#24600,#24601,#24602)) ;
#5046=EDGE_LOOP('',(#24603,#24604,#24605,#24606)) ;
#5047=EDGE_LOOP('',(#24607,#24608,#24609,#24610)) ;
#5048=EDGE_LOOP('',(#24611,#24612,#24613,#24614)) ;
#5049=EDGE_LOOP('',(#24615,#24616,#24617,#24618)) ;
#5050=EDGE_LOOP('',(#24619,#24620,#24621,#24622)) ;
#5051=EDGE_LOOP('',(#24623,#24624,#24625,#24626)) ;
#5052=EDGE_LOOP('',(#24627,#24628,#24629,#24630)) ;
#5053=EDGE_LOOP('',(#24631,#24632,#24633,#24634)) ;
#5054=EDGE_LOOP('',(#24635,#24636,#24637,#24638)) ;
#5055=EDGE_LOOP('',(#24639,#24640,#24641,#24642)) ;
#5056=EDGE_LOOP('',(#24643,#24644,#24645,#24646)) ;
#5057=EDGE_LOOP('',(#24647,#24648,#24649,#24650)) ;
#5058=EDGE_LOOP('',(#24651,#24652,#24653,#24654)) ;
#5059=EDGE_LOOP('',(#24655,#24656,#24657,#24658)) ;
#5060=EDGE_LOOP('',(#24659,#24660,#24661,#24662)) ;
#5061=EDGE_LOOP('',(#24663,#24664,#24665,#24666)) ;
#5062=EDGE_LOOP('',(#24667,#24668,#24669,#24670)) ;
#5063=EDGE_LOOP('',(#24671,#24672,#24673,#24674)) ;
#5064=EDGE_LOOP('',(#24675,#24676,#24677,#24678)) ;
#5065=EDGE_LOOP('',(#24679,#24680,#24681,#24682)) ;
#5066=EDGE_LOOP('',(#24683,#24684,#24685,#24686)) ;
#5067=EDGE_LOOP('',(#24687,#24688,#24689,#24690)) ;
#5068=EDGE_LOOP('',(#24691,#24692,#24693,#24694)) ;
#5069=EDGE_LOOP('',(#24695,#24696,#24697,#24698)) ;
#5070=EDGE_LOOP('',(#24699,#24700,#24701,#24702)) ;
#5071=EDGE_LOOP('',(#24703,#24704,#24705,#24706)) ;
#5072=EDGE_LOOP('',(#24707,#24708,#24709,#24710)) ;
#5073=EDGE_LOOP('',(#24711,#24712,#24713,#24714)) ;
#5074=EDGE_LOOP('',(#24715,#24716,#24717,#24718)) ;
#5075=EDGE_LOOP('',(#24719,#24720,#24721,#24722)) ;
#5076=EDGE_LOOP('',(#24723,#24724,#24725,#24726)) ;
#5077=EDGE_LOOP('',(#24727,#24728,#24729,#24730)) ;
#5078=EDGE_LOOP('',(#24731,#24732,#24733,#24734)) ;
#5079=EDGE_LOOP('',(#24735,#24736,#24737,#24738)) ;
#5080=EDGE_LOOP('',(#24739,#24740,#24741,#24742)) ;
#5081=EDGE_LOOP('',(#24743,#24744,#24745,#24746)) ;
#5082=EDGE_LOOP('',(#24747,#24748,#24749,#24750)) ;
#5083=EDGE_LOOP('',(#24751,#24752,#24753,#24754)) ;
#5084=EDGE_LOOP('',(#24755,#24756,#24757,#24758)) ;
#5085=EDGE_LOOP('',(#24759,#24760,#24761,#24762)) ;
#5086=EDGE_LOOP('',(#24763,#24764,#24765,#24766)) ;
#5087=EDGE_LOOP('',(#24767,#24768,#24769,#24770)) ;
#5088=EDGE_LOOP('',(#24771,#24772,#24773,#24774)) ;
#5089=EDGE_LOOP('',(#24775,#24776,#24777,#24778)) ;
#5090=EDGE_LOOP('',(#24779,#24780,#24781,#24782)) ;
#5091=EDGE_LOOP('',(#24783,#24784,#24785,#24786)) ;
#5092=EDGE_LOOP('',(#24787,#24788,#24789,#24790)) ;
#5093=EDGE_LOOP('',(#24791,#24792,#24793,#24794)) ;
#5094=EDGE_LOOP('',(#24795,#24796,#24797,#24798,#24799,#24800,#24801,#24802,
#24803,#24804)) ;
#5095=EDGE_LOOP('',(#24805,#24806,#24807,#24808)) ;
#5096=EDGE_LOOP('',(#24809,#24810,#24811,#24812)) ;
#5097=EDGE_LOOP('',(#24813,#24814,#24815,#24816)) ;
#5098=EDGE_LOOP('',(#24817,#24818,#24819,#24820)) ;
#5099=EDGE_LOOP('',(#24821,#24822,#24823,#24824)) ;
#5100=EDGE_LOOP('',(#24825,#24826,#24827,#24828)) ;
#5101=EDGE_LOOP('',(#24829,#24830,#24831,#24832)) ;
#5102=EDGE_LOOP('',(#24833,#24834,#24835,#24836)) ;
#5103=EDGE_LOOP('',(#24837,#24838,#24839,#24840)) ;
#5104=EDGE_LOOP('',(#24841,#24842,#24843,#24844)) ;
#5105=EDGE_LOOP('',(#24845,#24846,#24847,#24848)) ;
#5106=EDGE_LOOP('',(#24849,#24850,#24851,#24852,#24853,#24854,#24855,#24856,
#24857,#24858)) ;
#5107=EDGE_LOOP('',(#24859,#24860,#24861,#24862)) ;
#5108=EDGE_LOOP('',(#24863,#24864,#24865,#24866)) ;
#5109=EDGE_LOOP('',(#24867,#24868,#24869,#24870)) ;
#5110=EDGE_LOOP('',(#24871,#24872,#24873,#24874)) ;
#5111=EDGE_LOOP('',(#24875,#24876,#24877,#24878)) ;
#5112=EDGE_LOOP('',(#24879,#24880,#24881,#24882)) ;
#5113=EDGE_LOOP('',(#24883,#24884,#24885,#24886)) ;
#5114=EDGE_LOOP('',(#24887,#24888,#24889,#24890)) ;
#5115=EDGE_LOOP('',(#24891,#24892,#24893,#24894)) ;
#5116=EDGE_LOOP('',(#24895,#24896,#24897,#24898)) ;
#5117=EDGE_LOOP('',(#24899,#24900,#24901,#24902)) ;
#5118=EDGE_LOOP('',(#24903,#24904,#24905,#24906,#24907,#24908,#24909,#24910,
#24911,#24912)) ;
#5119=EDGE_LOOP('',(#24913,#24914,#24915,#24916)) ;
#5120=EDGE_LOOP('',(#24917,#24918,#24919,#24920)) ;
#5121=EDGE_LOOP('',(#24921,#24922,#24923,#24924)) ;
#5122=EDGE_LOOP('',(#24925,#24926,#24927,#24928)) ;
#5123=EDGE_LOOP('',(#24929,#24930,#24931,#24932)) ;
#5124=EDGE_LOOP('',(#24933,#24934,#24935,#24936)) ;
#5125=EDGE_LOOP('',(#24937,#24938,#24939,#24940)) ;
#5126=EDGE_LOOP('',(#24941,#24942,#24943,#24944)) ;
#5127=EDGE_LOOP('',(#24945,#24946,#24947,#24948)) ;
#5128=EDGE_LOOP('',(#24949,#24950,#24951,#24952)) ;
#5129=EDGE_LOOP('',(#24953,#24954,#24955,#24956)) ;
#5130=EDGE_LOOP('',(#24957,#24958,#24959,#24960,#24961,#24962,#24963,#24964,
#24965,#24966)) ;
#5131=EDGE_LOOP('',(#24967,#24968,#24969,#24970)) ;
#5132=EDGE_LOOP('',(#24971,#24972,#24973,#24974)) ;
#5133=EDGE_LOOP('',(#24975,#24976,#24977,#24978)) ;
#5134=EDGE_LOOP('',(#24979,#24980,#24981,#24982)) ;
#5135=EDGE_LOOP('',(#24983,#24984,#24985,#24986)) ;
#5136=EDGE_LOOP('',(#24987,#24988,#24989,#24990)) ;
#5137=EDGE_LOOP('',(#24991,#24992,#24993,#24994)) ;
#5138=EDGE_LOOP('',(#24995,#24996,#24997,#24998)) ;
#5139=EDGE_LOOP('',(#24999,#25000,#25001,#25002)) ;
#5140=EDGE_LOOP('',(#25003,#25004,#25005,#25006)) ;
#5141=EDGE_LOOP('',(#25007,#25008,#25009,#25010)) ;
#5142=EDGE_LOOP('',(#25011,#25012,#25013,#25014,#25015,#25016,#25017,#25018,
#25019,#25020)) ;
#5143=EDGE_LOOP('',(#25021,#25022,#25023,#25024)) ;
#5144=EDGE_LOOP('',(#25025,#25026,#25027,#25028)) ;
#5145=EDGE_LOOP('',(#25029,#25030,#25031,#25032)) ;
#5146=EDGE_LOOP('',(#25033,#25034,#25035,#25036)) ;
#5147=EDGE_LOOP('',(#25037,#25038,#25039,#25040)) ;
#5148=EDGE_LOOP('',(#25041,#25042,#25043,#25044)) ;
#5149=EDGE_LOOP('',(#25045,#25046,#25047,#25048)) ;
#5150=EDGE_LOOP('',(#25049,#25050,#25051,#25052)) ;
#5151=EDGE_LOOP('',(#25053,#25054,#25055,#25056)) ;
#5152=EDGE_LOOP('',(#25057,#25058,#25059,#25060)) ;
#5153=EDGE_LOOP('',(#25061,#25062,#25063,#25064)) ;
#5154=EDGE_LOOP('',(#25065,#25066,#25067,#25068,#25069,#25070,#25071,#25072,
#25073,#25074)) ;
#5155=EDGE_LOOP('',(#25075,#25076,#25077,#25078)) ;
#5156=EDGE_LOOP('',(#25079,#25080,#25081,#25082)) ;
#5157=EDGE_LOOP('',(#25083,#25084,#25085,#25086)) ;
#5158=EDGE_LOOP('',(#25087,#25088,#25089,#25090)) ;
#5159=EDGE_LOOP('',(#25091,#25092,#25093,#25094)) ;
#5160=EDGE_LOOP('',(#25095,#25096,#25097,#25098)) ;
#5161=EDGE_LOOP('',(#25099,#25100,#25101,#25102)) ;
#5162=EDGE_LOOP('',(#25103,#25104,#25105,#25106)) ;
#5163=EDGE_LOOP('',(#25107,#25108,#25109,#25110)) ;
#5164=EDGE_LOOP('',(#25111,#25112,#25113,#25114)) ;
#5165=EDGE_LOOP('',(#25115,#25116,#25117,#25118)) ;
#5166=EDGE_LOOP('',(#25119,#25120,#25121,#25122,#25123,#25124,#25125,#25126,
#25127,#25128)) ;
#5167=EDGE_LOOP('',(#25129,#25130,#25131,#25132)) ;
#5168=EDGE_LOOP('',(#25133,#25134,#25135,#25136)) ;
#5169=EDGE_LOOP('',(#25137,#25138,#25139,#25140)) ;
#5170=EDGE_LOOP('',(#25141,#25142,#25143,#25144)) ;
#5171=EDGE_LOOP('',(#25145,#25146,#25147,#25148)) ;
#5172=EDGE_LOOP('',(#25149,#25150,#25151,#25152)) ;
#5173=EDGE_LOOP('',(#25153,#25154,#25155,#25156)) ;
#5174=EDGE_LOOP('',(#25157,#25158,#25159,#25160)) ;
#5175=EDGE_LOOP('',(#25161,#25162,#25163,#25164)) ;
#5176=EDGE_LOOP('',(#25165,#25166,#25167,#25168)) ;
#5177=EDGE_LOOP('',(#25169,#25170,#25171,#25172)) ;
#5178=EDGE_LOOP('',(#25173,#25174,#25175,#25176,#25177,#25178,#25179,#25180,
#25181,#25182)) ;
#5179=EDGE_LOOP('',(#25183,#25184,#25185,#25186)) ;
#5180=EDGE_LOOP('',(#25187,#25188,#25189,#25190)) ;
#5181=EDGE_LOOP('',(#25191,#25192,#25193,#25194)) ;
#5182=EDGE_LOOP('',(#25195,#25196,#25197,#25198)) ;
#5183=EDGE_LOOP('',(#25199,#25200,#25201,#25202)) ;
#5184=EDGE_LOOP('',(#25203,#25204,#25205,#25206)) ;
#5185=EDGE_LOOP('',(#25207,#25208,#25209,#25210)) ;
#5186=EDGE_LOOP('',(#25211,#25212,#25213,#25214)) ;
#5187=EDGE_LOOP('',(#25215,#25216,#25217,#25218)) ;
#5188=EDGE_LOOP('',(#25219,#25220,#25221,#25222)) ;
#5189=EDGE_LOOP('',(#25223,#25224,#25225,#25226)) ;
#5190=EDGE_LOOP('',(#25227,#25228,#25229,#25230)) ;
#5191=EDGE_LOOP('',(#25231,#25232,#25233,#25234)) ;
#5192=EDGE_LOOP('',(#25235,#25236,#25237,#25238)) ;
#5193=EDGE_LOOP('',(#25239,#25240,#25241,#25242)) ;
#5194=EDGE_LOOP('',(#25243,#25244,#25245,#25246,#25247,#25248,#25249,#25250)) ;
#5195=EDGE_LOOP('',(#25251)) ;
#5196=EDGE_LOOP('',(#25252,#25253,#25254,#25255,#25256,#25257,#25258,#25259)) ;
#5197=EDGE_LOOP('',(#25260,#25261,#25262,#25263)) ;
#5198=EDGE_LOOP('',(#25264,#25265,#25266,#25267)) ;
#5199=EDGE_LOOP('',(#25268,#25269,#25270,#25271)) ;
#5200=EDGE_LOOP('',(#25272,#25273,#25274,#25275)) ;
#5201=EDGE_LOOP('',(#25276,#25277,#25278,#25279)) ;
#5202=EDGE_LOOP('',(#25280,#25281,#25282,#25283)) ;
#5203=EDGE_LOOP('',(#25284,#25285,#25286,#25287)) ;
#5204=EDGE_LOOP('',(#25288,#25289,#25290,#25291)) ;
#5205=EDGE_LOOP('',(#25292,#25293,#25294,#25295)) ;
#5206=EDGE_LOOP('',(#25296,#25297,#25298,#25299,#25300,#25301,#25302,#25303,
#25304,#25305)) ;
#5207=EDGE_LOOP('',(#25306,#25307,#25308,#25309)) ;
#5208=EDGE_LOOP('',(#25310,#25311,#25312,#25313)) ;
#5209=EDGE_LOOP('',(#25314,#25315,#25316,#25317)) ;
#5210=EDGE_LOOP('',(#25318,#25319,#25320,#25321)) ;
#5211=EDGE_LOOP('',(#25322,#25323,#25324,#25325)) ;
#5212=EDGE_LOOP('',(#25326,#25327,#25328,#25329)) ;
#5213=EDGE_LOOP('',(#25330,#25331,#25332,#25333)) ;
#5214=EDGE_LOOP('',(#25334,#25335,#25336,#25337)) ;
#5215=EDGE_LOOP('',(#25338,#25339,#25340,#25341)) ;
#5216=EDGE_LOOP('',(#25342)) ;
#5217=EDGE_LOOP('',(#25343)) ;
#5218=EDGE_LOOP('',(#25344,#25345,#25346,#25347)) ;
#5219=EDGE_LOOP('',(#25348,#25349,#25350,#25351)) ;
#5220=EDGE_LOOP('',(#25352,#25353,#25354,#25355)) ;
#5221=EDGE_LOOP('',(#25356,#25357,#25358,#25359)) ;
#5222=EDGE_LOOP('',(#25360,#25361,#25362,#25363)) ;
#5223=EDGE_LOOP('',(#25364,#25365,#25366,#25367)) ;
#5224=EDGE_LOOP('',(#25368,#25369,#25370,#25371)) ;
#5225=EDGE_LOOP('',(#25372,#25373,#25374,#25375)) ;
#5226=EDGE_LOOP('',(#25376,#25377,#25378,#25379)) ;
#5227=EDGE_LOOP('',(#25380,#25381,#25382,#25383)) ;
#5228=EDGE_LOOP('',(#25384,#25385,#25386,#25387)) ;
#5229=EDGE_LOOP('',(#25388,#25389,#25390,#25391)) ;
#5230=EDGE_LOOP('',(#25392,#25393,#25394,#25395)) ;
#5231=EDGE_LOOP('',(#25396,#25397,#25398)) ;
#5232=EDGE_LOOP('',(#25399,#25400,#25401)) ;
#5233=EDGE_LOOP('',(#25402,#25403,#25404,#25405)) ;
#5234=EDGE_LOOP('',(#25406,#25407,#25408)) ;
#5235=EDGE_LOOP('',(#25409,#25410,#25411)) ;
#5236=EDGE_LOOP('',(#25412,#25413,#25414,#25415)) ;
#5237=EDGE_LOOP('',(#25416,#25417,#25418,#25419)) ;
#5238=EDGE_LOOP('',(#25420,#25421,#25422,#25423)) ;
#5239=EDGE_LOOP('',(#25424,#25425,#25426,#25427)) ;
#5240=EDGE_LOOP('',(#25428,#25429,#25430)) ;
#5241=EDGE_LOOP('',(#25431,#25432,#25433)) ;
#5242=EDGE_LOOP('',(#25434,#25435,#25436,#25437)) ;
#5243=EDGE_LOOP('',(#25438,#25439,#25440,#25441)) ;
#5244=EDGE_LOOP('',(#25442,#25443,#25444,#25445)) ;
#5245=EDGE_LOOP('',(#25446,#25447,#25448,#25449)) ;
#5246=EDGE_LOOP('',(#25450,#25451,#25452)) ;
#5247=EDGE_LOOP('',(#25453,#25454,#25455)) ;
#5248=EDGE_LOOP('',(#25456,#25457,#25458,#25459)) ;
#5249=EDGE_LOOP('',(#25460,#25461,#25462,#25463)) ;
#5250=EDGE_LOOP('',(#25464,#25465,#25466,#25467)) ;
#5251=EDGE_LOOP('',(#25468,#25469,#25470,#25471)) ;
#5252=EDGE_LOOP('',(#25472,#25473,#25474,#25475)) ;
#5253=EDGE_LOOP('',(#25476,#25477,#25478,#25479)) ;
#5254=EDGE_LOOP('',(#25480,#25481,#25482,#25483)) ;
#5255=EDGE_LOOP('',(#25484,#25485,#25486,#25487)) ;
#5256=EDGE_LOOP('',(#25488,#25489,#25490,#25491)) ;
#5257=EDGE_LOOP('',(#25492,#25493,#25494,#25495)) ;
#5258=EDGE_LOOP('',(#25496,#25497,#25498,#25499)) ;
#5259=EDGE_LOOP('',(#25500,#25501,#25502,#25503)) ;
#5260=EDGE_LOOP('',(#25504,#25505,#25506,#25507)) ;
#5261=EDGE_LOOP('',(#25508,#25509,#25510)) ;
#5262=EDGE_LOOP('',(#25511,#25512,#25513)) ;
#5263=EDGE_LOOP('',(#25514,#25515,#25516,#25517)) ;
#5264=EDGE_LOOP('',(#25518,#25519,#25520)) ;
#5265=EDGE_LOOP('',(#25521,#25522,#25523)) ;
#5266=EDGE_LOOP('',(#25524,#25525,#25526,#25527)) ;
#5267=EDGE_LOOP('',(#25528,#25529,#25530,#25531)) ;
#5268=EDGE_LOOP('',(#25532,#25533,#25534,#25535)) ;
#5269=EDGE_LOOP('',(#25536,#25537,#25538,#25539)) ;
#5270=EDGE_LOOP('',(#25540,#25541,#25542)) ;
#5271=EDGE_LOOP('',(#25543,#25544,#25545)) ;
#5272=EDGE_LOOP('',(#25546,#25547,#25548,#25549)) ;
#5273=EDGE_LOOP('',(#25550,#25551,#25552,#25553)) ;
#5274=EDGE_LOOP('',(#25554,#25555,#25556,#25557)) ;
#5275=EDGE_LOOP('',(#25558,#25559,#25560,#25561)) ;
#5276=EDGE_LOOP('',(#25562,#25563,#25564)) ;
#5277=EDGE_LOOP('',(#25565,#25566,#25567)) ;
#5278=EDGE_LOOP('',(#25568,#25569,#25570,#25571)) ;
#5279=EDGE_LOOP('',(#25572,#25573,#25574,#25575)) ;
#5280=EDGE_LOOP('',(#25576,#25577,#25578,#25579)) ;
#5281=EDGE_LOOP('',(#25580,#25581,#25582,#25583)) ;
#5282=EDGE_LOOP('',(#25584,#25585,#25586,#25587)) ;
#5283=EDGE_LOOP('',(#25588,#25589,#25590,#25591)) ;
#5284=EDGE_LOOP('',(#25592,#25593,#25594,#25595)) ;
#5285=EDGE_LOOP('',(#25596,#25597,#25598,#25599)) ;
#5286=EDGE_LOOP('',(#25600,#25601,#25602,#25603)) ;
#5287=EDGE_LOOP('',(#25604,#25605,#25606,#25607)) ;
#5288=EDGE_LOOP('',(#25608,#25609,#25610,#25611)) ;
#5289=EDGE_LOOP('',(#25612,#25613,#25614,#25615)) ;
#5290=EDGE_LOOP('',(#25616,#25617,#25618,#25619)) ;
#5291=EDGE_LOOP('',(#25620,#25621,#25622)) ;
#5292=EDGE_LOOP('',(#25623,#25624,#25625)) ;
#5293=EDGE_LOOP('',(#25626,#25627,#25628,#25629)) ;
#5294=EDGE_LOOP('',(#25630,#25631,#25632)) ;
#5295=EDGE_LOOP('',(#25633,#25634,#25635)) ;
#5296=EDGE_LOOP('',(#25636,#25637,#25638,#25639)) ;
#5297=EDGE_LOOP('',(#25640,#25641,#25642,#25643)) ;
#5298=EDGE_LOOP('',(#25644,#25645,#25646,#25647)) ;
#5299=EDGE_LOOP('',(#25648,#25649,#25650,#25651)) ;
#5300=EDGE_LOOP('',(#25652,#25653,#25654)) ;
#5301=EDGE_LOOP('',(#25655,#25656,#25657)) ;
#5302=EDGE_LOOP('',(#25658,#25659,#25660,#25661)) ;
#5303=EDGE_LOOP('',(#25662,#25663,#25664,#25665)) ;
#5304=EDGE_LOOP('',(#25666,#25667,#25668,#25669)) ;
#5305=EDGE_LOOP('',(#25670,#25671,#25672,#25673)) ;
#5306=EDGE_LOOP('',(#25674,#25675,#25676)) ;
#5307=EDGE_LOOP('',(#25677,#25678,#25679)) ;
#5308=EDGE_LOOP('',(#25680,#25681,#25682,#25683)) ;
#5309=EDGE_LOOP('',(#25684,#25685,#25686,#25687)) ;
#5310=EDGE_LOOP('',(#25688,#25689,#25690,#25691)) ;
#5311=EDGE_LOOP('',(#25692,#25693,#25694,#25695)) ;
#5312=EDGE_LOOP('',(#25696,#25697,#25698,#25699)) ;
#5313=EDGE_LOOP('',(#25700,#25701,#25702,#25703)) ;
#5314=EDGE_LOOP('',(#25704,#25705,#25706,#25707)) ;
#5315=EDGE_LOOP('',(#25708,#25709,#25710,#25711)) ;
#5316=EDGE_LOOP('',(#25712,#25713,#25714,#25715)) ;
#5317=EDGE_LOOP('',(#25716,#25717,#25718,#25719)) ;
#5318=EDGE_LOOP('',(#25720,#25721,#25722,#25723)) ;
#5319=EDGE_LOOP('',(#25724,#25725,#25726,#25727)) ;
#5320=EDGE_LOOP('',(#25728,#25729,#25730,#25731)) ;
#5321=EDGE_LOOP('',(#25732,#25733,#25734)) ;
#5322=EDGE_LOOP('',(#25735,#25736,#25737)) ;
#5323=EDGE_LOOP('',(#25738,#25739,#25740,#25741)) ;
#5324=EDGE_LOOP('',(#25742,#25743,#25744)) ;
#5325=EDGE_LOOP('',(#25745,#25746,#25747)) ;
#5326=EDGE_LOOP('',(#25748,#25749,#25750,#25751)) ;
#5327=EDGE_LOOP('',(#25752,#25753,#25754,#25755)) ;
#5328=EDGE_LOOP('',(#25756,#25757,#25758,#25759)) ;
#5329=EDGE_LOOP('',(#25760,#25761,#25762,#25763)) ;
#5330=EDGE_LOOP('',(#25764,#25765,#25766)) ;
#5331=EDGE_LOOP('',(#25767,#25768,#25769)) ;
#5332=EDGE_LOOP('',(#25770,#25771,#25772,#25773)) ;
#5333=EDGE_LOOP('',(#25774,#25775,#25776,#25777)) ;
#5334=EDGE_LOOP('',(#25778,#25779,#25780,#25781)) ;
#5335=EDGE_LOOP('',(#25782,#25783,#25784,#25785)) ;
#5336=EDGE_LOOP('',(#25786,#25787,#25788)) ;
#5337=EDGE_LOOP('',(#25789,#25790,#25791)) ;
#5338=EDGE_LOOP('',(#25792,#25793,#25794,#25795)) ;
#5339=EDGE_LOOP('',(#25796,#25797,#25798,#25799)) ;
#5340=EDGE_LOOP('',(#25800,#25801,#25802,#25803)) ;
#5341=EDGE_LOOP('',(#25804,#25805,#25806,#25807)) ;
#5342=EDGE_LOOP('',(#25808,#25809,#25810,#25811)) ;
#5343=EDGE_LOOP('',(#25812,#25813,#25814,#25815)) ;
#5344=EDGE_LOOP('',(#25816,#25817,#25818,#25819)) ;
#5345=EDGE_LOOP('',(#25820,#25821,#25822,#25823)) ;
#5346=EDGE_LOOP('',(#25824,#25825,#25826,#25827)) ;
#5347=EDGE_LOOP('',(#25828,#25829,#25830,#25831)) ;
#5348=EDGE_LOOP('',(#25832,#25833,#25834,#25835)) ;
#5349=EDGE_LOOP('',(#25836,#25837,#25838,#25839)) ;
#5350=EDGE_LOOP('',(#25840,#25841,#25842,#25843)) ;
#5351=EDGE_LOOP('',(#25844,#25845,#25846)) ;
#5352=EDGE_LOOP('',(#25847,#25848,#25849)) ;
#5353=EDGE_LOOP('',(#25850,#25851,#25852,#25853)) ;
#5354=EDGE_LOOP('',(#25854,#25855,#25856)) ;
#5355=EDGE_LOOP('',(#25857,#25858,#25859)) ;
#5356=EDGE_LOOP('',(#25860,#25861,#25862,#25863)) ;
#5357=EDGE_LOOP('',(#25864,#25865,#25866,#25867)) ;
#5358=EDGE_LOOP('',(#25868,#25869,#25870,#25871)) ;
#5359=EDGE_LOOP('',(#25872,#25873,#25874,#25875)) ;
#5360=EDGE_LOOP('',(#25876,#25877,#25878)) ;
#5361=EDGE_LOOP('',(#25879,#25880,#25881)) ;
#5362=EDGE_LOOP('',(#25882,#25883,#25884,#25885)) ;
#5363=EDGE_LOOP('',(#25886,#25887,#25888,#25889)) ;
#5364=EDGE_LOOP('',(#25890,#25891,#25892,#25893)) ;
#5365=EDGE_LOOP('',(#25894,#25895,#25896,#25897)) ;
#5366=EDGE_LOOP('',(#25898,#25899,#25900)) ;
#5367=EDGE_LOOP('',(#25901,#25902,#25903)) ;
#5368=EDGE_LOOP('',(#25904,#25905,#25906,#25907)) ;
#5369=EDGE_LOOP('',(#25908,#25909,#25910,#25911)) ;
#5370=EDGE_LOOP('',(#25912,#25913,#25914,#25915)) ;
#5371=EDGE_LOOP('',(#25916,#25917,#25918,#25919)) ;
#5372=EDGE_LOOP('',(#25920,#25921,#25922,#25923)) ;
#5373=EDGE_LOOP('',(#25924,#25925,#25926,#25927)) ;
#5374=EDGE_LOOP('',(#25928,#25929,#25930,#25931)) ;
#5375=EDGE_LOOP('',(#25932,#25933,#25934,#25935)) ;
#5376=EDGE_LOOP('',(#25936,#25937,#25938,#25939)) ;
#5377=EDGE_LOOP('',(#25940,#25941,#25942,#25943)) ;
#5378=EDGE_LOOP('',(#25944,#25945,#25946,#25947)) ;
#5379=EDGE_LOOP('',(#25948,#25949,#25950,#25951)) ;
#5380=EDGE_LOOP('',(#25952,#25953,#25954,#25955)) ;
#5381=EDGE_LOOP('',(#25956,#25957,#25958)) ;
#5382=EDGE_LOOP('',(#25959,#25960,#25961)) ;
#5383=EDGE_LOOP('',(#25962,#25963,#25964,#25965)) ;
#5384=EDGE_LOOP('',(#25966,#25967,#25968)) ;
#5385=EDGE_LOOP('',(#25969,#25970,#25971)) ;
#5386=EDGE_LOOP('',(#25972,#25973,#25974,#25975)) ;
#5387=EDGE_LOOP('',(#25976,#25977,#25978,#25979)) ;
#5388=EDGE_LOOP('',(#25980,#25981,#25982,#25983)) ;
#5389=EDGE_LOOP('',(#25984,#25985,#25986,#25987)) ;
#5390=EDGE_LOOP('',(#25988,#25989,#25990)) ;
#5391=EDGE_LOOP('',(#25991,#25992,#25993)) ;
#5392=EDGE_LOOP('',(#25994,#25995,#25996,#25997)) ;
#5393=EDGE_LOOP('',(#25998,#25999,#26000,#26001)) ;
#5394=EDGE_LOOP('',(#26002,#26003,#26004,#26005)) ;
#5395=EDGE_LOOP('',(#26006,#26007,#26008,#26009)) ;
#5396=EDGE_LOOP('',(#26010,#26011,#26012)) ;
#5397=EDGE_LOOP('',(#26013,#26014,#26015)) ;
#5398=EDGE_LOOP('',(#26016,#26017,#26018,#26019)) ;
#5399=EDGE_LOOP('',(#26020,#26021,#26022,#26023)) ;
#5400=EDGE_LOOP('',(#26024,#26025,#26026,#26027)) ;
#5401=EDGE_LOOP('',(#26028,#26029,#26030,#26031)) ;
#5402=EDGE_LOOP('',(#26032,#26033,#26034,#26035)) ;
#5403=EDGE_LOOP('',(#26036,#26037,#26038,#26039)) ;
#5404=EDGE_LOOP('',(#26040,#26041,#26042,#26043)) ;
#5405=EDGE_LOOP('',(#26044,#26045,#26046,#26047)) ;
#5406=EDGE_LOOP('',(#26048,#26049,#26050,#26051)) ;
#5407=EDGE_LOOP('',(#26052,#26053,#26054,#26055)) ;
#5408=EDGE_LOOP('',(#26056,#26057,#26058,#26059)) ;
#5409=EDGE_LOOP('',(#26060,#26061,#26062,#26063)) ;
#5410=EDGE_LOOP('',(#26064,#26065,#26066,#26067)) ;
#5411=EDGE_LOOP('',(#26068,#26069,#26070)) ;
#5412=EDGE_LOOP('',(#26071,#26072,#26073)) ;
#5413=EDGE_LOOP('',(#26074,#26075,#26076,#26077)) ;
#5414=EDGE_LOOP('',(#26078,#26079,#26080)) ;
#5415=EDGE_LOOP('',(#26081,#26082,#26083)) ;
#5416=EDGE_LOOP('',(#26084,#26085,#26086,#26087)) ;
#5417=EDGE_LOOP('',(#26088,#26089,#26090,#26091)) ;
#5418=EDGE_LOOP('',(#26092,#26093,#26094,#26095)) ;
#5419=EDGE_LOOP('',(#26096,#26097,#26098,#26099)) ;
#5420=EDGE_LOOP('',(#26100,#26101,#26102)) ;
#5421=EDGE_LOOP('',(#26103,#26104,#26105)) ;
#5422=EDGE_LOOP('',(#26106,#26107,#26108,#26109)) ;
#5423=EDGE_LOOP('',(#26110,#26111,#26112,#26113)) ;
#5424=EDGE_LOOP('',(#26114,#26115,#26116,#26117)) ;
#5425=EDGE_LOOP('',(#26118,#26119,#26120,#26121)) ;
#5426=EDGE_LOOP('',(#26122,#26123,#26124)) ;
#5427=EDGE_LOOP('',(#26125,#26126,#26127)) ;
#5428=EDGE_LOOP('',(#26128,#26129,#26130,#26131)) ;
#5429=EDGE_LOOP('',(#26132,#26133,#26134,#26135)) ;
#5430=EDGE_LOOP('',(#26136,#26137,#26138,#26139)) ;
#5431=EDGE_LOOP('',(#26140,#26141,#26142,#26143)) ;
#5432=EDGE_LOOP('',(#26144,#26145,#26146,#26147)) ;
#5433=EDGE_LOOP('',(#26148,#26149,#26150,#26151)) ;
#5434=EDGE_LOOP('',(#26152,#26153,#26154,#26155)) ;
#5435=EDGE_LOOP('',(#26156,#26157,#26158,#26159)) ;
#5436=EDGE_LOOP('',(#26160,#26161,#26162,#26163)) ;
#5437=EDGE_LOOP('',(#26164,#26165,#26166,#26167)) ;
#5438=EDGE_LOOP('',(#26168,#26169,#26170,#26171)) ;
#5439=EDGE_LOOP('',(#26172,#26173,#26174,#26175)) ;
#5440=EDGE_LOOP('',(#26176,#26177,#26178,#26179)) ;
#5441=EDGE_LOOP('',(#26180,#26181,#26182)) ;
#5442=EDGE_LOOP('',(#26183,#26184,#26185)) ;
#5443=EDGE_LOOP('',(#26186,#26187,#26188,#26189)) ;
#5444=EDGE_LOOP('',(#26190,#26191,#26192)) ;
#5445=EDGE_LOOP('',(#26193,#26194,#26195)) ;
#5446=EDGE_LOOP('',(#26196,#26197,#26198,#26199)) ;
#5447=EDGE_LOOP('',(#26200,#26201,#26202,#26203)) ;
#5448=EDGE_LOOP('',(#26204,#26205,#26206,#26207)) ;
#5449=EDGE_LOOP('',(#26208,#26209,#26210,#26211)) ;
#5450=EDGE_LOOP('',(#26212,#26213,#26214)) ;
#5451=EDGE_LOOP('',(#26215,#26216,#26217)) ;
#5452=EDGE_LOOP('',(#26218,#26219,#26220,#26221)) ;
#5453=EDGE_LOOP('',(#26222,#26223,#26224,#26225)) ;
#5454=EDGE_LOOP('',(#26226,#26227,#26228,#26229)) ;
#5455=EDGE_LOOP('',(#26230,#26231,#26232,#26233)) ;
#5456=EDGE_LOOP('',(#26234,#26235,#26236)) ;
#5457=EDGE_LOOP('',(#26237,#26238,#26239)) ;
#5458=EDGE_LOOP('',(#26240,#26241,#26242,#26243)) ;
#5459=EDGE_LOOP('',(#26244,#26245,#26246,#26247)) ;
#5460=EDGE_LOOP('',(#26248,#26249,#26250,#26251)) ;
#5461=EDGE_LOOP('',(#26252,#26253,#26254,#26255)) ;
#5462=EDGE_LOOP('',(#26256,#26257,#26258,#26259)) ;
#5463=EDGE_LOOP('',(#26260,#26261,#26262,#26263)) ;
#5464=EDGE_LOOP('',(#26264,#26265,#26266,#26267)) ;
#5465=EDGE_LOOP('',(#26268,#26269,#26270,#26271)) ;
#5466=EDGE_LOOP('',(#26272,#26273,#26274,#26275)) ;
#5467=EDGE_LOOP('',(#26276,#26277,#26278,#26279)) ;
#5468=EDGE_LOOP('',(#26280,#26281,#26282,#26283)) ;
#5469=EDGE_LOOP('',(#26284,#26285,#26286,#26287)) ;
#5470=EDGE_LOOP('',(#26288,#26289,#26290,#26291)) ;
#5471=EDGE_LOOP('',(#26292,#26293,#26294)) ;
#5472=EDGE_LOOP('',(#26295,#26296,#26297)) ;
#5473=EDGE_LOOP('',(#26298,#26299,#26300,#26301)) ;
#5474=EDGE_LOOP('',(#26302,#26303,#26304)) ;
#5475=EDGE_LOOP('',(#26305,#26306,#26307)) ;
#5476=EDGE_LOOP('',(#26308,#26309,#26310,#26311)) ;
#5477=EDGE_LOOP('',(#26312,#26313,#26314,#26315)) ;
#5478=EDGE_LOOP('',(#26316,#26317,#26318,#26319)) ;
#5479=EDGE_LOOP('',(#26320,#26321,#26322,#26323)) ;
#5480=EDGE_LOOP('',(#26324,#26325,#26326)) ;
#5481=EDGE_LOOP('',(#26327,#26328,#26329)) ;
#5482=EDGE_LOOP('',(#26330,#26331,#26332,#26333)) ;
#5483=EDGE_LOOP('',(#26334,#26335,#26336,#26337)) ;
#5484=EDGE_LOOP('',(#26338,#26339,#26340,#26341)) ;
#5485=EDGE_LOOP('',(#26342,#26343,#26344,#26345)) ;
#5486=EDGE_LOOP('',(#26346,#26347,#26348)) ;
#5487=EDGE_LOOP('',(#26349,#26350,#26351)) ;
#5488=EDGE_LOOP('',(#26352,#26353,#26354,#26355)) ;
#5489=EDGE_LOOP('',(#26356,#26357,#26358,#26359)) ;
#5490=EDGE_LOOP('',(#26360,#26361,#26362,#26363)) ;
#5491=EDGE_LOOP('',(#26364,#26365,#26366,#26367)) ;
#5492=EDGE_LOOP('',(#26368,#26369,#26370,#26371)) ;
#5493=EDGE_LOOP('',(#26372,#26373,#26374,#26375)) ;
#5494=EDGE_LOOP('',(#26376,#26377,#26378,#26379)) ;
#5495=EDGE_LOOP('',(#26380,#26381,#26382,#26383)) ;
#5496=EDGE_LOOP('',(#26384,#26385,#26386,#26387)) ;
#5497=EDGE_LOOP('',(#26388,#26389,#26390,#26391)) ;
#5498=EDGE_LOOP('',(#26392,#26393,#26394,#26395)) ;
#5499=EDGE_LOOP('',(#26396,#26397,#26398,#26399)) ;
#5500=EDGE_LOOP('',(#26400,#26401,#26402,#26403)) ;
#5501=EDGE_LOOP('',(#26404,#26405,#26406,#26407)) ;
#5502=EDGE_LOOP('',(#26408,#26409,#26410,#26411)) ;
#5503=EDGE_LOOP('',(#26412,#26413,#26414,#26415)) ;
#5504=EDGE_LOOP('',(#26416,#26417,#26418,#26419)) ;
#5505=EDGE_LOOP('',(#26420,#26421,#26422,#26423)) ;
#5506=EDGE_LOOP('',(#26424,#26425,#26426,#26427)) ;
#5507=EDGE_LOOP('',(#26428,#26429,#26430,#26431)) ;
#5508=EDGE_LOOP('',(#26432,#26433,#26434,#26435)) ;
#5509=EDGE_LOOP('',(#26436,#26437,#26438,#26439)) ;
#5510=EDGE_LOOP('',(#26440,#26441,#26442,#26443)) ;
#5511=EDGE_LOOP('',(#26444,#26445,#26446,#26447)) ;
#5512=EDGE_LOOP('',(#26448,#26449,#26450,#26451)) ;
#5513=EDGE_LOOP('',(#26452,#26453,#26454,#26455)) ;
#5514=EDGE_LOOP('',(#26456,#26457,#26458,#26459)) ;
#5515=EDGE_LOOP('',(#26460,#26461,#26462,#26463,#26464,#26465,#26466,#26467,
#26468,#26469,#26470,#26471,#26472,#26473,#26474,#26475,#26476,#26477,#26478,
#26479,#26480,#26481,#26482,#26483,#26484,#26485,#26486,#26487,#26488,#26489,
#26490,#26491,#26492,#26493,#26494,#26495,#26496,#26497,#26498,#26499)) ;
#5516=EDGE_LOOP('',(#26500,#26501,#26502,#26503)) ;
#5517=EDGE_LOOP('',(#26504,#26505,#26506,#26507,#26508,#26509)) ;
#5518=EDGE_LOOP('',(#26510,#26511,#26512,#26513)) ;
#5519=EDGE_LOOP('',(#26514,#26515,#26516,#26517)) ;
#5520=EDGE_LOOP('',(#26518,#26519,#26520,#26521)) ;
#5521=EDGE_LOOP('',(#26522,#26523,#26524,#26525)) ;
#5522=EDGE_LOOP('',(#26526,#26527,#26528,#26529)) ;
#5523=EDGE_LOOP('',(#26530,#26531,#26532,#26533)) ;
#5524=EDGE_LOOP('',(#26534,#26535,#26536,#26537)) ;
#5525=EDGE_LOOP('',(#26538,#26539,#26540,#26541)) ;
#5526=EDGE_LOOP('',(#26542,#26543,#26544,#26545,#26546,#26547)) ;
#5527=EDGE_LOOP('',(#26548,#26549,#26550,#26551)) ;
#5528=EDGE_LOOP('',(#26552,#26553,#26554,#26555)) ;
#5529=EDGE_LOOP('',(#26556,#26557,#26558,#26559)) ;
#5530=EDGE_LOOP('',(#26560,#26561,#26562,#26563)) ;
#5531=EDGE_LOOP('',(#26564,#26565,#26566,#26567)) ;
#5532=EDGE_LOOP('',(#26568,#26569,#26570,#26571)) ;
#5533=EDGE_LOOP('',(#26572,#26573,#26574,#26575)) ;
#5534=EDGE_LOOP('',(#26576,#26577,#26578,#26579)) ;
#5535=EDGE_LOOP('',(#26580,#26581,#26582,#26583)) ;
#5536=EDGE_LOOP('',(#26584,#26585,#26586,#26587)) ;
#5537=EDGE_LOOP('',(#26588,#26589,#26590,#26591,#26592)) ;
#5538=EDGE_LOOP('',(#26593,#26594,#26595,#26596,#26597,#26598)) ;
#5539=EDGE_LOOP('',(#26599,#26600,#26601,#26602,#26603,#26604)) ;
#5540=EDGE_LOOP('',(#26605,#26606,#26607,#26608,#26609,#26610)) ;
#5541=EDGE_LOOP('',(#26611,#26612,#26613,#26614,#26615,#26616)) ;
#5542=EDGE_LOOP('',(#26617,#26618,#26619,#26620,#26621,#26622)) ;
#5543=EDGE_LOOP('',(#26623,#26624,#26625,#26626,#26627,#26628)) ;
#5544=EDGE_LOOP('',(#26629,#26630,#26631,#26632,#26633,#26634)) ;
#5545=EDGE_LOOP('',(#26635,#26636,#26637,#26638,#26639,#26640)) ;
#5546=EDGE_LOOP('',(#26641,#26642,#26643,#26644,#26645,#26646)) ;
#5547=EDGE_LOOP('',(#26647,#26648,#26649,#26650,#26651,#26652)) ;
#5548=EDGE_LOOP('',(#26653,#26654,#26655,#26656,#26657,#26658)) ;
#5549=EDGE_LOOP('',(#26659,#26660,#26661,#26662,#26663,#26664)) ;
#5550=EDGE_LOOP('',(#26665,#26666,#26667,#26668,#26669,#26670)) ;
#5551=EDGE_LOOP('',(#26671,#26672,#26673,#26674,#26675,#26676)) ;
#5552=EDGE_LOOP('',(#26677,#26678,#26679,#26680,#26681,#26682)) ;
#5553=EDGE_LOOP('',(#26683,#26684,#26685,#26686,#26687,#26688)) ;
#5554=EDGE_LOOP('',(#26689,#26690,#26691,#26692)) ;
#5555=EDGE_LOOP('',(#26693,#26694,#26695,#26696,#26697,#26698,#26699,#26700,
#26701,#26702,#26703,#26704,#26705,#26706,#26707,#26708,#26709,#26710,#26711,
#26712,#26713,#26714,#26715,#26716,#26717,#26718,#26719,#26720,#26721,#26722,
#26723,#26724,#26725,#26726,#26727,#26728,#26729,#26730,#26731,#26732)) ;
#5556=EDGE_LOOP('',(#26733,#26734,#26735,#26736)) ;
#5557=EDGE_LOOP('',(#26737,#26738,#26739,#26740)) ;
#5558=EDGE_LOOP('',(#26741,#26742,#26743,#26744)) ;
#5559=EDGE_LOOP('',(#26745,#26746,#26747,#26748)) ;
#5560=EDGE_LOOP('',(#26749,#26750,#26751,#26752)) ;
#5561=EDGE_LOOP('',(#26753,#26754,#26755,#26756)) ;
#5562=EDGE_LOOP('',(#26757,#26758,#26759,#26760)) ;
#5563=EDGE_LOOP('',(#26761,#26762,#26763,#26764)) ;
#5564=EDGE_LOOP('',(#26765,#26766,#26767,#26768)) ;
#5565=EDGE_LOOP('',(#26769,#26770,#26771,#26772,#26773,#26774,#26775,#26776)) ;
#5566=EDGE_LOOP('',(#26777,#26778,#26779,#26780,#26781,#26782,#26783,#26784)) ;
#5567=EDGE_LOOP('',(#26785)) ;
#5568=EDGE_LOOP('',(#26786,#26787,#26788,#26789,#26790)) ;
#5569=EDGE_LOOP('',(#26791,#26792,#26793,#26794,#26795)) ;
#5570=EDGE_LOOP('',(#26796,#26797,#26798,#26799)) ;
#5571=EDGE_LOOP('',(#26800,#26801,#26802,#26803)) ;
#5572=EDGE_LOOP('',(#26804,#26805,#26806,#26807)) ;
#5573=EDGE_LOOP('',(#26808,#26809,#26810,#26811)) ;
#5574=EDGE_LOOP('',(#26812,#26813,#26814,#26815,#26816,#26817,#26818,#26819)) ;
#5575=EDGE_LOOP('',(#26820,#26821,#26822,#26823,#26824,#26825,#26826,#26827)) ;
#5576=EDGE_LOOP('',(#26828)) ;
#5577=EDGE_LOOP('',(#26829,#26830,#26831,#26832,#26833)) ;
#5578=EDGE_LOOP('',(#26834,#26835,#26836,#26837,#26838)) ;
#5579=EDGE_LOOP('',(#26839,#26840,#26841,#26842)) ;
#5580=EDGE_LOOP('',(#26843,#26844,#26845,#26846)) ;
#5581=EDGE_LOOP('',(#26847,#26848,#26849,#26850)) ;
#5582=EDGE_LOOP('',(#26851,#26852,#26853,#26854)) ;
#5583=EDGE_LOOP('',(#26855,#26856,#26857,#26858,#26859,#26860,#26861,#26862)) ;
#5584=EDGE_LOOP('',(#26863,#26864,#26865,#26866,#26867,#26868,#26869,#26870)) ;
#5585=EDGE_LOOP('',(#26871)) ;
#5586=EDGE_LOOP('',(#26872,#26873,#26874,#26875,#26876)) ;
#5587=EDGE_LOOP('',(#26877,#26878,#26879,#26880,#26881)) ;
#5588=EDGE_LOOP('',(#26882,#26883,#26884,#26885)) ;
#5589=EDGE_LOOP('',(#26886,#26887,#26888,#26889)) ;
#5590=EDGE_LOOP('',(#26890,#26891,#26892,#26893)) ;
#5591=EDGE_LOOP('',(#26894,#26895,#26896,#26897)) ;
#5592=EDGE_LOOP('',(#26898,#26899,#26900,#26901,#26902,#26903,#26904,#26905)) ;
#5593=EDGE_LOOP('',(#26906,#26907,#26908,#26909,#26910,#26911,#26912,#26913)) ;
#5594=EDGE_LOOP('',(#26914)) ;
#5595=EDGE_LOOP('',(#26915,#26916,#26917,#26918,#26919)) ;
#5596=EDGE_LOOP('',(#26920,#26921,#26922,#26923,#26924)) ;
#5597=EDGE_LOOP('',(#26925,#26926,#26927,#26928)) ;
#5598=EDGE_LOOP('',(#26929,#26930,#26931,#26932)) ;
#5599=EDGE_LOOP('',(#26933,#26934,#26935,#26936)) ;
#5600=EDGE_LOOP('',(#26937,#26938,#26939,#26940)) ;
#5601=EDGE_LOOP('',(#26941,#26942,#26943,#26944,#26945,#26946,#26947,#26948)) ;
#5602=EDGE_LOOP('',(#26949,#26950,#26951,#26952,#26953,#26954,#26955,#26956)) ;
#5603=EDGE_LOOP('',(#26957)) ;
#5604=EDGE_LOOP('',(#26958,#26959,#26960,#26961,#26962)) ;
#5605=EDGE_LOOP('',(#26963,#26964,#26965,#26966,#26967)) ;
#5606=EDGE_LOOP('',(#26968,#26969,#26970,#26971)) ;
#5607=EDGE_LOOP('',(#26972,#26973,#26974,#26975)) ;
#5608=EDGE_LOOP('',(#26976,#26977,#26978,#26979)) ;
#5609=EDGE_LOOP('',(#26980,#26981,#26982,#26983)) ;
#5610=EDGE_LOOP('',(#26984,#26985,#26986,#26987,#26988,#26989,#26990,#26991)) ;
#5611=EDGE_LOOP('',(#26992,#26993,#26994,#26995,#26996,#26997,#26998,#26999)) ;
#5612=EDGE_LOOP('',(#27000)) ;
#5613=EDGE_LOOP('',(#27001,#27002,#27003,#27004,#27005)) ;
#5614=EDGE_LOOP('',(#27006,#27007,#27008,#27009,#27010)) ;
#5615=EDGE_LOOP('',(#27011,#27012,#27013,#27014)) ;
#5616=EDGE_LOOP('',(#27015,#27016,#27017,#27018)) ;
#5617=EDGE_LOOP('',(#27019,#27020,#27021,#27022)) ;
#5618=EDGE_LOOP('',(#27023,#27024,#27025,#27026)) ;
#5619=EDGE_LOOP('',(#27027,#27028,#27029,#27030,#27031,#27032,#27033,#27034)) ;
#5620=EDGE_LOOP('',(#27035,#27036,#27037,#27038,#27039,#27040,#27041,#27042)) ;
#5621=EDGE_LOOP('',(#27043)) ;
#5622=EDGE_LOOP('',(#27044,#27045,#27046,#27047,#27048)) ;
#5623=EDGE_LOOP('',(#27049,#27050,#27051,#27052,#27053)) ;
#5624=EDGE_LOOP('',(#27054,#27055,#27056,#27057)) ;
#5625=EDGE_LOOP('',(#27058,#27059,#27060,#27061)) ;
#5626=EDGE_LOOP('',(#27062,#27063,#27064,#27065)) ;
#5627=EDGE_LOOP('',(#27066,#27067,#27068,#27069)) ;
#5628=EDGE_LOOP('',(#27070,#27071,#27072,#27073,#27074,#27075,#27076,#27077)) ;
#5629=EDGE_LOOP('',(#27078,#27079,#27080,#27081,#27082,#27083,#27084,#27085)) ;
#5630=EDGE_LOOP('',(#27086)) ;
#5631=EDGE_LOOP('',(#27087,#27088,#27089,#27090,#27091)) ;
#5632=EDGE_LOOP('',(#27092,#27093,#27094,#27095,#27096)) ;
#5633=EDGE_LOOP('',(#27097,#27098,#27099,#27100)) ;
#5634=EDGE_LOOP('',(#27101,#27102,#27103,#27104)) ;
#5635=EDGE_LOOP('',(#27105,#27106,#27107,#27108)) ;
#5636=EDGE_LOOP('',(#27109,#27110,#27111,#27112,#27113)) ;
#5637=EDGE_LOOP('',(#27114,#27115,#27116,#27117,#27118)) ;
#5638=EDGE_LOOP('',(#27119,#27120,#27121,#27122)) ;
#5639=EDGE_LOOP('',(#27123,#27124,#27125,#27126,#27127)) ;
#5640=EDGE_LOOP('',(#27128,#27129,#27130,#27131,#27132,#27133,#27134,#27135,
#27136,#27137,#27138,#27139,#27140,#27141,#27142,#27143,#27144,#27145,#27146,
#27147,#27148,#27149,#27150,#27151,#27152,#27153,#27154,#27155,#27156,#27157,
#27158,#27159,#27160,#27161,#27162,#27163,#27164,#27165,#27166,#27167,#27168,
#27169,#27170,#27171,#27172,#27173,#27174,#27175,#27176,#27177,#27178,#27179,
#27180,#27181,#27182,#27183,#27184,#27185,#27186,#27187,#27188,#27189,#27190,
#27191,#27192,#27193,#27194,#27195,#27196,#27197,#27198,#27199,#27200,#27201,
#27202,#27203)) ;
#5641=EDGE_LOOP('',(#27204,#27205,#27206,#27207)) ;
#5642=EDGE_LOOP('',(#27208,#27209,#27210,#27211)) ;
#5643=EDGE_LOOP('',(#27212,#27213,#27214,#27215)) ;
#5644=EDGE_LOOP('',(#27216,#27217,#27218,#27219)) ;
#5645=EDGE_LOOP('',(#27220,#27221,#27222,#27223)) ;
#5646=EDGE_LOOP('',(#27224,#27225,#27226,#27227)) ;
#5647=EDGE_LOOP('',(#27228,#27229,#27230,#27231)) ;
#5648=EDGE_LOOP('',(#27232,#27233,#27234,#27235)) ;
#5649=EDGE_LOOP('',(#27236,#27237,#27238,#27239)) ;
#5650=EDGE_LOOP('',(#27240,#27241,#27242,#27243)) ;
#5651=EDGE_LOOP('',(#27244,#27245,#27246,#27247)) ;
#5652=EDGE_LOOP('',(#27248,#27249,#27250,#27251)) ;
#5653=EDGE_LOOP('',(#27252,#27253,#27254,#27255)) ;
#5654=EDGE_LOOP('',(#27256,#27257,#27258,#27259)) ;
#5655=EDGE_LOOP('',(#27260,#27261,#27262,#27263)) ;
#5656=EDGE_LOOP('',(#27264,#27265,#27266,#27267)) ;
#5657=EDGE_LOOP('',(#27268,#27269,#27270,#27271)) ;
#5658=EDGE_LOOP('',(#27272,#27273,#27274,#27275)) ;
#5659=EDGE_LOOP('',(#27276,#27277,#27278,#27279)) ;
#5660=EDGE_LOOP('',(#27280,#27281,#27282,#27283)) ;
#5661=EDGE_LOOP('',(#27284,#27285,#27286,#27287)) ;
#5662=EDGE_LOOP('',(#27288,#27289,#27290,#27291)) ;
#5663=EDGE_LOOP('',(#27292,#27293,#27294,#27295)) ;
#5664=EDGE_LOOP('',(#27296,#27297,#27298,#27299)) ;
#5665=EDGE_LOOP('',(#27300,#27301,#27302,#27303)) ;
#5666=EDGE_LOOP('',(#27304,#27305,#27306,#27307)) ;
#5667=EDGE_LOOP('',(#27308,#27309,#27310,#27311)) ;
#5668=EDGE_LOOP('',(#27312,#27313,#27314,#27315)) ;
#5669=EDGE_LOOP('',(#27316,#27317,#27318,#27319)) ;
#5670=EDGE_LOOP('',(#27320,#27321,#27322,#27323)) ;
#5671=EDGE_LOOP('',(#27324,#27325,#27326,#27327)) ;
#5672=EDGE_LOOP('',(#27328,#27329,#27330,#27331)) ;
#5673=EDGE_LOOP('',(#27332,#27333,#27334,#27335)) ;
#5674=EDGE_LOOP('',(#27336,#27337,#27338,#27339)) ;
#5675=EDGE_LOOP('',(#27340,#27341,#27342,#27343)) ;
#5676=EDGE_LOOP('',(#27344,#27345,#27346,#27347)) ;
#5677=EDGE_LOOP('',(#27348,#27349,#27350,#27351)) ;
#5678=EDGE_LOOP('',(#27352,#27353,#27354,#27355)) ;
#5679=EDGE_LOOP('',(#27356,#27357,#27358,#27359)) ;
#5680=EDGE_LOOP('',(#27360,#27361,#27362,#27363)) ;
#7022=LINE('',#69343,#9341) ;
#7023=LINE('',#69345,#9342) ;
#7024=LINE('',#69347,#9343) ;
#7025=LINE('',#69348,#9344) ;
#7026=LINE('',#69351,#9345) ;
#7027=LINE('',#69353,#9346) ;
#7028=LINE('',#69354,#9347) ;
#7029=LINE('',#69357,#9348) ;
#7030=LINE('',#69359,#9349) ;
#7031=LINE('',#69360,#9350) ;
#7032=LINE('',#69362,#9351) ;
#7033=LINE('',#69366,#9352) ;
#7034=LINE('',#69368,#9353) ;
#7035=LINE('',#69370,#9354) ;
#7036=LINE('',#69371,#9355) ;
#7037=LINE('',#69374,#9356) ;
#7038=LINE('',#69376,#9357) ;
#7039=LINE('',#69377,#9358) ;
#7040=LINE('',#69380,#9359) ;
#7041=LINE('',#69382,#9360) ;
#7042=LINE('',#69383,#9361) ;
#7043=LINE('',#69385,#9362) ;
#7044=LINE('',#69389,#9363) ;
#7045=LINE('',#69391,#9364) ;
#7046=LINE('',#69393,#9365) ;
#7047=LINE('',#69394,#9366) ;
#7048=LINE('',#69397,#9367) ;
#7049=LINE('',#69399,#9368) ;
#7050=LINE('',#69400,#9369) ;
#7051=LINE('',#69403,#9370) ;
#7052=LINE('',#69405,#9371) ;
#7053=LINE('',#69406,#9372) ;
#7054=LINE('',#69408,#9373) ;
#7055=LINE('',#69412,#9374) ;
#7056=LINE('',#69414,#9375) ;
#7057=LINE('',#69416,#9376) ;
#7058=LINE('',#69417,#9377) ;
#7059=LINE('',#69420,#9378) ;
#7060=LINE('',#69422,#9379) ;
#7061=LINE('',#69423,#9380) ;
#7062=LINE('',#69426,#9381) ;
#7063=LINE('',#69428,#9382) ;
#7064=LINE('',#69429,#9383) ;
#7065=LINE('',#69431,#9384) ;
#7066=LINE('',#69435,#9385) ;
#7067=LINE('',#69437,#9386) ;
#7068=LINE('',#69439,#9387) ;
#7069=LINE('',#69440,#9388) ;
#7070=LINE('',#69443,#9389) ;
#7071=LINE('',#69445,#9390) ;
#7072=LINE('',#69446,#9391) ;
#7073=LINE('',#69449,#9392) ;
#7074=LINE('',#69451,#9393) ;
#7075=LINE('',#69452,#9394) ;
#7076=LINE('',#69454,#9395) ;
#7077=LINE('',#69458,#9396) ;
#7078=LINE('',#69460,#9397) ;
#7079=LINE('',#69462,#9398) ;
#7080=LINE('',#69463,#9399) ;
#7081=LINE('',#69466,#9400) ;
#7082=LINE('',#69468,#9401) ;
#7083=LINE('',#69469,#9402) ;
#7084=LINE('',#69472,#9403) ;
#7085=LINE('',#69474,#9404) ;
#7086=LINE('',#69475,#9405) ;
#7087=LINE('',#69477,#9406) ;
#7088=LINE('',#69481,#9407) ;
#7089=LINE('',#69483,#9408) ;
#7090=LINE('',#69485,#9409) ;
#7091=LINE('',#69486,#9410) ;
#7092=LINE('',#69489,#9411) ;
#7093=LINE('',#69491,#9412) ;
#7094=LINE('',#69492,#9413) ;
#7095=LINE('',#69495,#9414) ;
#7096=LINE('',#69497,#9415) ;
#7097=LINE('',#69498,#9416) ;
#7098=LINE('',#69500,#9417) ;
#7099=LINE('',#69504,#9418) ;
#7100=LINE('',#69506,#9419) ;
#7101=LINE('',#69508,#9420) ;
#7102=LINE('',#69509,#9421) ;
#7103=LINE('',#69512,#9422) ;
#7104=LINE('',#69514,#9423) ;
#7105=LINE('',#69515,#9424) ;
#7106=LINE('',#69518,#9425) ;
#7107=LINE('',#69520,#9426) ;
#7108=LINE('',#69521,#9427) ;
#7109=LINE('',#69523,#9428) ;
#7110=LINE('',#69527,#9429) ;
#7111=LINE('',#69529,#9430) ;
#7112=LINE('',#69531,#9431) ;
#7113=LINE('',#69532,#9432) ;
#7114=LINE('',#69535,#9433) ;
#7115=LINE('',#69537,#9434) ;
#7116=LINE('',#69538,#9435) ;
#7117=LINE('',#69541,#9436) ;
#7118=LINE('',#69543,#9437) ;
#7119=LINE('',#69544,#9438) ;
#7120=LINE('',#69546,#9439) ;
#7121=LINE('',#69548,#9440) ;
#7122=LINE('',#69549,#9441) ;
#7123=LINE('',#69550,#9442) ;
#7124=LINE('',#69551,#9443) ;
#7125=LINE('',#69552,#9444) ;
#7126=LINE('',#69553,#9445) ;
#7127=LINE('',#69555,#9446) ;
#7128=LINE('',#69557,#9447) ;
#7129=LINE('',#69559,#9448) ;
#7130=LINE('',#69561,#9449) ;
#7131=LINE('',#69563,#9450) ;
#7132=LINE('',#69565,#9451) ;
#7133=LINE('',#69567,#9452) ;
#7134=LINE('',#69569,#9453) ;
#7135=LINE('',#69571,#9454) ;
#7136=LINE('',#69573,#9455) ;
#7137=LINE('',#69575,#9456) ;
#7138=LINE('',#69577,#9457) ;
#7139=LINE('',#69579,#9458) ;
#7140=LINE('',#69581,#9459) ;
#7141=LINE('',#69583,#9460) ;
#7142=LINE('',#69585,#9461) ;
#7143=LINE('',#69587,#9462) ;
#7144=LINE('',#69589,#9463) ;
#7145=LINE('',#69591,#9464) ;
#7146=LINE('',#69593,#9465) ;
#7147=LINE('',#69595,#9466) ;
#7148=LINE('',#69597,#9467) ;
#7149=LINE('',#69599,#9468) ;
#7150=LINE('',#69601,#9469) ;
#7151=LINE('',#69603,#9470) ;
#7152=LINE('',#69605,#9471) ;
#7153=LINE('',#69607,#9472) ;
#7154=LINE('',#69609,#9473) ;
#7155=LINE('',#69611,#9474) ;
#7156=LINE('',#69613,#9475) ;
#7157=LINE('',#69615,#9476) ;
#7158=LINE('',#69617,#9477) ;
#7159=LINE('',#69619,#9478) ;
#7160=LINE('',#69621,#9479) ;
#7161=LINE('',#69623,#9480) ;
#7162=LINE('',#69625,#9481) ;
#7163=LINE('',#69627,#9482) ;
#7164=LINE('',#69629,#9483) ;
#7165=LINE('',#69631,#9484) ;
#7166=LINE('',#69633,#9485) ;
#7167=LINE('',#69634,#9486) ;
#7168=LINE('',#69635,#9487) ;
#7169=LINE('',#69636,#9488) ;
#7170=LINE('',#69646,#9489) ;
#7171=LINE('',#69650,#9490) ;
#7172=LINE('',#69652,#9491) ;
#7173=LINE('',#69654,#9492) ;
#7174=LINE('',#69655,#9493) ;
#7175=LINE('',#69658,#9494) ;
#7176=LINE('',#69662,#9495) ;
#7177=LINE('',#69666,#9496) ;
#7178=LINE('',#69670,#9497) ;
#7179=LINE('',#69681,#9498) ;
#7180=LINE('',#69685,#9499) ;
#7181=LINE('',#69687,#9500) ;
#7182=LINE('',#69689,#9501) ;
#7183=LINE('',#69690,#9502) ;
#7184=LINE('',#69693,#9503) ;
#7185=LINE('',#69697,#9504) ;
#7186=LINE('',#69701,#9505) ;
#7187=LINE('',#69705,#9506) ;
#7188=LINE('',#69716,#9507) ;
#7189=LINE('',#69720,#9508) ;
#7190=LINE('',#69722,#9509) ;
#7191=LINE('',#69724,#9510) ;
#7192=LINE('',#69725,#9511) ;
#7193=LINE('',#69728,#9512) ;
#7194=LINE('',#69732,#9513) ;
#7195=LINE('',#69736,#9514) ;
#7196=LINE('',#69740,#9515) ;
#7197=LINE('',#69751,#9516) ;
#7198=LINE('',#69755,#9517) ;
#7199=LINE('',#69757,#9518) ;
#7200=LINE('',#69759,#9519) ;
#7201=LINE('',#69760,#9520) ;
#7202=LINE('',#69763,#9521) ;
#7203=LINE('',#69767,#9522) ;
#7204=LINE('',#69771,#9523) ;
#7205=LINE('',#69775,#9524) ;
#7206=LINE('',#69786,#9525) ;
#7207=LINE('',#69790,#9526) ;
#7208=LINE('',#69792,#9527) ;
#7209=LINE('',#69794,#9528) ;
#7210=LINE('',#69795,#9529) ;
#7211=LINE('',#69798,#9530) ;
#7212=LINE('',#69802,#9531) ;
#7213=LINE('',#69806,#9532) ;
#7214=LINE('',#69810,#9533) ;
#7215=LINE('',#69821,#9534) ;
#7216=LINE('',#69825,#9535) ;
#7217=LINE('',#69827,#9536) ;
#7218=LINE('',#69829,#9537) ;
#7219=LINE('',#69830,#9538) ;
#7220=LINE('',#69833,#9539) ;
#7221=LINE('',#69837,#9540) ;
#7222=LINE('',#69841,#9541) ;
#7223=LINE('',#69845,#9542) ;
#7224=LINE('',#69856,#9543) ;
#7225=LINE('',#69860,#9544) ;
#7226=LINE('',#69862,#9545) ;
#7227=LINE('',#69864,#9546) ;
#7228=LINE('',#69865,#9547) ;
#7229=LINE('',#69868,#9548) ;
#7230=LINE('',#69872,#9549) ;
#7231=LINE('',#69876,#9550) ;
#7232=LINE('',#69880,#9551) ;
#7233=LINE('',#69891,#9552) ;
#7234=LINE('',#69895,#9553) ;
#7235=LINE('',#69897,#9554) ;
#7236=LINE('',#69899,#9555) ;
#7237=LINE('',#69900,#9556) ;
#7238=LINE('',#69903,#9557) ;
#7239=LINE('',#69907,#9558) ;
#7240=LINE('',#69911,#9559) ;
#7241=LINE('',#69915,#9560) ;
#7242=LINE('',#69926,#9561) ;
#7243=LINE('',#69928,#9562) ;
#7244=LINE('',#69930,#9563) ;
#7245=LINE('',#69931,#9564) ;
#7246=LINE('',#69934,#9565) ;
#7247=LINE('',#69938,#9566) ;
#7248=LINE('',#69942,#9567) ;
#7249=LINE('',#69946,#9568) ;
#7250=LINE('',#69951,#9569) ;
#7251=LINE('',#69980,#9570) ;
#7252=LINE('',#69989,#9571) ;
#7253=LINE('',#69997,#9572) ;
#7254=LINE('',#70005,#9573) ;
#7255=LINE('',#70010,#9574) ;
#7256=LINE('',#70013,#9575) ;
#7257=LINE('',#70016,#9576) ;
#7258=LINE('',#70020,#9577) ;
#7259=LINE('',#70022,#9578) ;
#7260=LINE('',#70024,#9579) ;
#7261=LINE('',#70026,#9580) ;
#7262=LINE('',#70028,#9581) ;
#7263=LINE('',#70032,#9582) ;
#7264=LINE('',#70036,#9583) ;
#7265=LINE('',#70037,#9584) ;
#7266=LINE('',#70042,#9585) ;
#7267=LINE('',#70051,#9586) ;
#7268=LINE('',#70059,#9587) ;
#7269=LINE('',#70067,#9588) ;
#7270=LINE('',#70072,#9589) ;
#7271=LINE('',#70075,#9590) ;
#7272=LINE('',#70078,#9591) ;
#7273=LINE('',#70082,#9592) ;
#7274=LINE('',#70084,#9593) ;
#7275=LINE('',#70086,#9594) ;
#7276=LINE('',#70088,#9595) ;
#7277=LINE('',#70090,#9596) ;
#7278=LINE('',#70094,#9597) ;
#7279=LINE('',#70098,#9598) ;
#7280=LINE('',#70099,#9599) ;
#7281=LINE('',#70104,#9600) ;
#7282=LINE('',#70113,#9601) ;
#7283=LINE('',#70121,#9602) ;
#7284=LINE('',#70129,#9603) ;
#7285=LINE('',#70134,#9604) ;
#7286=LINE('',#70137,#9605) ;
#7287=LINE('',#70140,#9606) ;
#7288=LINE('',#70144,#9607) ;
#7289=LINE('',#70146,#9608) ;
#7290=LINE('',#70148,#9609) ;
#7291=LINE('',#70150,#9610) ;
#7292=LINE('',#70152,#9611) ;
#7293=LINE('',#70156,#9612) ;
#7294=LINE('',#70160,#9613) ;
#7295=LINE('',#70161,#9614) ;
#7296=LINE('',#70166,#9615) ;
#7297=LINE('',#70175,#9616) ;
#7298=LINE('',#70183,#9617) ;
#7299=LINE('',#70191,#9618) ;
#7300=LINE('',#70196,#9619) ;
#7301=LINE('',#70199,#9620) ;
#7302=LINE('',#70202,#9621) ;
#7303=LINE('',#70206,#9622) ;
#7304=LINE('',#70208,#9623) ;
#7305=LINE('',#70210,#9624) ;
#7306=LINE('',#70212,#9625) ;
#7307=LINE('',#70214,#9626) ;
#7308=LINE('',#70218,#9627) ;
#7309=LINE('',#70222,#9628) ;
#7310=LINE('',#70223,#9629) ;
#7311=LINE('',#70228,#9630) ;
#7312=LINE('',#70237,#9631) ;
#7313=LINE('',#70245,#9632) ;
#7314=LINE('',#70253,#9633) ;
#7315=LINE('',#70258,#9634) ;
#7316=LINE('',#70261,#9635) ;
#7317=LINE('',#70264,#9636) ;
#7318=LINE('',#70268,#9637) ;
#7319=LINE('',#70270,#9638) ;
#7320=LINE('',#70272,#9639) ;
#7321=LINE('',#70274,#9640) ;
#7322=LINE('',#70276,#9641) ;
#7323=LINE('',#70280,#9642) ;
#7324=LINE('',#70284,#9643) ;
#7325=LINE('',#70285,#9644) ;
#7326=LINE('',#70290,#9645) ;
#7327=LINE('',#70299,#9646) ;
#7328=LINE('',#70307,#9647) ;
#7329=LINE('',#70315,#9648) ;
#7330=LINE('',#70320,#9649) ;
#7331=LINE('',#70323,#9650) ;
#7332=LINE('',#70326,#9651) ;
#7333=LINE('',#70330,#9652) ;
#7334=LINE('',#70332,#9653) ;
#7335=LINE('',#70334,#9654) ;
#7336=LINE('',#70336,#9655) ;
#7337=LINE('',#70338,#9656) ;
#7338=LINE('',#70342,#9657) ;
#7339=LINE('',#70346,#9658) ;
#7340=LINE('',#70347,#9659) ;
#7341=LINE('',#70352,#9660) ;
#7342=LINE('',#70361,#9661) ;
#7343=LINE('',#70369,#9662) ;
#7344=LINE('',#70377,#9663) ;
#7345=LINE('',#70382,#9664) ;
#7346=LINE('',#70385,#9665) ;
#7347=LINE('',#70388,#9666) ;
#7348=LINE('',#70392,#9667) ;
#7349=LINE('',#70394,#9668) ;
#7350=LINE('',#70396,#9669) ;
#7351=LINE('',#70398,#9670) ;
#7352=LINE('',#70400,#9671) ;
#7353=LINE('',#70404,#9672) ;
#7354=LINE('',#70408,#9673) ;
#7355=LINE('',#70409,#9674) ;
#7356=LINE('',#70414,#9675) ;
#7357=LINE('',#70423,#9676) ;
#7358=LINE('',#70431,#9677) ;
#7359=LINE('',#70439,#9678) ;
#7360=LINE('',#70444,#9679) ;
#7361=LINE('',#70447,#9680) ;
#7362=LINE('',#70450,#9681) ;
#7363=LINE('',#70454,#9682) ;
#7364=LINE('',#70456,#9683) ;
#7365=LINE('',#70458,#9684) ;
#7366=LINE('',#70460,#9685) ;
#7367=LINE('',#70462,#9686) ;
#7368=LINE('',#70466,#9687) ;
#7369=LINE('',#70470,#9688) ;
#7370=LINE('',#70471,#9689) ;
#7371=LINE('',#70476,#9690) ;
#7372=LINE('',#70485,#9691) ;
#7373=LINE('',#70493,#9692) ;
#7374=LINE('',#70501,#9693) ;
#7375=LINE('',#70506,#9694) ;
#7376=LINE('',#70509,#9695) ;
#7377=LINE('',#70513,#9696) ;
#7378=LINE('',#70515,#9697) ;
#7379=LINE('',#70517,#9698) ;
#7380=LINE('',#70520,#9699) ;
#7381=LINE('',#70524,#9700) ;
#7382=LINE('',#70525,#9701) ;
#7383=LINE('',#70528,#9702) ;
#7384=LINE('',#70532,#9703) ;
#7385=LINE('',#70533,#9704) ;
#7386=LINE('',#70539,#9705) ;
#7387=LINE('',#70542,#9706) ;
#7388=LINE('',#70553,#9707) ;
#7389=LINE('',#70554,#9708) ;
#7390=LINE('',#70565,#9709) ;
#7391=LINE('',#70566,#9710) ;
#7392=LINE('',#70577,#9711) ;
#7393=LINE('',#70578,#9712) ;
#7394=LINE('',#70584,#9713) ;
#7395=LINE('',#70587,#9714) ;
#7396=LINE('',#70590,#9715) ;
#7397=LINE('',#70591,#9716) ;
#7398=LINE('',#70594,#9717) ;
#7399=LINE('',#70598,#9718) ;
#7400=LINE('',#70599,#9719) ;
#7401=LINE('',#70605,#9720) ;
#7402=LINE('',#70608,#9721) ;
#7403=LINE('',#70619,#9722) ;
#7404=LINE('',#70620,#9723) ;
#7405=LINE('',#70631,#9724) ;
#7406=LINE('',#70632,#9725) ;
#7407=LINE('',#70643,#9726) ;
#7408=LINE('',#70644,#9727) ;
#7409=LINE('',#70650,#9728) ;
#7410=LINE('',#70653,#9729) ;
#7411=LINE('',#70656,#9730) ;
#7412=LINE('',#70657,#9731) ;
#7413=LINE('',#70660,#9732) ;
#7414=LINE('',#70664,#9733) ;
#7415=LINE('',#70665,#9734) ;
#7416=LINE('',#70671,#9735) ;
#7417=LINE('',#70674,#9736) ;
#7418=LINE('',#70685,#9737) ;
#7419=LINE('',#70686,#9738) ;
#7420=LINE('',#70697,#9739) ;
#7421=LINE('',#70698,#9740) ;
#7422=LINE('',#70709,#9741) ;
#7423=LINE('',#70710,#9742) ;
#7424=LINE('',#70716,#9743) ;
#7425=LINE('',#70719,#9744) ;
#7426=LINE('',#70722,#9745) ;
#7427=LINE('',#70723,#9746) ;
#7428=LINE('',#70726,#9747) ;
#7429=LINE('',#70730,#9748) ;
#7430=LINE('',#70731,#9749) ;
#7431=LINE('',#70737,#9750) ;
#7432=LINE('',#70740,#9751) ;
#7433=LINE('',#70751,#9752) ;
#7434=LINE('',#70752,#9753) ;
#7435=LINE('',#70763,#9754) ;
#7436=LINE('',#70764,#9755) ;
#7437=LINE('',#70775,#9756) ;
#7438=LINE('',#70776,#9757) ;
#7439=LINE('',#70782,#9758) ;
#7440=LINE('',#70785,#9759) ;
#7441=LINE('',#70788,#9760) ;
#7442=LINE('',#70789,#9761) ;
#7443=LINE('',#70792,#9762) ;
#7444=LINE('',#70796,#9763) ;
#7445=LINE('',#70797,#9764) ;
#7446=LINE('',#70803,#9765) ;
#7447=LINE('',#70806,#9766) ;
#7448=LINE('',#70817,#9767) ;
#7449=LINE('',#70818,#9768) ;
#7450=LINE('',#70829,#9769) ;
#7451=LINE('',#70830,#9770) ;
#7452=LINE('',#70841,#9771) ;
#7453=LINE('',#70842,#9772) ;
#7454=LINE('',#70848,#9773) ;
#7455=LINE('',#70851,#9774) ;
#7456=LINE('',#70854,#9775) ;
#7457=LINE('',#70855,#9776) ;
#7458=LINE('',#70858,#9777) ;
#7459=LINE('',#70862,#9778) ;
#7460=LINE('',#70863,#9779) ;
#7461=LINE('',#70869,#9780) ;
#7462=LINE('',#70872,#9781) ;
#7463=LINE('',#70883,#9782) ;
#7464=LINE('',#70884,#9783) ;
#7465=LINE('',#70895,#9784) ;
#7466=LINE('',#70896,#9785) ;
#7467=LINE('',#70907,#9786) ;
#7468=LINE('',#70908,#9787) ;
#7469=LINE('',#70914,#9788) ;
#7470=LINE('',#70917,#9789) ;
#7471=LINE('',#70920,#9790) ;
#7472=LINE('',#70921,#9791) ;
#7473=LINE('',#70924,#9792) ;
#7474=LINE('',#70928,#9793) ;
#7475=LINE('',#70929,#9794) ;
#7476=LINE('',#70935,#9795) ;
#7477=LINE('',#70938,#9796) ;
#7478=LINE('',#70949,#9797) ;
#7479=LINE('',#70950,#9798) ;
#7480=LINE('',#70961,#9799) ;
#7481=LINE('',#70962,#9800) ;
#7482=LINE('',#70973,#9801) ;
#7483=LINE('',#70974,#9802) ;
#7484=LINE('',#70980,#9803) ;
#7485=LINE('',#70983,#9804) ;
#7486=LINE('',#70986,#9805) ;
#7487=LINE('',#70987,#9806) ;
#7488=LINE('',#70990,#9807) ;
#7489=LINE('',#70994,#9808) ;
#7490=LINE('',#70995,#9809) ;
#7491=LINE('',#71001,#9810) ;
#7492=LINE('',#71004,#9811) ;
#7493=LINE('',#71015,#9812) ;
#7494=LINE('',#71016,#9813) ;
#7495=LINE('',#71027,#9814) ;
#7496=LINE('',#71028,#9815) ;
#7497=LINE('',#71039,#9816) ;
#7498=LINE('',#71040,#9817) ;
#7499=LINE('',#71046,#9818) ;
#7500=LINE('',#71049,#9819) ;
#7501=LINE('',#71052,#9820) ;
#7502=LINE('',#71053,#9821) ;
#7503=LINE('',#71056,#9822) ;
#7504=LINE('',#71060,#9823) ;
#7505=LINE('',#71061,#9824) ;
#7506=LINE('',#71067,#9825) ;
#7507=LINE('',#71070,#9826) ;
#7508=LINE('',#71081,#9827) ;
#7509=LINE('',#71082,#9828) ;
#7510=LINE('',#71093,#9829) ;
#7511=LINE('',#71094,#9830) ;
#7512=LINE('',#71103,#9831) ;
#7513=LINE('',#71109,#9832) ;
#7514=LINE('',#71112,#9833) ;
#7515=LINE('',#71115,#9834) ;
#7516=LINE('',#71118,#9835) ;
#7517=LINE('',#71120,#9836) ;
#7518=LINE('',#71122,#9837) ;
#7519=LINE('',#71125,#9838) ;
#7520=LINE('',#71128,#9839) ;
#7521=LINE('',#71132,#9840) ;
#7522=LINE('',#71133,#9841) ;
#7523=LINE('',#71139,#9842) ;
#7524=LINE('',#71142,#9843) ;
#7525=LINE('',#71153,#9844) ;
#7526=LINE('',#71154,#9845) ;
#7527=LINE('',#71165,#9846) ;
#7528=LINE('',#71166,#9847) ;
#7529=LINE('',#71175,#9848) ;
#7530=LINE('',#71181,#9849) ;
#7531=LINE('',#71184,#9850) ;
#7532=LINE('',#71187,#9851) ;
#7533=LINE('',#71190,#9852) ;
#7534=LINE('',#71192,#9853) ;
#7535=LINE('',#71194,#9854) ;
#7536=LINE('',#71197,#9855) ;
#7537=LINE('',#71200,#9856) ;
#7538=LINE('',#71204,#9857) ;
#7539=LINE('',#71205,#9858) ;
#7540=LINE('',#71211,#9859) ;
#7541=LINE('',#71214,#9860) ;
#7542=LINE('',#71225,#9861) ;
#7543=LINE('',#71226,#9862) ;
#7544=LINE('',#71237,#9863) ;
#7545=LINE('',#71238,#9864) ;
#7546=LINE('',#71247,#9865) ;
#7547=LINE('',#71253,#9866) ;
#7548=LINE('',#71256,#9867) ;
#7549=LINE('',#71259,#9868) ;
#7550=LINE('',#71262,#9869) ;
#7551=LINE('',#71264,#9870) ;
#7552=LINE('',#71266,#9871) ;
#7553=LINE('',#71269,#9872) ;
#7554=LINE('',#71272,#9873) ;
#7555=LINE('',#71276,#9874) ;
#7556=LINE('',#71277,#9875) ;
#7557=LINE('',#71283,#9876) ;
#7558=LINE('',#71286,#9877) ;
#7559=LINE('',#71297,#9878) ;
#7560=LINE('',#71298,#9879) ;
#7561=LINE('',#71309,#9880) ;
#7562=LINE('',#71310,#9881) ;
#7563=LINE('',#71319,#9882) ;
#7564=LINE('',#71325,#9883) ;
#7565=LINE('',#71328,#9884) ;
#7566=LINE('',#71331,#9885) ;
#7567=LINE('',#71334,#9886) ;
#7568=LINE('',#71336,#9887) ;
#7569=LINE('',#71338,#9888) ;
#7570=LINE('',#71341,#9889) ;
#7571=LINE('',#71344,#9890) ;
#7572=LINE('',#71348,#9891) ;
#7573=LINE('',#71349,#9892) ;
#7574=LINE('',#71355,#9893) ;
#7575=LINE('',#71358,#9894) ;
#7576=LINE('',#71369,#9895) ;
#7577=LINE('',#71370,#9896) ;
#7578=LINE('',#71381,#9897) ;
#7579=LINE('',#71382,#9898) ;
#7580=LINE('',#71391,#9899) ;
#7581=LINE('',#71397,#9900) ;
#7582=LINE('',#71400,#9901) ;
#7583=LINE('',#71403,#9902) ;
#7584=LINE('',#71406,#9903) ;
#7585=LINE('',#71408,#9904) ;
#7586=LINE('',#71410,#9905) ;
#7587=LINE('',#71413,#9906) ;
#7588=LINE('',#71416,#9907) ;
#7589=LINE('',#71420,#9908) ;
#7590=LINE('',#71421,#9909) ;
#7591=LINE('',#71427,#9910) ;
#7592=LINE('',#71430,#9911) ;
#7593=LINE('',#71441,#9912) ;
#7594=LINE('',#71442,#9913) ;
#7595=LINE('',#71453,#9914) ;
#7596=LINE('',#71454,#9915) ;
#7597=LINE('',#71463,#9916) ;
#7598=LINE('',#71469,#9917) ;
#7599=LINE('',#71472,#9918) ;
#7600=LINE('',#71475,#9919) ;
#7601=LINE('',#71478,#9920) ;
#7602=LINE('',#71480,#9921) ;
#7603=LINE('',#71482,#9922) ;
#7604=LINE('',#71485,#9923) ;
#7605=LINE('',#71488,#9924) ;
#7606=LINE('',#71492,#9925) ;
#7607=LINE('',#71493,#9926) ;
#7608=LINE('',#71499,#9927) ;
#7609=LINE('',#71502,#9928) ;
#7610=LINE('',#71513,#9929) ;
#7611=LINE('',#71514,#9930) ;
#7612=LINE('',#71525,#9931) ;
#7613=LINE('',#71526,#9932) ;
#7614=LINE('',#71535,#9933) ;
#7615=LINE('',#71541,#9934) ;
#7616=LINE('',#71544,#9935) ;
#7617=LINE('',#71547,#9936) ;
#7618=LINE('',#71550,#9937) ;
#7619=LINE('',#71552,#9938) ;
#7620=LINE('',#71554,#9939) ;
#7621=LINE('',#71557,#9940) ;
#7622=LINE('',#71560,#9941) ;
#7623=LINE('',#71564,#9942) ;
#7624=LINE('',#71565,#9943) ;
#7625=LINE('',#71571,#9944) ;
#7626=LINE('',#71574,#9945) ;
#7627=LINE('',#71585,#9946) ;
#7628=LINE('',#71586,#9947) ;
#7629=LINE('',#71597,#9948) ;
#7630=LINE('',#71598,#9949) ;
#7631=LINE('',#71607,#9950) ;
#7632=LINE('',#71613,#9951) ;
#7633=LINE('',#71616,#9952) ;
#7634=LINE('',#71619,#9953) ;
#7635=LINE('',#71622,#9954) ;
#7636=LINE('',#71624,#9955) ;
#7637=LINE('',#71626,#9956) ;
#7638=LINE('',#71629,#9957) ;
#7639=LINE('',#71632,#9958) ;
#7640=LINE('',#71636,#9959) ;
#7641=LINE('',#71637,#9960) ;
#7642=LINE('',#71643,#9961) ;
#7643=LINE('',#71646,#9962) ;
#7644=LINE('',#71657,#9963) ;
#7645=LINE('',#71658,#9964) ;
#7646=LINE('',#71669,#9965) ;
#7647=LINE('',#71670,#9966) ;
#7648=LINE('',#71681,#9967) ;
#7649=LINE('',#71682,#9968) ;
#7650=LINE('',#71688,#9969) ;
#7651=LINE('',#71691,#9970) ;
#7652=LINE('',#71694,#9971) ;
#7653=LINE('',#71695,#9972) ;
#7654=LINE('',#71698,#9973) ;
#7655=LINE('',#71702,#9974) ;
#7656=LINE('',#71703,#9975) ;
#7657=LINE('',#71707,#9976) ;
#7658=LINE('',#71709,#9977) ;
#7659=LINE('',#71711,#9978) ;
#7660=LINE('',#71712,#9979) ;
#7661=LINE('',#71715,#9980) ;
#7662=LINE('',#71719,#9981) ;
#7663=LINE('',#71723,#9982) ;
#7664=LINE('',#71727,#9983) ;
#7665=LINE('',#71735,#9984) ;
#7666=LINE('',#71744,#9985) ;
#7667=LINE('',#71752,#9986) ;
#7668=LINE('',#71762,#9987) ;
#7669=LINE('',#71765,#9988) ;
#7670=LINE('',#71768,#9989) ;
#7671=LINE('',#71770,#9990) ;
#7672=LINE('',#71773,#9991) ;
#7673=LINE('',#71775,#9992) ;
#7674=LINE('',#71778,#9993) ;
#7675=LINE('',#71781,#9994) ;
#7676=LINE('',#71785,#9995) ;
#7677=LINE('',#71786,#9996) ;
#7678=LINE('',#71789,#9997) ;
#7679=LINE('',#71790,#9998) ;
#7680=LINE('',#71797,#9999) ;
#7681=LINE('',#71798,#10000) ;
#7682=LINE('',#71802,#10001) ;
#7683=LINE('',#71805,#10002) ;
#7684=LINE('',#71808,#10003) ;
#7685=LINE('',#71819,#10004) ;
#7686=LINE('',#71827,#10005) ;
#7687=LINE('',#71839,#10006) ;
#7688=LINE('',#71842,#10007) ;
#7689=LINE('',#71849,#10008) ;
#7690=LINE('',#71851,#10009) ;
#7691=LINE('',#71852,#10010) ;
#7692=LINE('',#71856,#10011) ;
#7693=LINE('',#71858,#10012) ;
#7694=LINE('',#71863,#10013) ;
#7695=LINE('',#71873,#10014) ;
#7696=LINE('',#71875,#10015) ;
#7697=LINE('',#71877,#10016) ;
#7698=LINE('',#71878,#10017) ;
#7699=LINE('',#71901,#10018) ;
#7700=LINE('',#71904,#10019) ;
#7701=LINE('',#71912,#10020) ;
#7702=LINE('',#71924,#10021) ;
#7703=LINE('',#71927,#10022) ;
#7704=LINE('',#71934,#10023) ;
#7705=LINE('',#71936,#10024) ;
#7706=LINE('',#71937,#10025) ;
#7707=LINE('',#71941,#10026) ;
#7708=LINE('',#71943,#10027) ;
#7709=LINE('',#71949,#10028) ;
#7710=LINE('',#71960,#10029) ;
#7711=LINE('',#71962,#10030) ;
#7712=LINE('',#71964,#10031) ;
#7713=LINE('',#71965,#10032) ;
#7714=LINE('',#71978,#10033) ;
#7715=LINE('',#71982,#10034) ;
#7716=LINE('',#71995,#10035) ;
#7717=LINE('',#71998,#10036) ;
#7718=LINE('',#72006,#10037) ;
#7719=LINE('',#72018,#10038) ;
#7720=LINE('',#72021,#10039) ;
#7721=LINE('',#72028,#10040) ;
#7722=LINE('',#72030,#10041) ;
#7723=LINE('',#72031,#10042) ;
#7724=LINE('',#72035,#10043) ;
#7725=LINE('',#72037,#10044) ;
#7726=LINE('',#72043,#10045) ;
#7727=LINE('',#72054,#10046) ;
#7728=LINE('',#72056,#10047) ;
#7729=LINE('',#72058,#10048) ;
#7730=LINE('',#72059,#10049) ;
#7731=LINE('',#72072,#10050) ;
#7732=LINE('',#72076,#10051) ;
#7733=LINE('',#72089,#10052) ;
#7734=LINE('',#72092,#10053) ;
#7735=LINE('',#72100,#10054) ;
#7736=LINE('',#72112,#10055) ;
#7737=LINE('',#72115,#10056) ;
#7738=LINE('',#72122,#10057) ;
#7739=LINE('',#72124,#10058) ;
#7740=LINE('',#72125,#10059) ;
#7741=LINE('',#72129,#10060) ;
#7742=LINE('',#72131,#10061) ;
#7743=LINE('',#72137,#10062) ;
#7744=LINE('',#72148,#10063) ;
#7745=LINE('',#72150,#10064) ;
#7746=LINE('',#72152,#10065) ;
#7747=LINE('',#72153,#10066) ;
#7748=LINE('',#72166,#10067) ;
#7749=LINE('',#72170,#10068) ;
#7750=LINE('',#72183,#10069) ;
#7751=LINE('',#72186,#10070) ;
#7752=LINE('',#72194,#10071) ;
#7753=LINE('',#72206,#10072) ;
#7754=LINE('',#72209,#10073) ;
#7755=LINE('',#72216,#10074) ;
#7756=LINE('',#72218,#10075) ;
#7757=LINE('',#72219,#10076) ;
#7758=LINE('',#72223,#10077) ;
#7759=LINE('',#72225,#10078) ;
#7760=LINE('',#72231,#10079) ;
#7761=LINE('',#72242,#10080) ;
#7762=LINE('',#72244,#10081) ;
#7763=LINE('',#72246,#10082) ;
#7764=LINE('',#72247,#10083) ;
#7765=LINE('',#72260,#10084) ;
#7766=LINE('',#72264,#10085) ;
#7767=LINE('',#72277,#10086) ;
#7768=LINE('',#72280,#10087) ;
#7769=LINE('',#72288,#10088) ;
#7770=LINE('',#72300,#10089) ;
#7771=LINE('',#72303,#10090) ;
#7772=LINE('',#72310,#10091) ;
#7773=LINE('',#72312,#10092) ;
#7774=LINE('',#72313,#10093) ;
#7775=LINE('',#72317,#10094) ;
#7776=LINE('',#72319,#10095) ;
#7777=LINE('',#72325,#10096) ;
#7778=LINE('',#72336,#10097) ;
#7779=LINE('',#72338,#10098) ;
#7780=LINE('',#72340,#10099) ;
#7781=LINE('',#72341,#10100) ;
#7782=LINE('',#72354,#10101) ;
#7783=LINE('',#72358,#10102) ;
#7784=LINE('',#72371,#10103) ;
#7785=LINE('',#72374,#10104) ;
#7786=LINE('',#72382,#10105) ;
#7787=LINE('',#72394,#10106) ;
#7788=LINE('',#72397,#10107) ;
#7789=LINE('',#72404,#10108) ;
#7790=LINE('',#72406,#10109) ;
#7791=LINE('',#72407,#10110) ;
#7792=LINE('',#72411,#10111) ;
#7793=LINE('',#72413,#10112) ;
#7794=LINE('',#72419,#10113) ;
#7795=LINE('',#72430,#10114) ;
#7796=LINE('',#72432,#10115) ;
#7797=LINE('',#72434,#10116) ;
#7798=LINE('',#72435,#10117) ;
#7799=LINE('',#72448,#10118) ;
#7800=LINE('',#72452,#10119) ;
#7801=LINE('',#72465,#10120) ;
#7802=LINE('',#72468,#10121) ;
#7803=LINE('',#72476,#10122) ;
#7804=LINE('',#72488,#10123) ;
#7805=LINE('',#72491,#10124) ;
#7806=LINE('',#72498,#10125) ;
#7807=LINE('',#72500,#10126) ;
#7808=LINE('',#72501,#10127) ;
#7809=LINE('',#72505,#10128) ;
#7810=LINE('',#72507,#10129) ;
#7811=LINE('',#72513,#10130) ;
#7812=LINE('',#72524,#10131) ;
#7813=LINE('',#72526,#10132) ;
#7814=LINE('',#72528,#10133) ;
#7815=LINE('',#72529,#10134) ;
#7816=LINE('',#72542,#10135) ;
#7817=LINE('',#72546,#10136) ;
#7818=LINE('',#72559,#10137) ;
#7819=LINE('',#72562,#10138) ;
#7820=LINE('',#72570,#10139) ;
#7821=LINE('',#72582,#10140) ;
#7822=LINE('',#72585,#10141) ;
#7823=LINE('',#72592,#10142) ;
#7824=LINE('',#72594,#10143) ;
#7825=LINE('',#72595,#10144) ;
#7826=LINE('',#72599,#10145) ;
#7827=LINE('',#72601,#10146) ;
#7828=LINE('',#72607,#10147) ;
#7829=LINE('',#72618,#10148) ;
#7830=LINE('',#72620,#10149) ;
#7831=LINE('',#72622,#10150) ;
#7832=LINE('',#72623,#10151) ;
#7833=LINE('',#72636,#10152) ;
#7834=LINE('',#72640,#10153) ;
#7835=LINE('',#72648,#10154) ;
#7836=LINE('',#72649,#10155) ;
#7837=LINE('',#72651,#10156) ;
#7838=LINE('',#72652,#10157) ;
#7839=LINE('',#72654,#10158) ;
#7840=LINE('',#72655,#10159) ;
#7841=LINE('',#72657,#10160) ;
#7842=LINE('',#72658,#10161) ;
#7843=LINE('',#72660,#10162) ;
#7844=LINE('',#72661,#10163) ;
#7845=LINE('',#72663,#10164) ;
#7846=LINE('',#72664,#10165) ;
#7847=LINE('',#72666,#10166) ;
#7848=LINE('',#72667,#10167) ;
#7849=LINE('',#72669,#10168) ;
#7850=LINE('',#72670,#10169) ;
#7851=LINE('',#72672,#10170) ;
#7852=LINE('',#72673,#10171) ;
#7853=LINE('',#72675,#10172) ;
#7854=LINE('',#72677,#10173) ;
#7855=LINE('',#72679,#10174) ;
#7856=LINE('',#72681,#10175) ;
#7857=LINE('',#72683,#10176) ;
#7858=LINE('',#72685,#10177) ;
#7859=LINE('',#72687,#10178) ;
#7860=LINE('',#72689,#10179) ;
#7861=LINE('',#72691,#10180) ;
#7862=LINE('',#72693,#10181) ;
#7863=LINE('',#72695,#10182) ;
#7864=LINE('',#72697,#10183) ;
#7865=LINE('',#72699,#10184) ;
#7866=LINE('',#72701,#10185) ;
#7867=LINE('',#72703,#10186) ;
#7868=LINE('',#72705,#10187) ;
#7869=LINE('',#72707,#10188) ;
#7870=LINE('',#72709,#10189) ;
#7871=LINE('',#72713,#10190) ;
#7872=LINE('',#72715,#10191) ;
#7873=LINE('',#72717,#10192) ;
#7874=LINE('',#72719,#10193) ;
#7875=LINE('',#72721,#10194) ;
#7876=LINE('',#72723,#10195) ;
#7877=LINE('',#72725,#10196) ;
#7878=LINE('',#72727,#10197) ;
#7879=LINE('',#72729,#10198) ;
#7880=LINE('',#72731,#10199) ;
#7881=LINE('',#72733,#10200) ;
#7882=LINE('',#72735,#10201) ;
#7883=LINE('',#72737,#10202) ;
#7884=LINE('',#72739,#10203) ;
#7885=LINE('',#72741,#10204) ;
#7886=LINE('',#72743,#10205) ;
#7887=LINE('',#72745,#10206) ;
#7888=LINE('',#72747,#10207) ;
#7889=LINE('',#72749,#10208) ;
#7890=LINE('',#72751,#10209) ;
#7891=LINE('',#72753,#10210) ;
#7892=LINE('',#72755,#10211) ;
#7893=LINE('',#72757,#10212) ;
#7894=LINE('',#72759,#10213) ;
#7895=LINE('',#72761,#10214) ;
#7896=LINE('',#72763,#10215) ;
#7897=LINE('',#72765,#10216) ;
#7898=LINE('',#72767,#10217) ;
#7899=LINE('',#72769,#10218) ;
#7900=LINE('',#72771,#10219) ;
#7901=LINE('',#72773,#10220) ;
#7902=LINE('',#72775,#10221) ;
#7903=LINE('',#72777,#10222) ;
#7904=LINE('',#72779,#10223) ;
#7905=LINE('',#72781,#10224) ;
#7906=LINE('',#72783,#10225) ;
#7907=LINE('',#72785,#10226) ;
#7908=LINE('',#72787,#10227) ;
#7909=LINE('',#72789,#10228) ;
#7910=LINE('',#72790,#10229) ;
#7911=LINE('',#72795,#10230) ;
#7912=LINE('',#72798,#10231) ;
#7913=LINE('',#72800,#10232) ;
#7914=LINE('',#72801,#10233) ;
#7915=LINE('',#72805,#10234) ;
#7916=LINE('',#72812,#10235) ;
#7917=LINE('',#72818,#10236) ;
#7918=LINE('',#72823,#10237) ;
#7919=LINE('',#72829,#10238) ;
#7920=LINE('',#72835,#10239) ;
#7921=LINE('',#72842,#10240) ;
#7922=LINE('',#72847,#10241) ;
#7923=LINE('',#72854,#10242) ;
#7924=LINE('',#72855,#10243) ;
#7925=LINE('',#72856,#10244) ;
#7926=LINE('',#72859,#10245) ;
#7927=LINE('',#72862,#10246) ;
#7928=LINE('',#72866,#10247) ;
#7929=LINE('',#72868,#10248) ;
#7930=LINE('',#72870,#10249) ;
#7931=LINE('',#72871,#10250) ;
#7932=LINE('',#72875,#10251) ;
#7933=LINE('',#72877,#10252) ;
#7934=LINE('',#72879,#10253) ;
#7935=LINE('',#72880,#10254) ;
#7936=LINE('',#72884,#10255) ;
#7937=LINE('',#72886,#10256) ;
#7938=LINE('',#72888,#10257) ;
#7939=LINE('',#72889,#10258) ;
#7940=LINE('',#72893,#10259) ;
#7941=LINE('',#72895,#10260) ;
#7942=LINE('',#72897,#10261) ;
#7943=LINE('',#72898,#10262) ;
#7944=LINE('',#72902,#10263) ;
#7945=LINE('',#72904,#10264) ;
#7946=LINE('',#72906,#10265) ;
#7947=LINE('',#72907,#10266) ;
#7948=LINE('',#72911,#10267) ;
#7949=LINE('',#72913,#10268) ;
#7950=LINE('',#72915,#10269) ;
#7951=LINE('',#72916,#10270) ;
#7952=LINE('',#72920,#10271) ;
#7953=LINE('',#72922,#10272) ;
#7954=LINE('',#72924,#10273) ;
#7955=LINE('',#72925,#10274) ;
#7956=LINE('',#72929,#10275) ;
#7957=LINE('',#72931,#10276) ;
#7958=LINE('',#72933,#10277) ;
#7959=LINE('',#72934,#10278) ;
#7960=LINE('',#72936,#10279) ;
#7961=LINE('',#72937,#10280) ;
#7962=LINE('',#72939,#10281) ;
#7963=LINE('',#72941,#10282) ;
#7964=LINE('',#72942,#10283) ;
#7965=LINE('',#72945,#10284) ;
#7966=LINE('',#72946,#10285) ;
#7967=LINE('',#72947,#10286) ;
#7968=LINE('',#72949,#10287) ;
#7969=LINE('',#72951,#10288) ;
#7970=LINE('',#72952,#10289) ;
#7971=LINE('',#72955,#10290) ;
#7972=LINE('',#72956,#10291) ;
#7973=LINE('',#72957,#10292) ;
#7974=LINE('',#72959,#10293) ;
#7975=LINE('',#72961,#10294) ;
#7976=LINE('',#72962,#10295) ;
#7977=LINE('',#72965,#10296) ;
#7978=LINE('',#72966,#10297) ;
#7979=LINE('',#72967,#10298) ;
#7980=LINE('',#72969,#10299) ;
#7981=LINE('',#72971,#10300) ;
#7982=LINE('',#72972,#10301) ;
#7983=LINE('',#72975,#10302) ;
#7984=LINE('',#72976,#10303) ;
#7985=LINE('',#72977,#10304) ;
#7986=LINE('',#72979,#10305) ;
#7987=LINE('',#72981,#10306) ;
#7988=LINE('',#72982,#10307) ;
#7989=LINE('',#72985,#10308) ;
#7990=LINE('',#72986,#10309) ;
#7991=LINE('',#72987,#10310) ;
#7992=LINE('',#72989,#10311) ;
#7993=LINE('',#72991,#10312) ;
#7994=LINE('',#72992,#10313) ;
#7995=LINE('',#72995,#10314) ;
#7996=LINE('',#72996,#10315) ;
#7997=LINE('',#72997,#10316) ;
#7998=LINE('',#72999,#10317) ;
#7999=LINE('',#73001,#10318) ;
#8000=LINE('',#73002,#10319) ;
#8001=LINE('',#73005,#10320) ;
#8002=LINE('',#73006,#10321) ;
#8003=LINE('',#73007,#10322) ;
#8004=LINE('',#73009,#10323) ;
#8005=LINE('',#73011,#10324) ;
#8006=LINE('',#73012,#10325) ;
#8007=LINE('',#73015,#10326) ;
#8008=LINE('',#73016,#10327) ;
#8009=LINE('',#73017,#10328) ;
#8010=LINE('',#73020,#10329) ;
#8011=LINE('',#73022,#10330) ;
#8012=LINE('',#73024,#10331) ;
#8013=LINE('',#73026,#10332) ;
#8014=LINE('',#73028,#10333) ;
#8015=LINE('',#73030,#10334) ;
#8016=LINE('',#73032,#10335) ;
#8017=LINE('',#73034,#10336) ;
#8018=LINE('',#73036,#10337) ;
#8019=LINE('',#73049,#10338) ;
#8020=LINE('',#73053,#10339) ;
#8021=LINE('',#73067,#10340) ;
#8022=LINE('',#73071,#10341) ;
#8023=LINE('',#73085,#10342) ;
#8024=LINE('',#73089,#10343) ;
#8025=LINE('',#73103,#10344) ;
#8026=LINE('',#73107,#10345) ;
#8027=LINE('',#73121,#10346) ;
#8028=LINE('',#73125,#10347) ;
#8029=LINE('',#73139,#10348) ;
#8030=LINE('',#73143,#10349) ;
#8031=LINE('',#73157,#10350) ;
#8032=LINE('',#73161,#10351) ;
#8033=LINE('',#73175,#10352) ;
#8034=LINE('',#73179,#10353) ;
#8035=LINE('',#73190,#10354) ;
#8036=LINE('',#73194,#10355) ;
#8037=LINE('',#73197,#10356) ;
#8038=LINE('',#73199,#10357) ;
#8039=LINE('',#73201,#10358) ;
#8040=LINE('',#73205,#10359) ;
#8041=LINE('',#73207,#10360) ;
#8042=LINE('',#73209,#10361) ;
#8043=LINE('',#73213,#10362) ;
#8044=LINE('',#73215,#10363) ;
#8045=LINE('',#73217,#10364) ;
#8046=LINE('',#73221,#10365) ;
#8047=LINE('',#73223,#10366) ;
#8048=LINE('',#73225,#10367) ;
#8049=LINE('',#73229,#10368) ;
#8050=LINE('',#73231,#10369) ;
#8051=LINE('',#73233,#10370) ;
#8052=LINE('',#73237,#10371) ;
#8053=LINE('',#73239,#10372) ;
#8054=LINE('',#73241,#10373) ;
#8055=LINE('',#73245,#10374) ;
#8056=LINE('',#73247,#10375) ;
#8057=LINE('',#73249,#10376) ;
#8058=LINE('',#73253,#10377) ;
#8059=LINE('',#73255,#10378) ;
#8060=LINE('',#73257,#10379) ;
#9341=VECTOR('',#39208,10.) ;
#9342=VECTOR('',#39209,10.) ;
#9343=VECTOR('',#39210,10.) ;
#9344=VECTOR('',#39211,10.) ;
#9345=VECTOR('',#39214,10.) ;
#9346=VECTOR('',#39215,10.) ;
#9347=VECTOR('',#39216,10.) ;
#9348=VECTOR('',#39219,10.) ;
#9349=VECTOR('',#39220,10.) ;
#9350=VECTOR('',#39221,10.) ;
#9351=VECTOR('',#39224,10.) ;
#9352=VECTOR('',#39227,10.) ;
#9353=VECTOR('',#39228,10.) ;
#9354=VECTOR('',#39229,10.) ;
#9355=VECTOR('',#39230,10.) ;
#9356=VECTOR('',#39233,10.) ;
#9357=VECTOR('',#39234,10.) ;
#9358=VECTOR('',#39235,10.) ;
#9359=VECTOR('',#39238,10.) ;
#9360=VECTOR('',#39239,10.) ;
#9361=VECTOR('',#39240,10.) ;
#9362=VECTOR('',#39243,10.) ;
#9363=VECTOR('',#39246,10.) ;
#9364=VECTOR('',#39247,10.) ;
#9365=VECTOR('',#39248,10.) ;
#9366=VECTOR('',#39249,10.) ;
#9367=VECTOR('',#39252,10.) ;
#9368=VECTOR('',#39253,10.) ;
#9369=VECTOR('',#39254,10.) ;
#9370=VECTOR('',#39257,10.) ;
#9371=VECTOR('',#39258,10.) ;
#9372=VECTOR('',#39259,10.) ;
#9373=VECTOR('',#39262,10.) ;
#9374=VECTOR('',#39265,10.) ;
#9375=VECTOR('',#39266,10.) ;
#9376=VECTOR('',#39267,10.) ;
#9377=VECTOR('',#39268,10.) ;
#9378=VECTOR('',#39271,10.) ;
#9379=VECTOR('',#39272,10.) ;
#9380=VECTOR('',#39273,10.) ;
#9381=VECTOR('',#39276,10.) ;
#9382=VECTOR('',#39277,10.) ;
#9383=VECTOR('',#39278,10.) ;
#9384=VECTOR('',#39281,10.) ;
#9385=VECTOR('',#39284,10.) ;
#9386=VECTOR('',#39285,10.) ;
#9387=VECTOR('',#39286,10.) ;
#9388=VECTOR('',#39287,10.) ;
#9389=VECTOR('',#39290,10.) ;
#9390=VECTOR('',#39291,10.) ;
#9391=VECTOR('',#39292,10.) ;
#9392=VECTOR('',#39295,10.) ;
#9393=VECTOR('',#39296,10.) ;
#9394=VECTOR('',#39297,10.) ;
#9395=VECTOR('',#39300,10.) ;
#9396=VECTOR('',#39303,10.) ;
#9397=VECTOR('',#39304,10.) ;
#9398=VECTOR('',#39305,10.) ;
#9399=VECTOR('',#39306,10.) ;
#9400=VECTOR('',#39309,10.) ;
#9401=VECTOR('',#39310,10.) ;
#9402=VECTOR('',#39311,10.) ;
#9403=VECTOR('',#39314,10.) ;
#9404=VECTOR('',#39315,10.) ;
#9405=VECTOR('',#39316,10.) ;
#9406=VECTOR('',#39319,10.) ;
#9407=VECTOR('',#39322,10.) ;
#9408=VECTOR('',#39323,10.) ;
#9409=VECTOR('',#39324,10.) ;
#9410=VECTOR('',#39325,10.) ;
#9411=VECTOR('',#39328,10.) ;
#9412=VECTOR('',#39329,10.) ;
#9413=VECTOR('',#39330,10.) ;
#9414=VECTOR('',#39333,10.) ;
#9415=VECTOR('',#39334,10.) ;
#9416=VECTOR('',#39335,10.) ;
#9417=VECTOR('',#39338,10.) ;
#9418=VECTOR('',#39341,10.) ;
#9419=VECTOR('',#39342,10.) ;
#9420=VECTOR('',#39343,10.) ;
#9421=VECTOR('',#39344,10.) ;
#9422=VECTOR('',#39347,10.) ;
#9423=VECTOR('',#39348,10.) ;
#9424=VECTOR('',#39349,10.) ;
#9425=VECTOR('',#39352,10.) ;
#9426=VECTOR('',#39353,10.) ;
#9427=VECTOR('',#39354,10.) ;
#9428=VECTOR('',#39357,10.) ;
#9429=VECTOR('',#39360,10.) ;
#9430=VECTOR('',#39361,10.) ;
#9431=VECTOR('',#39362,10.) ;
#9432=VECTOR('',#39363,10.) ;
#9433=VECTOR('',#39366,10.) ;
#9434=VECTOR('',#39367,10.) ;
#9435=VECTOR('',#39368,10.) ;
#9436=VECTOR('',#39371,10.) ;
#9437=VECTOR('',#39372,10.) ;
#9438=VECTOR('',#39373,10.) ;
#9439=VECTOR('',#39376,10.) ;
#9440=VECTOR('',#39379,10.) ;
#9441=VECTOR('',#39380,10.) ;
#9442=VECTOR('',#39381,10.) ;
#9443=VECTOR('',#39382,10.) ;
#9444=VECTOR('',#39383,10.) ;
#9445=VECTOR('',#39384,10.) ;
#9446=VECTOR('',#39385,10.) ;
#9447=VECTOR('',#39386,13.3) ;
#9448=VECTOR('',#39387,87.07601714263) ;
#9449=VECTOR('',#39388,10.) ;
#9450=VECTOR('',#39389,10.) ;
#9451=VECTOR('',#39390,10.) ;
#9452=VECTOR('',#39391,87.07601714263) ;
#9453=VECTOR('',#39392,10.) ;
#9454=VECTOR('',#39393,10.) ;
#9455=VECTOR('',#39394,10.) ;
#9456=VECTOR('',#39395,87.07601714263) ;
#9457=VECTOR('',#39396,10.) ;
#9458=VECTOR('',#39397,10.) ;
#9459=VECTOR('',#39398,10.) ;
#9460=VECTOR('',#39399,87.07601714263) ;
#9461=VECTOR('',#39400,10.) ;
#9462=VECTOR('',#39401,10.) ;
#9463=VECTOR('',#39402,10.) ;
#9464=VECTOR('',#39403,87.07601714263) ;
#9465=VECTOR('',#39404,10.) ;
#9466=VECTOR('',#39405,10.) ;
#9467=VECTOR('',#39406,10.) ;
#9468=VECTOR('',#39407,87.07601714263) ;
#9469=VECTOR('',#39408,10.) ;
#9470=VECTOR('',#39409,10.) ;
#9471=VECTOR('',#39410,10.) ;
#9472=VECTOR('',#39411,87.07601714263) ;
#9473=VECTOR('',#39412,10.) ;
#9474=VECTOR('',#39413,10.) ;
#9475=VECTOR('',#39414,10.) ;
#9476=VECTOR('',#39415,87.07601714263) ;
#9477=VECTOR('',#39416,10.) ;
#9478=VECTOR('',#39417,10.) ;
#9479=VECTOR('',#39418,10.) ;
#9480=VECTOR('',#39419,87.07601714263) ;
#9481=VECTOR('',#39420,10.) ;
#9482=VECTOR('',#39421,10.) ;
#9483=VECTOR('',#39422,10.) ;
#9484=VECTOR('',#39423,87.07601714263) ;
#9485=VECTOR('',#39424,10.) ;
#9486=VECTOR('',#39425,10.) ;
#9487=VECTOR('',#39426,10.) ;
#9488=VECTOR('',#39427,10.) ;
#9489=VECTOR('',#39440,1.5) ;
#9490=VECTOR('',#39443,10.) ;
#9491=VECTOR('',#39444,10.) ;
#9492=VECTOR('',#39445,10.) ;
#9493=VECTOR('',#39446,10.) ;
#9494=VECTOR('',#39447,10.) ;
#9495=VECTOR('',#39450,10.) ;
#9496=VECTOR('',#39453,10.) ;
#9497=VECTOR('',#39456,10.) ;
#9498=VECTOR('',#39471,1.5) ;
#9499=VECTOR('',#39474,10.) ;
#9500=VECTOR('',#39475,10.) ;
#9501=VECTOR('',#39476,10.) ;
#9502=VECTOR('',#39477,10.) ;
#9503=VECTOR('',#39478,10.) ;
#9504=VECTOR('',#39481,10.) ;
#9505=VECTOR('',#39484,10.) ;
#9506=VECTOR('',#39487,10.) ;
#9507=VECTOR('',#39502,1.5) ;
#9508=VECTOR('',#39505,10.) ;
#9509=VECTOR('',#39506,10.) ;
#9510=VECTOR('',#39507,10.) ;
#9511=VECTOR('',#39508,10.) ;
#9512=VECTOR('',#39509,10.) ;
#9513=VECTOR('',#39512,10.) ;
#9514=VECTOR('',#39515,10.) ;
#9515=VECTOR('',#39518,10.) ;
#9516=VECTOR('',#39533,1.5) ;
#9517=VECTOR('',#39536,10.) ;
#9518=VECTOR('',#39537,10.) ;
#9519=VECTOR('',#39538,10.) ;
#9520=VECTOR('',#39539,10.) ;
#9521=VECTOR('',#39540,10.) ;
#9522=VECTOR('',#39543,10.) ;
#9523=VECTOR('',#39546,10.) ;
#9524=VECTOR('',#39549,10.) ;
#9525=VECTOR('',#39564,1.5) ;
#9526=VECTOR('',#39567,10.) ;
#9527=VECTOR('',#39568,10.) ;
#9528=VECTOR('',#39569,10.) ;
#9529=VECTOR('',#39570,10.) ;
#9530=VECTOR('',#39571,10.) ;
#9531=VECTOR('',#39574,10.) ;
#9532=VECTOR('',#39577,10.) ;
#9533=VECTOR('',#39580,10.) ;
#9534=VECTOR('',#39595,1.5) ;
#9535=VECTOR('',#39598,10.) ;
#9536=VECTOR('',#39599,10.) ;
#9537=VECTOR('',#39600,10.) ;
#9538=VECTOR('',#39601,10.) ;
#9539=VECTOR('',#39602,10.) ;
#9540=VECTOR('',#39605,10.) ;
#9541=VECTOR('',#39608,10.) ;
#9542=VECTOR('',#39611,10.) ;
#9543=VECTOR('',#39626,1.5) ;
#9544=VECTOR('',#39629,10.) ;
#9545=VECTOR('',#39630,10.) ;
#9546=VECTOR('',#39631,10.) ;
#9547=VECTOR('',#39632,10.) ;
#9548=VECTOR('',#39633,10.) ;
#9549=VECTOR('',#39636,10.) ;
#9550=VECTOR('',#39639,10.) ;
#9551=VECTOR('',#39642,10.) ;
#9552=VECTOR('',#39657,1.5) ;
#9553=VECTOR('',#39660,10.) ;
#9554=VECTOR('',#39661,10.) ;
#9555=VECTOR('',#39662,10.) ;
#9556=VECTOR('',#39663,10.) ;
#9557=VECTOR('',#39664,10.) ;
#9558=VECTOR('',#39667,10.) ;
#9559=VECTOR('',#39670,10.) ;
#9560=VECTOR('',#39673,10.) ;
#9561=VECTOR('',#39686,10.) ;
#9562=VECTOR('',#39687,10.) ;
#9563=VECTOR('',#39688,10.) ;
#9564=VECTOR('',#39689,10.) ;
#9565=VECTOR('',#39690,10.) ;
#9566=VECTOR('',#39693,10.) ;
#9567=VECTOR('',#39696,10.) ;
#9568=VECTOR('',#39699,10.) ;
#9569=VECTOR('',#39706,1.5) ;
#9570=VECTOR('',#39743,10.) ;
#9571=VECTOR('',#39756,10.) ;
#9572=VECTOR('',#39767,10.) ;
#9573=VECTOR('',#39778,10.) ;
#9574=VECTOR('',#39785,10.) ;
#9575=VECTOR('',#39788,10.) ;
#9576=VECTOR('',#39791,10.) ;
#9577=VECTOR('',#39794,10.) ;
#9578=VECTOR('',#39795,10.) ;
#9579=VECTOR('',#39796,10.) ;
#9580=VECTOR('',#39797,10.) ;
#9581=VECTOR('',#39798,10.) ;
#9582=VECTOR('',#39803,10.) ;
#9583=VECTOR('',#39808,10.) ;
#9584=VECTOR('',#39809,10.) ;
#9585=VECTOR('',#39814,10.) ;
#9586=VECTOR('',#39827,10.) ;
#9587=VECTOR('',#39838,10.) ;
#9588=VECTOR('',#39849,10.) ;
#9589=VECTOR('',#39856,10.) ;
#9590=VECTOR('',#39859,10.) ;
#9591=VECTOR('',#39862,10.) ;
#9592=VECTOR('',#39865,10.) ;
#9593=VECTOR('',#39866,10.) ;
#9594=VECTOR('',#39867,10.) ;
#9595=VECTOR('',#39868,10.) ;
#9596=VECTOR('',#39869,10.) ;
#9597=VECTOR('',#39874,10.) ;
#9598=VECTOR('',#39879,10.) ;
#9599=VECTOR('',#39880,10.) ;
#9600=VECTOR('',#39885,10.) ;
#9601=VECTOR('',#39898,10.) ;
#9602=VECTOR('',#39909,10.) ;
#9603=VECTOR('',#39920,10.) ;
#9604=VECTOR('',#39927,10.) ;
#9605=VECTOR('',#39930,10.) ;
#9606=VECTOR('',#39933,10.) ;
#9607=VECTOR('',#39936,10.) ;
#9608=VECTOR('',#39937,10.) ;
#9609=VECTOR('',#39938,10.) ;
#9610=VECTOR('',#39939,10.) ;
#9611=VECTOR('',#39940,10.) ;
#9612=VECTOR('',#39945,10.) ;
#9613=VECTOR('',#39950,10.) ;
#9614=VECTOR('',#39951,10.) ;
#9615=VECTOR('',#39956,10.) ;
#9616=VECTOR('',#39969,10.) ;
#9617=VECTOR('',#39980,10.) ;
#9618=VECTOR('',#39991,10.) ;
#9619=VECTOR('',#39998,10.) ;
#9620=VECTOR('',#40001,10.) ;
#9621=VECTOR('',#40004,10.) ;
#9622=VECTOR('',#40007,10.) ;
#9623=VECTOR('',#40008,10.) ;
#9624=VECTOR('',#40009,10.) ;
#9625=VECTOR('',#40010,10.) ;
#9626=VECTOR('',#40011,10.) ;
#9627=VECTOR('',#40016,10.) ;
#9628=VECTOR('',#40021,10.) ;
#9629=VECTOR('',#40022,10.) ;
#9630=VECTOR('',#40027,10.) ;
#9631=VECTOR('',#40040,10.) ;
#9632=VECTOR('',#40051,10.) ;
#9633=VECTOR('',#40062,10.) ;
#9634=VECTOR('',#40069,10.) ;
#9635=VECTOR('',#40072,10.) ;
#9636=VECTOR('',#40075,10.) ;
#9637=VECTOR('',#40078,10.) ;
#9638=VECTOR('',#40079,10.) ;
#9639=VECTOR('',#40080,10.) ;
#9640=VECTOR('',#40081,10.) ;
#9641=VECTOR('',#40082,10.) ;
#9642=VECTOR('',#40087,10.) ;
#9643=VECTOR('',#40092,10.) ;
#9644=VECTOR('',#40093,10.) ;
#9645=VECTOR('',#40098,10.) ;
#9646=VECTOR('',#40111,10.) ;
#9647=VECTOR('',#40122,10.) ;
#9648=VECTOR('',#40133,10.) ;
#9649=VECTOR('',#40140,10.) ;
#9650=VECTOR('',#40143,10.) ;
#9651=VECTOR('',#40146,10.) ;
#9652=VECTOR('',#40149,10.) ;
#9653=VECTOR('',#40150,10.) ;
#9654=VECTOR('',#40151,10.) ;
#9655=VECTOR('',#40152,10.) ;
#9656=VECTOR('',#40153,10.) ;
#9657=VECTOR('',#40158,10.) ;
#9658=VECTOR('',#40163,10.) ;
#9659=VECTOR('',#40164,10.) ;
#9660=VECTOR('',#40169,10.) ;
#9661=VECTOR('',#40182,10.) ;
#9662=VECTOR('',#40193,10.) ;
#9663=VECTOR('',#40204,10.) ;
#9664=VECTOR('',#40211,10.) ;
#9665=VECTOR('',#40214,10.) ;
#9666=VECTOR('',#40217,10.) ;
#9667=VECTOR('',#40220,10.) ;
#9668=VECTOR('',#40221,10.) ;
#9669=VECTOR('',#40222,10.) ;
#9670=VECTOR('',#40223,10.) ;
#9671=VECTOR('',#40224,10.) ;
#9672=VECTOR('',#40229,10.) ;
#9673=VECTOR('',#40234,10.) ;
#9674=VECTOR('',#40235,10.) ;
#9675=VECTOR('',#40240,10.) ;
#9676=VECTOR('',#40253,10.) ;
#9677=VECTOR('',#40264,10.) ;
#9678=VECTOR('',#40275,10.) ;
#9679=VECTOR('',#40282,10.) ;
#9680=VECTOR('',#40285,10.) ;
#9681=VECTOR('',#40288,10.) ;
#9682=VECTOR('',#40291,10.) ;
#9683=VECTOR('',#40292,10.) ;
#9684=VECTOR('',#40293,10.) ;
#9685=VECTOR('',#40294,10.) ;
#9686=VECTOR('',#40295,10.) ;
#9687=VECTOR('',#40300,10.) ;
#9688=VECTOR('',#40305,10.) ;
#9689=VECTOR('',#40306,10.) ;
#9690=VECTOR('',#40311,10.) ;
#9691=VECTOR('',#40324,10.) ;
#9692=VECTOR('',#40335,10.) ;
#9693=VECTOR('',#40346,10.) ;
#9694=VECTOR('',#40353,10.) ;
#9695=VECTOR('',#40356,10.) ;
#9696=VECTOR('',#40359,10.) ;
#9697=VECTOR('',#40360,10.) ;
#9698=VECTOR('',#40361,10.) ;
#9699=VECTOR('',#40364,10.) ;
#9700=VECTOR('',#40367,10.) ;
#9701=VECTOR('',#40368,10.) ;
#9702=VECTOR('',#40371,10.) ;
#9703=VECTOR('',#40376,10.) ;
#9704=VECTOR('',#40377,10.) ;
#9705=VECTOR('',#40382,10.) ;
#9706=VECTOR('',#40385,10.) ;
#9707=VECTOR('',#40398,10.) ;
#9708=VECTOR('',#40399,10.) ;
#9709=VECTOR('',#40412,10.) ;
#9710=VECTOR('',#40413,10.) ;
#9711=VECTOR('',#40426,10.) ;
#9712=VECTOR('',#40427,10.) ;
#9713=VECTOR('',#40436,10.) ;
#9714=VECTOR('',#40439,10.) ;
#9715=VECTOR('',#40442,10.) ;
#9716=VECTOR('',#40443,10.) ;
#9717=VECTOR('',#40446,10.) ;
#9718=VECTOR('',#40451,10.) ;
#9719=VECTOR('',#40452,10.) ;
#9720=VECTOR('',#40457,10.) ;
#9721=VECTOR('',#40460,10.) ;
#9722=VECTOR('',#40473,10.) ;
#9723=VECTOR('',#40474,10.) ;
#9724=VECTOR('',#40487,10.) ;
#9725=VECTOR('',#40488,10.) ;
#9726=VECTOR('',#40501,10.) ;
#9727=VECTOR('',#40502,10.) ;
#9728=VECTOR('',#40511,10.) ;
#9729=VECTOR('',#40514,10.) ;
#9730=VECTOR('',#40517,10.) ;
#9731=VECTOR('',#40518,10.) ;
#9732=VECTOR('',#40521,10.) ;
#9733=VECTOR('',#40526,10.) ;
#9734=VECTOR('',#40527,10.) ;
#9735=VECTOR('',#40532,10.) ;
#9736=VECTOR('',#40535,10.) ;
#9737=VECTOR('',#40548,10.) ;
#9738=VECTOR('',#40549,10.) ;
#9739=VECTOR('',#40562,10.) ;
#9740=VECTOR('',#40563,10.) ;
#9741=VECTOR('',#40576,10.) ;
#9742=VECTOR('',#40577,10.) ;
#9743=VECTOR('',#40586,10.) ;
#9744=VECTOR('',#40589,10.) ;
#9745=VECTOR('',#40592,10.) ;
#9746=VECTOR('',#40593,10.) ;
#9747=VECTOR('',#40596,10.) ;
#9748=VECTOR('',#40601,10.) ;
#9749=VECTOR('',#40602,10.) ;
#9750=VECTOR('',#40607,10.) ;
#9751=VECTOR('',#40610,10.) ;
#9752=VECTOR('',#40623,10.) ;
#9753=VECTOR('',#40624,10.) ;
#9754=VECTOR('',#40637,10.) ;
#9755=VECTOR('',#40638,10.) ;
#9756=VECTOR('',#40651,10.) ;
#9757=VECTOR('',#40652,10.) ;
#9758=VECTOR('',#40661,10.) ;
#9759=VECTOR('',#40664,10.) ;
#9760=VECTOR('',#40667,10.) ;
#9761=VECTOR('',#40668,10.) ;
#9762=VECTOR('',#40671,10.) ;
#9763=VECTOR('',#40676,10.) ;
#9764=VECTOR('',#40677,10.) ;
#9765=VECTOR('',#40682,10.) ;
#9766=VECTOR('',#40685,10.) ;
#9767=VECTOR('',#40698,10.) ;
#9768=VECTOR('',#40699,10.) ;
#9769=VECTOR('',#40712,10.) ;
#9770=VECTOR('',#40713,10.) ;
#9771=VECTOR('',#40726,10.) ;
#9772=VECTOR('',#40727,10.) ;
#9773=VECTOR('',#40736,10.) ;
#9774=VECTOR('',#40739,10.) ;
#9775=VECTOR('',#40742,10.) ;
#9776=VECTOR('',#40743,10.) ;
#9777=VECTOR('',#40746,10.) ;
#9778=VECTOR('',#40751,10.) ;
#9779=VECTOR('',#40752,10.) ;
#9780=VECTOR('',#40757,10.) ;
#9781=VECTOR('',#40760,10.) ;
#9782=VECTOR('',#40773,10.) ;
#9783=VECTOR('',#40774,10.) ;
#9784=VECTOR('',#40787,10.) ;
#9785=VECTOR('',#40788,10.) ;
#9786=VECTOR('',#40801,10.) ;
#9787=VECTOR('',#40802,10.) ;
#9788=VECTOR('',#40811,10.) ;
#9789=VECTOR('',#40814,10.) ;
#9790=VECTOR('',#40817,10.) ;
#9791=VECTOR('',#40818,10.) ;
#9792=VECTOR('',#40821,10.) ;
#9793=VECTOR('',#40826,10.) ;
#9794=VECTOR('',#40827,10.) ;
#9795=VECTOR('',#40832,10.) ;
#9796=VECTOR('',#40835,10.) ;
#9797=VECTOR('',#40848,10.) ;
#9798=VECTOR('',#40849,10.) ;
#9799=VECTOR('',#40862,10.) ;
#9800=VECTOR('',#40863,10.) ;
#9801=VECTOR('',#40876,10.) ;
#9802=VECTOR('',#40877,10.) ;
#9803=VECTOR('',#40886,10.) ;
#9804=VECTOR('',#40889,10.) ;
#9805=VECTOR('',#40892,10.) ;
#9806=VECTOR('',#40893,10.) ;
#9807=VECTOR('',#40896,10.) ;
#9808=VECTOR('',#40901,10.) ;
#9809=VECTOR('',#40902,10.) ;
#9810=VECTOR('',#40907,10.) ;
#9811=VECTOR('',#40910,10.) ;
#9812=VECTOR('',#40923,10.) ;
#9813=VECTOR('',#40924,10.) ;
#9814=VECTOR('',#40937,10.) ;
#9815=VECTOR('',#40938,10.) ;
#9816=VECTOR('',#40951,10.) ;
#9817=VECTOR('',#40952,10.) ;
#9818=VECTOR('',#40961,10.) ;
#9819=VECTOR('',#40964,10.) ;
#9820=VECTOR('',#40967,10.) ;
#9821=VECTOR('',#40968,10.) ;
#9822=VECTOR('',#40971,10.) ;
#9823=VECTOR('',#40976,10.) ;
#9824=VECTOR('',#40977,10.) ;
#9825=VECTOR('',#40982,10.) ;
#9826=VECTOR('',#40985,10.) ;
#9827=VECTOR('',#40998,10.) ;
#9828=VECTOR('',#40999,10.) ;
#9829=VECTOR('',#41012,10.) ;
#9830=VECTOR('',#41013,10.) ;
#9831=VECTOR('',#41026,10.) ;
#9832=VECTOR('',#41035,10.) ;
#9833=VECTOR('',#41038,0.125) ;
#9834=VECTOR('',#41041,10.) ;
#9835=VECTOR('',#41044,10.) ;
#9836=VECTOR('',#41045,10.) ;
#9837=VECTOR('',#41046,10.) ;
#9838=VECTOR('',#41049,10.) ;
#9839=VECTOR('',#41052,10.) ;
#9840=VECTOR('',#41057,10.) ;
#9841=VECTOR('',#41058,10.) ;
#9842=VECTOR('',#41063,10.) ;
#9843=VECTOR('',#41066,10.) ;
#9844=VECTOR('',#41079,10.) ;
#9845=VECTOR('',#41080,10.) ;
#9846=VECTOR('',#41093,10.) ;
#9847=VECTOR('',#41094,10.) ;
#9848=VECTOR('',#41107,10.) ;
#9849=VECTOR('',#41116,10.) ;
#9850=VECTOR('',#41119,0.125) ;
#9851=VECTOR('',#41122,10.) ;
#9852=VECTOR('',#41125,10.) ;
#9853=VECTOR('',#41126,10.) ;
#9854=VECTOR('',#41127,10.) ;
#9855=VECTOR('',#41130,10.) ;
#9856=VECTOR('',#41133,10.) ;
#9857=VECTOR('',#41138,10.) ;
#9858=VECTOR('',#41139,10.) ;
#9859=VECTOR('',#41144,10.) ;
#9860=VECTOR('',#41147,10.) ;
#9861=VECTOR('',#41160,10.) ;
#9862=VECTOR('',#41161,10.) ;
#9863=VECTOR('',#41174,10.) ;
#9864=VECTOR('',#41175,10.) ;
#9865=VECTOR('',#41188,10.) ;
#9866=VECTOR('',#41197,10.) ;
#9867=VECTOR('',#41200,0.125) ;
#9868=VECTOR('',#41203,10.) ;
#9869=VECTOR('',#41206,10.) ;
#9870=VECTOR('',#41207,10.) ;
#9871=VECTOR('',#41208,10.) ;
#9872=VECTOR('',#41211,10.) ;
#9873=VECTOR('',#41214,10.) ;
#9874=VECTOR('',#41219,10.) ;
#9875=VECTOR('',#41220,10.) ;
#9876=VECTOR('',#41225,10.) ;
#9877=VECTOR('',#41228,10.) ;
#9878=VECTOR('',#41241,10.) ;
#9879=VECTOR('',#41242,10.) ;
#9880=VECTOR('',#41255,10.) ;
#9881=VECTOR('',#41256,10.) ;
#9882=VECTOR('',#41269,10.) ;
#9883=VECTOR('',#41278,10.) ;
#9884=VECTOR('',#41281,0.125) ;
#9885=VECTOR('',#41284,10.) ;
#9886=VECTOR('',#41287,10.) ;
#9887=VECTOR('',#41288,10.) ;
#9888=VECTOR('',#41289,10.) ;
#9889=VECTOR('',#41292,10.) ;
#9890=VECTOR('',#41295,10.) ;
#9891=VECTOR('',#41300,10.) ;
#9892=VECTOR('',#41301,10.) ;
#9893=VECTOR('',#41306,10.) ;
#9894=VECTOR('',#41309,10.) ;
#9895=VECTOR('',#41322,10.) ;
#9896=VECTOR('',#41323,10.) ;
#9897=VECTOR('',#41336,10.) ;
#9898=VECTOR('',#41337,10.) ;
#9899=VECTOR('',#41350,10.) ;
#9900=VECTOR('',#41359,10.) ;
#9901=VECTOR('',#41362,0.125) ;
#9902=VECTOR('',#41365,10.) ;
#9903=VECTOR('',#41368,10.) ;
#9904=VECTOR('',#41369,10.) ;
#9905=VECTOR('',#41370,10.) ;
#9906=VECTOR('',#41373,10.) ;
#9907=VECTOR('',#41376,10.) ;
#9908=VECTOR('',#41381,10.) ;
#9909=VECTOR('',#41382,10.) ;
#9910=VECTOR('',#41387,10.) ;
#9911=VECTOR('',#41390,10.) ;
#9912=VECTOR('',#41403,10.) ;
#9913=VECTOR('',#41404,10.) ;
#9914=VECTOR('',#41417,10.) ;
#9915=VECTOR('',#41418,10.) ;
#9916=VECTOR('',#41431,10.) ;
#9917=VECTOR('',#41440,10.) ;
#9918=VECTOR('',#41443,0.125) ;
#9919=VECTOR('',#41446,10.) ;
#9920=VECTOR('',#41449,10.) ;
#9921=VECTOR('',#41450,10.) ;
#9922=VECTOR('',#41451,10.) ;
#9923=VECTOR('',#41454,10.) ;
#9924=VECTOR('',#41457,10.) ;
#9925=VECTOR('',#41462,10.) ;
#9926=VECTOR('',#41463,10.) ;
#9927=VECTOR('',#41468,10.) ;
#9928=VECTOR('',#41471,10.) ;
#9929=VECTOR('',#41484,10.) ;
#9930=VECTOR('',#41485,10.) ;
#9931=VECTOR('',#41498,10.) ;
#9932=VECTOR('',#41499,10.) ;
#9933=VECTOR('',#41512,10.) ;
#9934=VECTOR('',#41521,10.) ;
#9935=VECTOR('',#41524,0.125) ;
#9936=VECTOR('',#41527,10.) ;
#9937=VECTOR('',#41530,10.) ;
#9938=VECTOR('',#41531,10.) ;
#9939=VECTOR('',#41532,10.) ;
#9940=VECTOR('',#41535,10.) ;
#9941=VECTOR('',#41538,10.) ;
#9942=VECTOR('',#41543,10.) ;
#9943=VECTOR('',#41544,10.) ;
#9944=VECTOR('',#41549,10.) ;
#9945=VECTOR('',#41552,10.) ;
#9946=VECTOR('',#41565,10.) ;
#9947=VECTOR('',#41566,10.) ;
#9948=VECTOR('',#41579,10.) ;
#9949=VECTOR('',#41580,10.) ;
#9950=VECTOR('',#41593,10.) ;
#9951=VECTOR('',#41602,10.) ;
#9952=VECTOR('',#41605,0.125) ;
#9953=VECTOR('',#41608,10.) ;
#9954=VECTOR('',#41611,10.) ;
#9955=VECTOR('',#41612,10.) ;
#9956=VECTOR('',#41613,10.) ;
#9957=VECTOR('',#41616,10.) ;
#9958=VECTOR('',#41619,10.) ;
#9959=VECTOR('',#41624,10.) ;
#9960=VECTOR('',#41625,10.) ;
#9961=VECTOR('',#41630,10.) ;
#9962=VECTOR('',#41633,10.) ;
#9963=VECTOR('',#41646,10.) ;
#9964=VECTOR('',#41647,10.) ;
#9965=VECTOR('',#41660,10.) ;
#9966=VECTOR('',#41661,10.) ;
#9967=VECTOR('',#41674,10.) ;
#9968=VECTOR('',#41675,10.) ;
#9969=VECTOR('',#41684,10.) ;
#9970=VECTOR('',#41687,10.) ;
#9971=VECTOR('',#41690,10.) ;
#9972=VECTOR('',#41691,10.) ;
#9973=VECTOR('',#41694,10.) ;
#9974=VECTOR('',#41699,10.) ;
#9975=VECTOR('',#41700,10.) ;
#9976=VECTOR('',#41703,10.) ;
#9977=VECTOR('',#41704,10.) ;
#9978=VECTOR('',#41705,10.) ;
#9979=VECTOR('',#41706,10.) ;
#9980=VECTOR('',#41707,10.) ;
#9981=VECTOR('',#41710,10.) ;
#9982=VECTOR('',#41713,10.) ;
#9983=VECTOR('',#41716,10.) ;
#9984=VECTOR('',#41725,10.) ;
#9985=VECTOR('',#41738,10.) ;
#9986=VECTOR('',#41749,10.) ;
#9987=VECTOR('',#41766,10.) ;
#9988=VECTOR('',#41769,0.125) ;
#9989=VECTOR('',#41772,10.) ;
#9990=VECTOR('',#41773,10.) ;
#9991=VECTOR('',#41776,10.) ;
#9992=VECTOR('',#41777,10.) ;
#9993=VECTOR('',#41780,10.) ;
#9994=VECTOR('',#41783,0.125) ;
#9995=VECTOR('',#41788,10.) ;
#9996=VECTOR('',#41789,10.) ;
#9997=VECTOR('',#41792,10.) ;
#9998=VECTOR('',#41793,10.) ;
#9999=VECTOR('',#41804,10.) ;
#10000=VECTOR('',#41805,10.) ;
#10001=VECTOR('',#41810,10.) ;
#10002=VECTOR('',#41813,10.) ;
#10003=VECTOR('',#41818,10.) ;
#10004=VECTOR('',#41833,10.) ;
#10005=VECTOR('',#41844,10.) ;
#10006=VECTOR('',#41861,10.) ;
#10007=VECTOR('',#41866,10.) ;
#10008=VECTOR('',#41877,10.) ;
#10009=VECTOR('',#41880,10.) ;
#10010=VECTOR('',#41881,10.) ;
#10011=VECTOR('',#41886,10.) ;
#10012=VECTOR('',#41889,10.) ;
#10013=VECTOR('',#41898,10.) ;
#10014=VECTOR('',#41913,10.) ;
#10015=VECTOR('',#41914,10.) ;
#10016=VECTOR('',#41915,10.) ;
#10017=VECTOR('',#41916,10.) ;
#10018=VECTOR('',#41957,10.) ;
#10019=VECTOR('',#41960,10.) ;
#10020=VECTOR('',#41971,10.) ;
#10021=VECTOR('',#41988,10.) ;
#10022=VECTOR('',#41993,10.) ;
#10023=VECTOR('',#42004,10.) ;
#10024=VECTOR('',#42007,10.) ;
#10025=VECTOR('',#42008,10.) ;
#10026=VECTOR('',#42013,10.) ;
#10027=VECTOR('',#42016,10.) ;
#10028=VECTOR('',#42027,10.) ;
#10029=VECTOR('',#42044,10.) ;
#10030=VECTOR('',#42045,10.) ;
#10031=VECTOR('',#42046,10.) ;
#10032=VECTOR('',#42047,10.) ;
#10033=VECTOR('',#42066,10.) ;
#10034=VECTOR('',#42073,10.) ;
#10035=VECTOR('',#42094,10.) ;
#10036=VECTOR('',#42097,10.) ;
#10037=VECTOR('',#42108,10.) ;
#10038=VECTOR('',#42125,10.) ;
#10039=VECTOR('',#42130,10.) ;
#10040=VECTOR('',#42141,10.) ;
#10041=VECTOR('',#42144,10.) ;
#10042=VECTOR('',#42145,10.) ;
#10043=VECTOR('',#42150,10.) ;
#10044=VECTOR('',#42153,10.) ;
#10045=VECTOR('',#42164,10.) ;
#10046=VECTOR('',#42181,10.) ;
#10047=VECTOR('',#42182,10.) ;
#10048=VECTOR('',#42183,10.) ;
#10049=VECTOR('',#42184,10.) ;
#10050=VECTOR('',#42203,10.) ;
#10051=VECTOR('',#42210,10.) ;
#10052=VECTOR('',#42231,10.) ;
#10053=VECTOR('',#42234,10.) ;
#10054=VECTOR('',#42245,10.) ;
#10055=VECTOR('',#42262,10.) ;
#10056=VECTOR('',#42267,10.) ;
#10057=VECTOR('',#42278,10.) ;
#10058=VECTOR('',#42281,10.) ;
#10059=VECTOR('',#42282,10.) ;
#10060=VECTOR('',#42287,10.) ;
#10061=VECTOR('',#42290,10.) ;
#10062=VECTOR('',#42301,10.) ;
#10063=VECTOR('',#42318,10.) ;
#10064=VECTOR('',#42319,10.) ;
#10065=VECTOR('',#42320,10.) ;
#10066=VECTOR('',#42321,10.) ;
#10067=VECTOR('',#42340,10.) ;
#10068=VECTOR('',#42347,10.) ;
#10069=VECTOR('',#42368,10.) ;
#10070=VECTOR('',#42371,10.) ;
#10071=VECTOR('',#42382,10.) ;
#10072=VECTOR('',#42399,10.) ;
#10073=VECTOR('',#42404,10.) ;
#10074=VECTOR('',#42415,10.) ;
#10075=VECTOR('',#42418,10.) ;
#10076=VECTOR('',#42419,10.) ;
#10077=VECTOR('',#42424,10.) ;
#10078=VECTOR('',#42427,10.) ;
#10079=VECTOR('',#42438,10.) ;
#10080=VECTOR('',#42455,10.) ;
#10081=VECTOR('',#42456,10.) ;
#10082=VECTOR('',#42457,10.) ;
#10083=VECTOR('',#42458,10.) ;
#10084=VECTOR('',#42477,10.) ;
#10085=VECTOR('',#42484,10.) ;
#10086=VECTOR('',#42505,10.) ;
#10087=VECTOR('',#42508,10.) ;
#10088=VECTOR('',#42519,10.) ;
#10089=VECTOR('',#42536,10.) ;
#10090=VECTOR('',#42541,10.) ;
#10091=VECTOR('',#42552,10.) ;
#10092=VECTOR('',#42555,10.) ;
#10093=VECTOR('',#42556,10.) ;
#10094=VECTOR('',#42561,10.) ;
#10095=VECTOR('',#42564,10.) ;
#10096=VECTOR('',#42575,10.) ;
#10097=VECTOR('',#42592,10.) ;
#10098=VECTOR('',#42593,10.) ;
#10099=VECTOR('',#42594,10.) ;
#10100=VECTOR('',#42595,10.) ;
#10101=VECTOR('',#42614,10.) ;
#10102=VECTOR('',#42621,10.) ;
#10103=VECTOR('',#42642,10.) ;
#10104=VECTOR('',#42645,10.) ;
#10105=VECTOR('',#42656,10.) ;
#10106=VECTOR('',#42673,10.) ;
#10107=VECTOR('',#42678,10.) ;
#10108=VECTOR('',#42689,10.) ;
#10109=VECTOR('',#42692,10.) ;
#10110=VECTOR('',#42693,10.) ;
#10111=VECTOR('',#42698,10.) ;
#10112=VECTOR('',#42701,10.) ;
#10113=VECTOR('',#42712,10.) ;
#10114=VECTOR('',#42729,10.) ;
#10115=VECTOR('',#42730,10.) ;
#10116=VECTOR('',#42731,10.) ;
#10117=VECTOR('',#42732,10.) ;
#10118=VECTOR('',#42751,10.) ;
#10119=VECTOR('',#42758,10.) ;
#10120=VECTOR('',#42779,10.) ;
#10121=VECTOR('',#42782,10.) ;
#10122=VECTOR('',#42793,10.) ;
#10123=VECTOR('',#42810,10.) ;
#10124=VECTOR('',#42815,10.) ;
#10125=VECTOR('',#42826,10.) ;
#10126=VECTOR('',#42829,10.) ;
#10127=VECTOR('',#42830,10.) ;
#10128=VECTOR('',#42835,10.) ;
#10129=VECTOR('',#42838,10.) ;
#10130=VECTOR('',#42849,10.) ;
#10131=VECTOR('',#42866,10.) ;
#10132=VECTOR('',#42867,10.) ;
#10133=VECTOR('',#42868,10.) ;
#10134=VECTOR('',#42869,10.) ;
#10135=VECTOR('',#42888,10.) ;
#10136=VECTOR('',#42895,10.) ;
#10137=VECTOR('',#42916,10.) ;
#10138=VECTOR('',#42919,10.) ;
#10139=VECTOR('',#42930,10.) ;
#10140=VECTOR('',#42947,10.) ;
#10141=VECTOR('',#42952,10.) ;
#10142=VECTOR('',#42963,10.) ;
#10143=VECTOR('',#42966,10.) ;
#10144=VECTOR('',#42967,10.) ;
#10145=VECTOR('',#42972,10.) ;
#10146=VECTOR('',#42975,10.) ;
#10147=VECTOR('',#42986,10.) ;
#10148=VECTOR('',#43003,10.) ;
#10149=VECTOR('',#43004,10.) ;
#10150=VECTOR('',#43005,10.) ;
#10151=VECTOR('',#43006,10.) ;
#10152=VECTOR('',#43025,10.) ;
#10153=VECTOR('',#43032,10.) ;
#10154=VECTOR('',#43047,10.) ;
#10155=VECTOR('',#43048,10.) ;
#10156=VECTOR('',#43051,10.) ;
#10157=VECTOR('',#43052,10.) ;
#10158=VECTOR('',#43055,10.) ;
#10159=VECTOR('',#43056,10.) ;
#10160=VECTOR('',#43059,10.) ;
#10161=VECTOR('',#43060,10.) ;
#10162=VECTOR('',#43063,10.) ;
#10163=VECTOR('',#43064,10.) ;
#10164=VECTOR('',#43067,10.) ;
#10165=VECTOR('',#43068,10.) ;
#10166=VECTOR('',#43071,10.) ;
#10167=VECTOR('',#43072,10.) ;
#10168=VECTOR('',#43075,10.) ;
#10169=VECTOR('',#43076,10.) ;
#10170=VECTOR('',#43079,10.) ;
#10171=VECTOR('',#43080,10.) ;
#10172=VECTOR('',#43083,10.) ;
#10173=VECTOR('',#43086,10.) ;
#10174=VECTOR('',#43089,10.) ;
#10175=VECTOR('',#43092,10.) ;
#10176=VECTOR('',#43095,10.) ;
#10177=VECTOR('',#43098,10.) ;
#10178=VECTOR('',#43101,10.) ;
#10179=VECTOR('',#43104,10.) ;
#10180=VECTOR('',#43107,10.) ;
#10181=VECTOR('',#43110,10.) ;
#10182=VECTOR('',#43113,10.) ;
#10183=VECTOR('',#43116,10.) ;
#10184=VECTOR('',#43119,10.) ;
#10185=VECTOR('',#43122,10.) ;
#10186=VECTOR('',#43125,10.) ;
#10187=VECTOR('',#43128,10.) ;
#10188=VECTOR('',#43131,10.) ;
#10189=VECTOR('',#43134,10.) ;
#10190=VECTOR('',#43137,12.00001256778) ;
#10191=VECTOR('',#43138,1.052365151151) ;
#10192=VECTOR('',#43139,10.) ;
#10193=VECTOR('',#43140,10.) ;
#10194=VECTOR('',#43141,12.00001256778) ;
#10195=VECTOR('',#43142,1.052365151151) ;
#10196=VECTOR('',#43143,10.) ;
#10197=VECTOR('',#43144,10.) ;
#10198=VECTOR('',#43145,12.00001256778) ;
#10199=VECTOR('',#43146,1.052365151151) ;
#10200=VECTOR('',#43147,10.) ;
#10201=VECTOR('',#43148,10.) ;
#10202=VECTOR('',#43149,12.00001256778) ;
#10203=VECTOR('',#43150,1.052365151151) ;
#10204=VECTOR('',#43151,10.) ;
#10205=VECTOR('',#43152,10.) ;
#10206=VECTOR('',#43153,12.00001256778) ;
#10207=VECTOR('',#43154,1.052365151151) ;
#10208=VECTOR('',#43155,12.00001251274) ;
#10209=VECTOR('',#43156,10.) ;
#10210=VECTOR('',#43157,12.00001256778) ;
#10211=VECTOR('',#43158,1.052365151151) ;
#10212=VECTOR('',#43159,12.00001251274) ;
#10213=VECTOR('',#43160,10.) ;
#10214=VECTOR('',#43161,12.00001256778) ;
#10215=VECTOR('',#43162,1.052365151151) ;
#10216=VECTOR('',#43163,12.00001251274) ;
#10217=VECTOR('',#43164,10.) ;
#10218=VECTOR('',#43165,12.00001256778) ;
#10219=VECTOR('',#43166,1.052365151151) ;
#10220=VECTOR('',#43167,12.00001256778) ;
#10221=VECTOR('',#43168,10.) ;
#10222=VECTOR('',#43169,12.00001256778) ;
#10223=VECTOR('',#43170,1.052365151151) ;
#10224=VECTOR('',#43171,10.) ;
#10225=VECTOR('',#43172,10.) ;
#10226=VECTOR('',#43173,10.) ;
#10227=VECTOR('',#43174,1.052365151151) ;
#10228=VECTOR('',#43175,10.) ;
#10229=VECTOR('',#43176,10.) ;
#10230=VECTOR('',#43181,1.07854801156) ;
#10231=VECTOR('',#43186,7.7511742566901) ;
#10232=VECTOR('',#43187,10.) ;
#10233=VECTOR('',#43188,7.75117425719307) ;
#10234=VECTOR('',#43191,1.07854801156) ;
#10235=VECTOR('',#43200,1.07854801156) ;
#10236=VECTOR('',#43207,1.07854801156) ;
#10237=VECTOR('',#43212,1.07854801156) ;
#10238=VECTOR('',#43219,1.07854801156) ;
#10239=VECTOR('',#43226,1.07854801156) ;
#10240=VECTOR('',#43235,1.07854801156) ;
#10241=VECTOR('',#43240,1.07854801156) ;
#10242=VECTOR('',#43249,7.75117425713307) ;
#10243=VECTOR('',#43250,10.) ;
#10244=VECTOR('',#43251,7.7511743083381) ;
#10245=VECTOR('',#43254,1.07854801156) ;
#10246=VECTOR('',#43259,10.) ;
#10247=VECTOR('',#43262,10.) ;
#10248=VECTOR('',#43263,10.) ;
#10249=VECTOR('',#43264,10.) ;
#10250=VECTOR('',#43265,10.) ;
#10251=VECTOR('',#43268,10.) ;
#10252=VECTOR('',#43269,10.) ;
#10253=VECTOR('',#43270,10.) ;
#10254=VECTOR('',#43271,10.) ;
#10255=VECTOR('',#43274,10.) ;
#10256=VECTOR('',#43275,10.) ;
#10257=VECTOR('',#43276,10.) ;
#10258=VECTOR('',#43277,10.) ;
#10259=VECTOR('',#43280,10.) ;
#10260=VECTOR('',#43281,10.) ;
#10261=VECTOR('',#43282,10.) ;
#10262=VECTOR('',#43283,10.) ;
#10263=VECTOR('',#43286,10.) ;
#10264=VECTOR('',#43287,10.) ;
#10265=VECTOR('',#43288,10.) ;
#10266=VECTOR('',#43289,10.) ;
#10267=VECTOR('',#43292,10.) ;
#10268=VECTOR('',#43293,10.) ;
#10269=VECTOR('',#43294,10.) ;
#10270=VECTOR('',#43295,10.) ;
#10271=VECTOR('',#43298,10.) ;
#10272=VECTOR('',#43299,10.) ;
#10273=VECTOR('',#43300,10.) ;
#10274=VECTOR('',#43301,10.) ;
#10275=VECTOR('',#43304,10.) ;
#10276=VECTOR('',#43305,10.) ;
#10277=VECTOR('',#43306,10.) ;
#10278=VECTOR('',#43307,10.) ;
#10279=VECTOR('',#43310,14.2521643894801) ;
#10280=VECTOR('',#43311,10.) ;
#10281=VECTOR('',#43314,7.75117425713307) ;
#10282=VECTOR('',#43315,10.) ;
#10283=VECTOR('',#43316,7.7511742567501) ;
#10284=VECTOR('',#43319,7.7511742566901) ;
#10285=VECTOR('',#43320,10.) ;
#10286=VECTOR('',#43321,7.75117425719307) ;
#10287=VECTOR('',#43324,7.75117425713307) ;
#10288=VECTOR('',#43325,10.) ;
#10289=VECTOR('',#43326,7.7511743083381) ;
#10290=VECTOR('',#43329,7.7511742566901) ;
#10291=VECTOR('',#43330,10.) ;
#10292=VECTOR('',#43331,7.75117425719307) ;
#10293=VECTOR('',#43334,7.75117425713307) ;
#10294=VECTOR('',#43335,10.) ;
#10295=VECTOR('',#43336,7.7511742567501) ;
#10296=VECTOR('',#43339,7.7511742566901) ;
#10297=VECTOR('',#43340,10.) ;
#10298=VECTOR('',#43341,7.75117425719307) ;
#10299=VECTOR('',#43344,7.75117425713307) ;
#10300=VECTOR('',#43345,10.) ;
#10301=VECTOR('',#43346,7.7511742567501) ;
#10302=VECTOR('',#43349,7.7511742566901) ;
#10303=VECTOR('',#43350,10.) ;
#10304=VECTOR('',#43351,7.75117425719307) ;
#10305=VECTOR('',#43354,7.75117425713307) ;
#10306=VECTOR('',#43355,10.) ;
#10307=VECTOR('',#43356,7.7511743083381) ;
#10308=VECTOR('',#43359,7.7511742566901) ;
#10309=VECTOR('',#43360,10.) ;
#10310=VECTOR('',#43361,7.75117425719307) ;
#10311=VECTOR('',#43364,7.75117425713307) ;
#10312=VECTOR('',#43365,10.) ;
#10313=VECTOR('',#43366,7.7511743083381) ;
#10314=VECTOR('',#43369,7.7511742566901) ;
#10315=VECTOR('',#43370,10.) ;
#10316=VECTOR('',#43371,7.75117425719307) ;
#10317=VECTOR('',#43374,7.75117425713307) ;
#10318=VECTOR('',#43375,10.) ;
#10319=VECTOR('',#43376,7.7511743083381) ;
#10320=VECTOR('',#43379,7.7511742566901) ;
#10321=VECTOR('',#43380,10.) ;
#10322=VECTOR('',#43381,7.75117425719307) ;
#10323=VECTOR('',#43384,7.75117425713307) ;
#10324=VECTOR('',#43385,10.) ;
#10325=VECTOR('',#43386,7.7511742567501) ;
#10326=VECTOR('',#43389,7.7511742566901) ;
#10327=VECTOR('',#43390,10.) ;
#10328=VECTOR('',#43391,7.75117425719307) ;
#10329=VECTOR('',#43396,10.) ;
#10330=VECTOR('',#43399,10.) ;
#10331=VECTOR('',#43402,10.) ;
#10332=VECTOR('',#43405,10.) ;
#10333=VECTOR('',#43408,10.) ;
#10334=VECTOR('',#43411,10.) ;
#10335=VECTOR('',#43414,10.) ;
#10336=VECTOR('',#43417,10.) ;
#10337=VECTOR('',#43420,10.) ;
#10338=VECTOR('',#43437,2.8575) ;
#10339=VECTOR('',#43444,10.) ;
#10340=VECTOR('',#43463,2.8575) ;
#10341=VECTOR('',#43470,10.) ;
#10342=VECTOR('',#43489,2.8575) ;
#10343=VECTOR('',#43496,10.) ;
#10344=VECTOR('',#43515,2.8575) ;
#10345=VECTOR('',#43522,10.) ;
#10346=VECTOR('',#43541,2.8575) ;
#10347=VECTOR('',#43548,10.) ;
#10348=VECTOR('',#43567,2.8575) ;
#10349=VECTOR('',#43574,10.) ;
#10350=VECTOR('',#43593,2.8575) ;
#10351=VECTOR('',#43600,10.) ;
#10352=VECTOR('',#43619,2.8575) ;
#10353=VECTOR('',#43626,10.) ;
#10354=VECTOR('',#43641,2.8575) ;
#10355=VECTOR('',#43648,14.2521643894201) ;
#10356=VECTOR('',#43653,10.) ;
#10357=VECTOR('',#43656,10.) ;
#10358=VECTOR('',#43659,10.) ;
#10359=VECTOR('',#43666,10.) ;
#10360=VECTOR('',#43669,10.) ;
#10361=VECTOR('',#43672,10.) ;
#10362=VECTOR('',#43679,10.) ;
#10363=VECTOR('',#43682,10.) ;
#10364=VECTOR('',#43685,10.) ;
#10365=VECTOR('',#43692,10.) ;
#10366=VECTOR('',#43695,10.) ;
#10367=VECTOR('',#43698,10.) ;
#10368=VECTOR('',#43705,10.) ;
#10369=VECTOR('',#43708,10.) ;
#10370=VECTOR('',#43711,10.) ;
#10371=VECTOR('',#43718,10.) ;
#10372=VECTOR('',#43721,10.) ;
#10373=VECTOR('',#43724,10.) ;
#10374=VECTOR('',#43731,10.) ;
#10375=VECTOR('',#43734,10.) ;
#10376=VECTOR('',#43737,10.) ;
#10377=VECTOR('',#43744,10.) ;
#10378=VECTOR('',#43747,10.) ;
#10379=VECTOR('',#43750,10.) ;
#11304=CIRCLE('',#33757,1.5) ;
#11305=CIRCLE('',#33758,0.125) ;
#11306=CIRCLE('',#33759,1.625) ;
#11307=CIRCLE('',#33761,1.5) ;
#11308=CIRCLE('',#33763,0.375) ;
#11309=CIRCLE('',#33764,0.375) ;
#11310=CIRCLE('',#33765,0.375) ;
#11311=CIRCLE('',#33766,0.375) ;
#11312=CIRCLE('',#33768,1.5) ;
#11313=CIRCLE('',#33769,0.125) ;
#11314=CIRCLE('',#33770,1.625) ;
#11315=CIRCLE('',#33772,1.5) ;
#11316=CIRCLE('',#33774,0.375) ;
#11317=CIRCLE('',#33775,0.375) ;
#11318=CIRCLE('',#33776,0.375) ;
#11319=CIRCLE('',#33777,0.375) ;
#11320=CIRCLE('',#33779,1.5) ;
#11321=CIRCLE('',#33780,0.125) ;
#11322=CIRCLE('',#33781,1.625) ;
#11323=CIRCLE('',#33783,1.5) ;
#11324=CIRCLE('',#33785,0.375) ;
#11325=CIRCLE('',#33786,0.375) ;
#11326=CIRCLE('',#33787,0.375) ;
#11327=CIRCLE('',#33788,0.375) ;
#11328=CIRCLE('',#33790,1.5) ;
#11329=CIRCLE('',#33791,0.125) ;
#11330=CIRCLE('',#33792,1.625) ;
#11331=CIRCLE('',#33794,1.5) ;
#11332=CIRCLE('',#33796,0.375) ;
#11333=CIRCLE('',#33797,0.375) ;
#11334=CIRCLE('',#33798,0.375) ;
#11335=CIRCLE('',#33799,0.375) ;
#11336=CIRCLE('',#33801,1.5) ;
#11337=CIRCLE('',#33802,0.125) ;
#11338=CIRCLE('',#33803,1.625) ;
#11339=CIRCLE('',#33805,1.5) ;
#11340=CIRCLE('',#33807,0.375) ;
#11341=CIRCLE('',#33808,0.375) ;
#11342=CIRCLE('',#33809,0.375) ;
#11343=CIRCLE('',#33810,0.375) ;
#11344=CIRCLE('',#33812,1.5) ;
#11345=CIRCLE('',#33813,0.125) ;
#11346=CIRCLE('',#33814,1.625) ;
#11347=CIRCLE('',#33816,1.5) ;
#11348=CIRCLE('',#33818,0.375) ;
#11349=CIRCLE('',#33819,0.375) ;
#11350=CIRCLE('',#33820,0.375) ;
#11351=CIRCLE('',#33821,0.375) ;
#11352=CIRCLE('',#33823,1.5) ;
#11353=CIRCLE('',#33824,0.125) ;
#11354=CIRCLE('',#33825,1.625) ;
#11355=CIRCLE('',#33827,1.5) ;
#11356=CIRCLE('',#33829,0.375) ;
#11357=CIRCLE('',#33830,0.375) ;
#11358=CIRCLE('',#33831,0.375) ;
#11359=CIRCLE('',#33832,0.375) ;
#11360=CIRCLE('',#33834,1.5) ;
#11361=CIRCLE('',#33835,0.125) ;
#11362=CIRCLE('',#33836,1.625) ;
#11363=CIRCLE('',#33838,1.5) ;
#11364=CIRCLE('',#33840,0.375) ;
#11365=CIRCLE('',#33841,0.375) ;
#11366=CIRCLE('',#33842,0.375) ;
#11367=CIRCLE('',#33843,0.375) ;
#11368=CIRCLE('',#33845,1.5) ;
#11369=CIRCLE('',#33846,0.125) ;
#11370=CIRCLE('',#33847,1.625) ;
#11371=CIRCLE('',#33849,0.375) ;
#11372=CIRCLE('',#33850,0.375) ;
#11373=CIRCLE('',#33851,0.375) ;
#11374=CIRCLE('',#33852,0.375) ;
#11375=CIRCLE('',#33854,1.5) ;
#11376=CIRCLE('',#33856,2.7325) ;
#11377=CIRCLE('',#33858,2.7325) ;
#11378=CIRCLE('',#33860,2.7325) ;
#11379=CIRCLE('',#33862,2.7325) ;
#11380=CIRCLE('',#33864,2.7325) ;
#11381=CIRCLE('',#33866,2.7325) ;
#11382=CIRCLE('',#33868,2.7325) ;
#11383=CIRCLE('',#33870,2.7325) ;
#11384=CIRCLE('',#33872,0.250000000000004) ;
#11385=CIRCLE('',#33873,0.249999999999986) ;
#11386=CIRCLE('',#33875,0.250000000000021) ;
#11387=CIRCLE('',#33876,0.125) ;
#11388=CIRCLE('',#33878,0.249999999999986) ;
#11389=CIRCLE('',#33880,0.250000000000057) ;
#11390=CIRCLE('',#33881,0.125) ;
#11391=CIRCLE('',#33883,0.249999999999986) ;
#11392=CIRCLE('',#33885,0.249999999999986) ;
#11393=CIRCLE('',#33886,0.125) ;
#11394=CIRCLE('',#33888,0.249999999999986) ;
#11395=CIRCLE('',#33890,0.125) ;
#11396=CIRCLE('',#33892,0.124999999999993) ;
#11397=CIRCLE('',#33894,0.188499999999969) ;
#11398=CIRCLE('',#33895,0.188499999999987) ;
#11399=CIRCLE('',#33897,0.124999999999957) ;
#11400=CIRCLE('',#33900,0.250000000000004) ;
#11401=CIRCLE('',#33901,0.249999999999986) ;
#11402=CIRCLE('',#33903,0.250000000000021) ;
#11403=CIRCLE('',#33904,0.125) ;
#11404=CIRCLE('',#33906,0.249999999999986) ;
#11405=CIRCLE('',#33908,0.250000000000057) ;
#11406=CIRCLE('',#33909,0.125) ;
#11407=CIRCLE('',#33911,0.249999999999986) ;
#11408=CIRCLE('',#33913,0.249999999999986) ;
#11409=CIRCLE('',#33914,0.125) ;
#11410=CIRCLE('',#33916,0.249999999999986) ;
#11411=CIRCLE('',#33918,0.125) ;
#11412=CIRCLE('',#33920,0.124999999999993) ;
#11413=CIRCLE('',#33922,0.188499999999969) ;
#11414=CIRCLE('',#33923,0.188499999999987) ;
#11415=CIRCLE('',#33925,0.124999999999957) ;
#11416=CIRCLE('',#33928,0.250000000000004) ;
#11417=CIRCLE('',#33929,0.249999999999986) ;
#11418=CIRCLE('',#33931,0.250000000000021) ;
#11419=CIRCLE('',#33932,0.125) ;
#11420=CIRCLE('',#33934,0.249999999999986) ;
#11421=CIRCLE('',#33936,0.250000000000057) ;
#11422=CIRCLE('',#33937,0.125) ;
#11423=CIRCLE('',#33939,0.249999999999986) ;
#11424=CIRCLE('',#33941,0.249999999999986) ;
#11425=CIRCLE('',#33942,0.125) ;
#11426=CIRCLE('',#33944,0.249999999999986) ;
#11427=CIRCLE('',#33946,0.125) ;
#11428=CIRCLE('',#33948,0.124999999999993) ;
#11429=CIRCLE('',#33950,0.188499999999969) ;
#11430=CIRCLE('',#33951,0.188499999999987) ;
#11431=CIRCLE('',#33953,0.124999999999957) ;
#11432=CIRCLE('',#33956,0.250000000000004) ;
#11433=CIRCLE('',#33957,0.249999999999986) ;
#11434=CIRCLE('',#33959,0.250000000000021) ;
#11435=CIRCLE('',#33960,0.125) ;
#11436=CIRCLE('',#33962,0.249999999999986) ;
#11437=CIRCLE('',#33964,0.250000000000057) ;
#11438=CIRCLE('',#33965,0.125) ;
#11439=CIRCLE('',#33967,0.249999999999986) ;
#11440=CIRCLE('',#33969,0.249999999999986) ;
#11441=CIRCLE('',#33970,0.125) ;
#11442=CIRCLE('',#33972,0.249999999999986) ;
#11443=CIRCLE('',#33974,0.125) ;
#11444=CIRCLE('',#33976,0.124999999999993) ;
#11445=CIRCLE('',#33978,0.188499999999969) ;
#11446=CIRCLE('',#33979,0.188499999999987) ;
#11447=CIRCLE('',#33981,0.124999999999957) ;
#11448=CIRCLE('',#33984,0.250000000000004) ;
#11449=CIRCLE('',#33985,0.249999999999986) ;
#11450=CIRCLE('',#33987,0.250000000000021) ;
#11451=CIRCLE('',#33988,0.125) ;
#11452=CIRCLE('',#33990,0.249999999999986) ;
#11453=CIRCLE('',#33992,0.250000000000057) ;
#11454=CIRCLE('',#33993,0.125) ;
#11455=CIRCLE('',#33995,0.249999999999986) ;
#11456=CIRCLE('',#33997,0.249999999999986) ;
#11457=CIRCLE('',#33998,0.125) ;
#11458=CIRCLE('',#34000,0.249999999999986) ;
#11459=CIRCLE('',#34002,0.125) ;
#11460=CIRCLE('',#34004,0.124999999999993) ;
#11461=CIRCLE('',#34006,0.188499999999969) ;
#11462=CIRCLE('',#34007,0.188499999999987) ;
#11463=CIRCLE('',#34009,0.124999999999957) ;
#11464=CIRCLE('',#34012,0.250000000000004) ;
#11465=CIRCLE('',#34013,0.249999999999986) ;
#11466=CIRCLE('',#34015,0.250000000000021) ;
#11467=CIRCLE('',#34016,0.125) ;
#11468=CIRCLE('',#34018,0.249999999999986) ;
#11469=CIRCLE('',#34020,0.250000000000057) ;
#11470=CIRCLE('',#34021,0.125) ;
#11471=CIRCLE('',#34023,0.249999999999986) ;
#11472=CIRCLE('',#34025,0.249999999999986) ;
#11473=CIRCLE('',#34026,0.125) ;
#11474=CIRCLE('',#34028,0.249999999999986) ;
#11475=CIRCLE('',#34030,0.125) ;
#11476=CIRCLE('',#34032,0.124999999999993) ;
#11477=CIRCLE('',#34034,0.188499999999969) ;
#11478=CIRCLE('',#34035,0.188499999999987) ;
#11479=CIRCLE('',#34037,0.124999999999957) ;
#11480=CIRCLE('',#34040,0.250000000000004) ;
#11481=CIRCLE('',#34041,0.249999999999986) ;
#11482=CIRCLE('',#34043,0.250000000000021) ;
#11483=CIRCLE('',#34044,0.125) ;
#11484=CIRCLE('',#34046,0.249999999999986) ;
#11485=CIRCLE('',#34048,0.250000000000057) ;
#11486=CIRCLE('',#34049,0.125) ;
#11487=CIRCLE('',#34051,0.249999999999986) ;
#11488=CIRCLE('',#34053,0.249999999999986) ;
#11489=CIRCLE('',#34054,0.125) ;
#11490=CIRCLE('',#34056,0.249999999999986) ;
#11491=CIRCLE('',#34058,0.125) ;
#11492=CIRCLE('',#34060,0.124999999999993) ;
#11493=CIRCLE('',#34062,0.188499999999969) ;
#11494=CIRCLE('',#34063,0.188499999999987) ;
#11495=CIRCLE('',#34065,0.124999999999957) ;
#11496=CIRCLE('',#34068,0.250000000000004) ;
#11497=CIRCLE('',#34069,0.249999999999986) ;
#11498=CIRCLE('',#34071,0.250000000000021) ;
#11499=CIRCLE('',#34072,0.125) ;
#11500=CIRCLE('',#34074,0.249999999999986) ;
#11501=CIRCLE('',#34076,0.250000000000057) ;
#11502=CIRCLE('',#34077,0.125) ;
#11503=CIRCLE('',#34079,0.249999999999986) ;
#11504=CIRCLE('',#34081,0.249999999999986) ;
#11505=CIRCLE('',#34082,0.125) ;
#11506=CIRCLE('',#34084,0.249999999999986) ;
#11507=CIRCLE('',#34086,0.125) ;
#11508=CIRCLE('',#34088,0.124999999999993) ;
#11509=CIRCLE('',#34090,0.188499999999969) ;
#11510=CIRCLE('',#34091,0.188499999999987) ;
#11511=CIRCLE('',#34093,0.124999999999957) ;
#11512=CIRCLE('',#34096,0.250000000000004) ;
#11513=CIRCLE('',#34097,0.249999999999986) ;
#11514=CIRCLE('',#34099,0.250000000000021) ;
#11515=CIRCLE('',#34100,0.125) ;
#11516=CIRCLE('',#34102,0.249999999999986) ;
#11517=CIRCLE('',#34104,0.250000000000057) ;
#11518=CIRCLE('',#34105,0.125) ;
#11519=CIRCLE('',#34107,0.249999999999986) ;
#11520=CIRCLE('',#34109,0.249999999999986) ;
#11521=CIRCLE('',#34110,0.125) ;
#11522=CIRCLE('',#34112,0.249999999999986) ;
#11523=CIRCLE('',#34114,0.125) ;
#11524=CIRCLE('',#34116,0.124999999999993) ;
#11525=CIRCLE('',#34118,0.188499999999987) ;
#11526=CIRCLE('',#34119,0.188499999999969) ;
#11527=CIRCLE('',#34121,0.124999999999957) ;
#11528=CIRCLE('',#34124,0.249999999999999) ;
#11529=CIRCLE('',#34125,0.249999999999986) ;
#11530=CIRCLE('',#34127,0.249999999999986) ;
#11531=CIRCLE('',#34128,0.375) ;
#11532=CIRCLE('',#34129,0.125) ;
#11533=CIRCLE('',#34131,0.24999999999995) ;
#11534=CIRCLE('',#34133,0.249999999999986) ;
#11535=CIRCLE('',#34134,0.375) ;
#11536=CIRCLE('',#34135,0.125) ;
#11537=CIRCLE('',#34137,0.249999999999986) ;
#11538=CIRCLE('',#34139,0.249999999999986) ;
#11539=CIRCLE('',#34140,0.375) ;
#11540=CIRCLE('',#34141,0.125) ;
#11541=CIRCLE('',#34143,0.249999999999986) ;
#11542=CIRCLE('',#34145,0.375) ;
#11543=CIRCLE('',#34146,0.125) ;
#11544=CIRCLE('',#34148,0.124999999999993) ;
#11545=CIRCLE('',#34151,0.124999999999993) ;
#11546=CIRCLE('',#34154,0.249999999999999) ;
#11547=CIRCLE('',#34155,0.249999999999986) ;
#11548=CIRCLE('',#34157,0.249999999999986) ;
#11549=CIRCLE('',#34158,0.375) ;
#11550=CIRCLE('',#34159,0.125) ;
#11551=CIRCLE('',#34161,0.24999999999995) ;
#11552=CIRCLE('',#34163,0.249999999999986) ;
#11553=CIRCLE('',#34164,0.375) ;
#11554=CIRCLE('',#34165,0.125) ;
#11555=CIRCLE('',#34167,0.249999999999986) ;
#11556=CIRCLE('',#34169,0.249999999999986) ;
#11557=CIRCLE('',#34170,0.375) ;
#11558=CIRCLE('',#34171,0.125) ;
#11559=CIRCLE('',#34173,0.249999999999986) ;
#11560=CIRCLE('',#34175,0.375) ;
#11561=CIRCLE('',#34176,0.125) ;
#11562=CIRCLE('',#34178,0.124999999999993) ;
#11563=CIRCLE('',#34181,0.124999999999993) ;
#11564=CIRCLE('',#34184,0.249999999999999) ;
#11565=CIRCLE('',#34185,0.249999999999986) ;
#11566=CIRCLE('',#34187,0.249999999999986) ;
#11567=CIRCLE('',#34188,0.375) ;
#11568=CIRCLE('',#34189,0.125) ;
#11569=CIRCLE('',#34191,0.24999999999995) ;
#11570=CIRCLE('',#34193,0.249999999999986) ;
#11571=CIRCLE('',#34194,0.375) ;
#11572=CIRCLE('',#34195,0.125) ;
#11573=CIRCLE('',#34197,0.249999999999986) ;
#11574=CIRCLE('',#34199,0.249999999999986) ;
#11575=CIRCLE('',#34200,0.375) ;
#11576=CIRCLE('',#34201,0.125) ;
#11577=CIRCLE('',#34203,0.249999999999986) ;
#11578=CIRCLE('',#34205,0.375) ;
#11579=CIRCLE('',#34206,0.125) ;
#11580=CIRCLE('',#34208,0.124999999999993) ;
#11581=CIRCLE('',#34211,0.124999999999993) ;
#11582=CIRCLE('',#34214,0.249999999999999) ;
#11583=CIRCLE('',#34215,0.249999999999986) ;
#11584=CIRCLE('',#34217,0.249999999999986) ;
#11585=CIRCLE('',#34218,0.375) ;
#11586=CIRCLE('',#34219,0.125) ;
#11587=CIRCLE('',#34221,0.24999999999995) ;
#11588=CIRCLE('',#34223,0.249999999999986) ;
#11589=CIRCLE('',#34224,0.375) ;
#11590=CIRCLE('',#34225,0.125) ;
#11591=CIRCLE('',#34227,0.249999999999986) ;
#11592=CIRCLE('',#34229,0.249999999999986) ;
#11593=CIRCLE('',#34230,0.375) ;
#11594=CIRCLE('',#34231,0.125) ;
#11595=CIRCLE('',#34233,0.249999999999986) ;
#11596=CIRCLE('',#34235,0.375) ;
#11597=CIRCLE('',#34236,0.125) ;
#11598=CIRCLE('',#34238,0.124999999999993) ;
#11599=CIRCLE('',#34241,0.124999999999993) ;
#11600=CIRCLE('',#34244,0.249999999999999) ;
#11601=CIRCLE('',#34245,0.249999999999986) ;
#11602=CIRCLE('',#34247,0.249999999999986) ;
#11603=CIRCLE('',#34248,0.375) ;
#11604=CIRCLE('',#34249,0.125) ;
#11605=CIRCLE('',#34251,0.24999999999995) ;
#11606=CIRCLE('',#34253,0.249999999999986) ;
#11607=CIRCLE('',#34254,0.375) ;
#11608=CIRCLE('',#34255,0.125) ;
#11609=CIRCLE('',#34257,0.249999999999986) ;
#11610=CIRCLE('',#34259,0.249999999999986) ;
#11611=CIRCLE('',#34260,0.375) ;
#11612=CIRCLE('',#34261,0.125) ;
#11613=CIRCLE('',#34263,0.249999999999986) ;
#11614=CIRCLE('',#34265,0.375) ;
#11615=CIRCLE('',#34266,0.125) ;
#11616=CIRCLE('',#34268,0.124999999999993) ;
#11617=CIRCLE('',#34271,0.124999999999993) ;
#11618=CIRCLE('',#34274,0.249999999999999) ;
#11619=CIRCLE('',#34275,0.249999999999986) ;
#11620=CIRCLE('',#34277,0.249999999999986) ;
#11621=CIRCLE('',#34278,0.375) ;
#11622=CIRCLE('',#34279,0.125) ;
#11623=CIRCLE('',#34281,0.24999999999995) ;
#11624=CIRCLE('',#34283,0.249999999999986) ;
#11625=CIRCLE('',#34284,0.375) ;
#11626=CIRCLE('',#34285,0.125) ;
#11627=CIRCLE('',#34287,0.249999999999986) ;
#11628=CIRCLE('',#34289,0.249999999999986) ;
#11629=CIRCLE('',#34290,0.375) ;
#11630=CIRCLE('',#34291,0.125) ;
#11631=CIRCLE('',#34293,0.249999999999986) ;
#11632=CIRCLE('',#34295,0.375) ;
#11633=CIRCLE('',#34296,0.125) ;
#11634=CIRCLE('',#34298,0.124999999999993) ;
#11635=CIRCLE('',#34301,0.124999999999993) ;
#11636=CIRCLE('',#34304,0.249999999999999) ;
#11637=CIRCLE('',#34305,0.249999999999986) ;
#11638=CIRCLE('',#34307,0.249999999999986) ;
#11639=CIRCLE('',#34308,0.375) ;
#11640=CIRCLE('',#34309,0.125) ;
#11641=CIRCLE('',#34311,0.24999999999995) ;
#11642=CIRCLE('',#34313,0.249999999999986) ;
#11643=CIRCLE('',#34314,0.375) ;
#11644=CIRCLE('',#34315,0.125) ;
#11645=CIRCLE('',#34317,0.249999999999986) ;
#11646=CIRCLE('',#34319,0.249999999999986) ;
#11647=CIRCLE('',#34320,0.375) ;
#11648=CIRCLE('',#34321,0.125) ;
#11649=CIRCLE('',#34323,0.249999999999986) ;
#11650=CIRCLE('',#34325,0.375) ;
#11651=CIRCLE('',#34326,0.125) ;
#11652=CIRCLE('',#34328,0.124999999999993) ;
#11653=CIRCLE('',#34331,0.124999999999993) ;
#11654=CIRCLE('',#34334,0.249999999999999) ;
#11655=CIRCLE('',#34335,0.249999999999986) ;
#11656=CIRCLE('',#34337,0.249999999999986) ;
#11657=CIRCLE('',#34338,0.375) ;
#11658=CIRCLE('',#34339,0.125) ;
#11659=CIRCLE('',#34341,0.24999999999995) ;
#11660=CIRCLE('',#34343,0.249999999999986) ;
#11661=CIRCLE('',#34344,0.375) ;
#11662=CIRCLE('',#34345,0.125) ;
#11663=CIRCLE('',#34347,0.249999999999986) ;
#11664=CIRCLE('',#34349,0.249999999999986) ;
#11665=CIRCLE('',#34350,0.375) ;
#11666=CIRCLE('',#34351,0.125) ;
#11667=CIRCLE('',#34353,0.249999999999986) ;
#11668=CIRCLE('',#34355,0.375) ;
#11669=CIRCLE('',#34356,0.125) ;
#11670=CIRCLE('',#34358,0.124999999999993) ;
#11671=CIRCLE('',#34361,0.124999999999993) ;
#11672=CIRCLE('',#34364,0.249999999999999) ;
#11673=CIRCLE('',#34365,0.249999999999915) ;
#11674=CIRCLE('',#34367,0.249999999999986) ;
#11675=CIRCLE('',#34368,0.375) ;
#11676=CIRCLE('',#34369,0.125) ;
#11677=CIRCLE('',#34371,0.24999999999995) ;
#11678=CIRCLE('',#34373,0.249999999999986) ;
#11679=CIRCLE('',#34374,0.375) ;
#11680=CIRCLE('',#34375,0.125) ;
#11681=CIRCLE('',#34377,0.249999999999986) ;
#11682=CIRCLE('',#34379,0.249999999999986) ;
#11683=CIRCLE('',#34380,0.375) ;
#11684=CIRCLE('',#34381,0.125) ;
#11685=CIRCLE('',#34383,0.249999999999986) ;
#11686=CIRCLE('',#34385,0.375) ;
#11687=CIRCLE('',#34386,0.125) ;
#11688=CIRCLE('',#34388,0.124999999999993) ;
#11689=CIRCLE('',#34390,0.188499999999987) ;
#11690=CIRCLE('',#34391,0.188499999999987) ;
#11691=CIRCLE('',#34393,0.124999999999993) ;
#11692=CIRCLE('',#34396,0.249999999999999) ;
#11693=CIRCLE('',#34397,0.249999999999915) ;
#11694=CIRCLE('',#34399,0.249999999999986) ;
#11695=CIRCLE('',#34400,0.375) ;
#11696=CIRCLE('',#34401,0.125) ;
#11697=CIRCLE('',#34403,0.24999999999995) ;
#11698=CIRCLE('',#34405,0.249999999999986) ;
#11699=CIRCLE('',#34406,0.375) ;
#11700=CIRCLE('',#34407,0.125) ;
#11701=CIRCLE('',#34409,0.249999999999986) ;
#11702=CIRCLE('',#34411,0.249999999999986) ;
#11703=CIRCLE('',#34412,0.375) ;
#11704=CIRCLE('',#34413,0.125) ;
#11705=CIRCLE('',#34415,0.249999999999986) ;
#11706=CIRCLE('',#34417,0.375) ;
#11707=CIRCLE('',#34418,0.125) ;
#11708=CIRCLE('',#34420,0.124999999999993) ;
#11709=CIRCLE('',#34422,0.188499999999987) ;
#11710=CIRCLE('',#34423,0.188499999999987) ;
#11711=CIRCLE('',#34425,0.124999999999993) ;
#11712=CIRCLE('',#34428,0.249999999999999) ;
#11713=CIRCLE('',#34429,0.249999999999915) ;
#11714=CIRCLE('',#34431,0.249999999999986) ;
#11715=CIRCLE('',#34432,0.375) ;
#11716=CIRCLE('',#34433,0.125) ;
#11717=CIRCLE('',#34435,0.24999999999995) ;
#11718=CIRCLE('',#34437,0.249999999999986) ;
#11719=CIRCLE('',#34438,0.375) ;
#11720=CIRCLE('',#34439,0.125) ;
#11721=CIRCLE('',#34441,0.249999999999986) ;
#11722=CIRCLE('',#34443,0.249999999999986) ;
#11723=CIRCLE('',#34444,0.375) ;
#11724=CIRCLE('',#34445,0.125) ;
#11725=CIRCLE('',#34447,0.249999999999986) ;
#11726=CIRCLE('',#34449,0.375) ;
#11727=CIRCLE('',#34450,0.125) ;
#11728=CIRCLE('',#34452,0.124999999999993) ;
#11729=CIRCLE('',#34454,0.188499999999987) ;
#11730=CIRCLE('',#34455,0.188499999999987) ;
#11731=CIRCLE('',#34457,0.124999999999993) ;
#11732=CIRCLE('',#34460,0.249999999999999) ;
#11733=CIRCLE('',#34461,0.249999999999915) ;
#11734=CIRCLE('',#34463,0.249999999999986) ;
#11735=CIRCLE('',#34464,0.375) ;
#11736=CIRCLE('',#34465,0.125) ;
#11737=CIRCLE('',#34467,0.24999999999995) ;
#11738=CIRCLE('',#34469,0.249999999999986) ;
#11739=CIRCLE('',#34470,0.375) ;
#11740=CIRCLE('',#34471,0.125) ;
#11741=CIRCLE('',#34473,0.249999999999986) ;
#11742=CIRCLE('',#34475,0.249999999999986) ;
#11743=CIRCLE('',#34476,0.375) ;
#11744=CIRCLE('',#34477,0.125) ;
#11745=CIRCLE('',#34479,0.249999999999986) ;
#11746=CIRCLE('',#34481,0.375) ;
#11747=CIRCLE('',#34482,0.125) ;
#11748=CIRCLE('',#34484,0.124999999999993) ;
#11749=CIRCLE('',#34486,0.188499999999987) ;
#11750=CIRCLE('',#34487,0.188499999999987) ;
#11751=CIRCLE('',#34489,0.124999999999993) ;
#11752=CIRCLE('',#34492,0.249999999999999) ;
#11753=CIRCLE('',#34493,0.249999999999915) ;
#11754=CIRCLE('',#34495,0.249999999999986) ;
#11755=CIRCLE('',#34496,0.375) ;
#11756=CIRCLE('',#34497,0.125) ;
#11757=CIRCLE('',#34499,0.24999999999995) ;
#11758=CIRCLE('',#34501,0.249999999999986) ;
#11759=CIRCLE('',#34502,0.375) ;
#11760=CIRCLE('',#34503,0.125) ;
#11761=CIRCLE('',#34505,0.249999999999986) ;
#11762=CIRCLE('',#34507,0.249999999999986) ;
#11763=CIRCLE('',#34508,0.375) ;
#11764=CIRCLE('',#34509,0.125) ;
#11765=CIRCLE('',#34511,0.249999999999986) ;
#11766=CIRCLE('',#34513,0.375) ;
#11767=CIRCLE('',#34514,0.125) ;
#11768=CIRCLE('',#34516,0.124999999999993) ;
#11769=CIRCLE('',#34518,0.188499999999987) ;
#11770=CIRCLE('',#34519,0.188499999999987) ;
#11771=CIRCLE('',#34521,0.124999999999993) ;
#11772=CIRCLE('',#34524,0.249999999999999) ;
#11773=CIRCLE('',#34525,0.249999999999915) ;
#11774=CIRCLE('',#34527,0.249999999999986) ;
#11775=CIRCLE('',#34528,0.375) ;
#11776=CIRCLE('',#34529,0.125) ;
#11777=CIRCLE('',#34531,0.24999999999995) ;
#11778=CIRCLE('',#34533,0.249999999999986) ;
#11779=CIRCLE('',#34534,0.375) ;
#11780=CIRCLE('',#34535,0.125) ;
#11781=CIRCLE('',#34537,0.249999999999986) ;
#11782=CIRCLE('',#34539,0.249999999999986) ;
#11783=CIRCLE('',#34540,0.375) ;
#11784=CIRCLE('',#34541,0.125) ;
#11785=CIRCLE('',#34543,0.249999999999986) ;
#11786=CIRCLE('',#34545,0.375) ;
#11787=CIRCLE('',#34546,0.125) ;
#11788=CIRCLE('',#34548,0.124999999999993) ;
#11789=CIRCLE('',#34550,0.188499999999987) ;
#11790=CIRCLE('',#34551,0.188499999999987) ;
#11791=CIRCLE('',#34553,0.124999999999993) ;
#11792=CIRCLE('',#34556,0.249999999999999) ;
#11793=CIRCLE('',#34557,0.249999999999915) ;
#11794=CIRCLE('',#34559,0.249999999999986) ;
#11795=CIRCLE('',#34560,0.375) ;
#11796=CIRCLE('',#34561,0.125) ;
#11797=CIRCLE('',#34563,0.24999999999995) ;
#11798=CIRCLE('',#34565,0.249999999999986) ;
#11799=CIRCLE('',#34566,0.375) ;
#11800=CIRCLE('',#34567,0.125) ;
#11801=CIRCLE('',#34569,0.249999999999986) ;
#11802=CIRCLE('',#34571,0.249999999999986) ;
#11803=CIRCLE('',#34572,0.375) ;
#11804=CIRCLE('',#34573,0.125) ;
#11805=CIRCLE('',#34575,0.249999999999986) ;
#11806=CIRCLE('',#34577,0.375) ;
#11807=CIRCLE('',#34578,0.125) ;
#11808=CIRCLE('',#34580,0.124999999999993) ;
#11809=CIRCLE('',#34582,0.188499999999987) ;
#11810=CIRCLE('',#34583,0.188499999999987) ;
#11811=CIRCLE('',#34585,0.124999999999993) ;
#11812=CIRCLE('',#34588,0.249999999999999) ;
#11813=CIRCLE('',#34589,0.249999999999915) ;
#11814=CIRCLE('',#34591,0.249999999999986) ;
#11815=CIRCLE('',#34592,0.375) ;
#11816=CIRCLE('',#34593,0.125) ;
#11817=CIRCLE('',#34595,0.24999999999995) ;
#11818=CIRCLE('',#34597,0.249999999999986) ;
#11819=CIRCLE('',#34598,0.375) ;
#11820=CIRCLE('',#34599,0.125) ;
#11821=CIRCLE('',#34601,0.249999999999986) ;
#11822=CIRCLE('',#34603,0.249999999999986) ;
#11823=CIRCLE('',#34604,0.375) ;
#11824=CIRCLE('',#34605,0.125) ;
#11825=CIRCLE('',#34607,0.249999999999986) ;
#11826=CIRCLE('',#34609,0.375) ;
#11827=CIRCLE('',#34610,0.125) ;
#11828=CIRCLE('',#34612,0.124999999999993) ;
#11829=CIRCLE('',#34614,0.188499999999987) ;
#11830=CIRCLE('',#34615,0.188499999999987) ;
#11831=CIRCLE('',#34617,0.124999999999993) ;
#11832=CIRCLE('',#34620,0.249999999999999) ;
#11833=CIRCLE('',#34621,0.249999999999986) ;
#11834=CIRCLE('',#34623,0.249999999999986) ;
#11835=CIRCLE('',#34624,0.375) ;
#11836=CIRCLE('',#34625,0.125) ;
#11837=CIRCLE('',#34627,0.24999999999995) ;
#11838=CIRCLE('',#34629,0.249999999999986) ;
#11839=CIRCLE('',#34630,0.375) ;
#11840=CIRCLE('',#34631,0.125) ;
#11841=CIRCLE('',#34633,0.249999999999986) ;
#11842=CIRCLE('',#34635,0.249999999999986) ;
#11843=CIRCLE('',#34636,0.375) ;
#11844=CIRCLE('',#34637,0.125) ;
#11845=CIRCLE('',#34639,0.249999999999986) ;
#11846=CIRCLE('',#34641,0.375) ;
#11847=CIRCLE('',#34642,0.125) ;
#11848=CIRCLE('',#34644,0.124999999999993) ;
#11849=CIRCLE('',#34647,0.124999999999993) ;
#11850=CIRCLE('',#34650,0.375) ;
#11851=CIRCLE('',#34651,0.375) ;
#11852=CIRCLE('',#34652,0.375) ;
#11853=CIRCLE('',#34653,0.375) ;
#11854=CIRCLE('',#34654,2.88334137894263) ;
#11855=CIRCLE('',#34656,0.249999999999999) ;
#11856=CIRCLE('',#34657,0.249999999999915) ;
#11857=CIRCLE('',#34659,0.249999999999986) ;
#11858=CIRCLE('',#34660,0.125) ;
#11859=CIRCLE('',#34662,0.24999999999995) ;
#11860=CIRCLE('',#34664,0.249999999999986) ;
#11861=CIRCLE('',#34665,0.125) ;
#11862=CIRCLE('',#34667,0.249999999999986) ;
#11863=CIRCLE('',#34669,0.249999999999986) ;
#11864=CIRCLE('',#34670,0.125) ;
#11865=CIRCLE('',#34672,0.249999999999986) ;
#11866=CIRCLE('',#34674,0.125) ;
#11867=CIRCLE('',#34676,0.124999999999993) ;
#11868=CIRCLE('',#34678,0.188499999999987) ;
#11869=CIRCLE('',#34679,0.188499999999987) ;
#11870=CIRCLE('',#34681,0.124999999999993) ;
#11871=CIRCLE('',#34685,0.124999999999993) ;
#11872=CIRCLE('',#34687,0.124999999999993) ;
#11873=CIRCLE('',#34690,0.125000000000006) ;
#11874=CIRCLE('',#34692,0.124999999999993) ;
#11875=CIRCLE('',#34695,2.7325) ;
#11876=CIRCLE('',#34697,0.124999999999993) ;
#11877=CIRCLE('',#34699,0.124999999999993) ;
#11878=CIRCLE('',#34700,0.124999999999993) ;
#11879=CIRCLE('',#34702,0.0634999999999941) ;
#11880=CIRCLE('',#34703,0.124999999999993) ;
#11881=CIRCLE('',#34705,0.124999999999993) ;
#11882=CIRCLE('',#34707,0.0634999999999764) ;
#11883=CIRCLE('',#34708,0.124999999999993) ;
#11884=CIRCLE('',#34710,0.0634999999999941) ;
#11885=CIRCLE('',#34711,0.124999999999993) ;
#11886=CIRCLE('',#34712,0.124999999999993) ;
#11887=CIRCLE('',#34715,0.125000000000028) ;
#11888=CIRCLE('',#34717,0.0634999999999941) ;
#11889=CIRCLE('',#34718,0.124999999999993) ;
#11890=CIRCLE('',#34720,0.124999999999993) ;
#11891=CIRCLE('',#34723,0.124999999999993) ;
#11892=CIRCLE('',#34728,0.124999999999993) ;
#11893=CIRCLE('',#34729,0.124999999999993) ;
#11894=CIRCLE('',#34737,0.124999999999993) ;
#11895=CIRCLE('',#34738,0.125000000000011) ;
#11896=CIRCLE('',#34740,0.124999999999993) ;
#11897=CIRCLE('',#34741,0.125000000000002) ;
#11898=CIRCLE('',#34744,0.124999999999993) ;
#11899=CIRCLE('',#34746,0.125000000000011) ;
#11900=CIRCLE('',#34748,0.124999999999993) ;
#11901=CIRCLE('',#34749,0.125000000000011) ;
#11902=CIRCLE('',#34753,0.124999999999993) ;
#11903=CIRCLE('',#34755,0.124999999999993) ;
#11904=CIRCLE('',#34756,0.124999999999993) ;
#11905=CIRCLE('',#34758,0.0634999999999941) ;
#11906=CIRCLE('',#34759,0.124999999999993) ;
#11907=CIRCLE('',#34761,0.124999999999993) ;
#11908=CIRCLE('',#34763,0.0634999999999764) ;
#11909=CIRCLE('',#34764,0.124999999999993) ;
#11910=CIRCLE('',#34766,0.0634999999999941) ;
#11911=CIRCLE('',#34767,0.124999999999993) ;
#11912=CIRCLE('',#34768,0.124999999999993) ;
#11913=CIRCLE('',#34771,0.125000000000028) ;
#11914=CIRCLE('',#34773,0.0634999999999941) ;
#11915=CIRCLE('',#34774,0.124999999999993) ;
#11916=CIRCLE('',#34776,0.124999999999993) ;
#11917=CIRCLE('',#34779,0.124999999999993) ;
#11918=CIRCLE('',#34782,0.124999999999993) ;
#11919=CIRCLE('',#34785,0.124999999999993) ;
#11920=CIRCLE('',#34786,0.124999999999993) ;
#11921=CIRCLE('',#34788,0.124999999999993) ;
#11922=CIRCLE('',#34795,0.124999999999993) ;
#11923=CIRCLE('',#34796,0.125000000000011) ;
#11924=CIRCLE('',#34797,0.125000000000006) ;
#11925=CIRCLE('',#34799,0.124999999999993) ;
#11926=CIRCLE('',#34800,0.125000000000002) ;
#11927=CIRCLE('',#34801,0.124999999999993) ;
#11928=CIRCLE('',#34804,0.124999999999993) ;
#11929=CIRCLE('',#34806,0.125000000000011) ;
#11930=CIRCLE('',#34808,0.124999999999993) ;
#11931=CIRCLE('',#34809,0.125000000000011) ;
#11932=CIRCLE('',#34813,0.124999999999993) ;
#11933=CIRCLE('',#34815,0.124999999999993) ;
#11934=CIRCLE('',#34816,0.124999999999993) ;
#11935=CIRCLE('',#34818,0.0634999999999941) ;
#11936=CIRCLE('',#34819,0.124999999999993) ;
#11937=CIRCLE('',#34821,0.124999999999993) ;
#11938=CIRCLE('',#34823,0.0634999999999764) ;
#11939=CIRCLE('',#34824,0.124999999999993) ;
#11940=CIRCLE('',#34826,0.0634999999999941) ;
#11941=CIRCLE('',#34827,0.124999999999993) ;
#11942=CIRCLE('',#34828,0.124999999999993) ;
#11943=CIRCLE('',#34831,0.125000000000028) ;
#11944=CIRCLE('',#34833,0.0634999999999941) ;
#11945=CIRCLE('',#34834,0.124999999999993) ;
#11946=CIRCLE('',#34836,0.124999999999993) ;
#11947=CIRCLE('',#34839,0.124999999999993) ;
#11948=CIRCLE('',#34842,0.124999999999993) ;
#11949=CIRCLE('',#34845,0.124999999999993) ;
#11950=CIRCLE('',#34846,0.124999999999993) ;
#11951=CIRCLE('',#34848,0.124999999999993) ;
#11952=CIRCLE('',#34855,0.124999999999993) ;
#11953=CIRCLE('',#34856,0.125000000000011) ;
#11954=CIRCLE('',#34857,0.125000000000006) ;
#11955=CIRCLE('',#34859,0.124999999999993) ;
#11956=CIRCLE('',#34860,0.125000000000002) ;
#11957=CIRCLE('',#34861,0.124999999999993) ;
#11958=CIRCLE('',#34864,0.124999999999993) ;
#11959=CIRCLE('',#34866,0.125000000000011) ;
#11960=CIRCLE('',#34868,0.124999999999993) ;
#11961=CIRCLE('',#34869,0.125000000000011) ;
#11962=CIRCLE('',#34873,0.124999999999993) ;
#11963=CIRCLE('',#34875,0.124999999999993) ;
#11964=CIRCLE('',#34876,0.124999999999993) ;
#11965=CIRCLE('',#34878,0.0634999999999941) ;
#11966=CIRCLE('',#34879,0.124999999999993) ;
#11967=CIRCLE('',#34881,0.124999999999993) ;
#11968=CIRCLE('',#34883,0.0634999999999764) ;
#11969=CIRCLE('',#34884,0.124999999999993) ;
#11970=CIRCLE('',#34886,0.0634999999999941) ;
#11971=CIRCLE('',#34887,0.124999999999993) ;
#11972=CIRCLE('',#34888,0.124999999999993) ;
#11973=CIRCLE('',#34891,0.125000000000028) ;
#11974=CIRCLE('',#34893,0.0634999999999941) ;
#11975=CIRCLE('',#34894,0.124999999999993) ;
#11976=CIRCLE('',#34896,0.124999999999993) ;
#11977=CIRCLE('',#34899,0.124999999999993) ;
#11978=CIRCLE('',#34902,0.124999999999993) ;
#11979=CIRCLE('',#34905,0.124999999999993) ;
#11980=CIRCLE('',#34906,0.124999999999993) ;
#11981=CIRCLE('',#34908,0.124999999999993) ;
#11982=CIRCLE('',#34915,0.124999999999993) ;
#11983=CIRCLE('',#34916,0.125000000000011) ;
#11984=CIRCLE('',#34917,0.125000000000006) ;
#11985=CIRCLE('',#34919,0.124999999999993) ;
#11986=CIRCLE('',#34920,0.125000000000002) ;
#11987=CIRCLE('',#34921,0.124999999999993) ;
#11988=CIRCLE('',#34924,0.124999999999993) ;
#11989=CIRCLE('',#34926,0.125000000000011) ;
#11990=CIRCLE('',#34928,0.124999999999993) ;
#11991=CIRCLE('',#34929,0.125000000000011) ;
#11992=CIRCLE('',#34933,0.124999999999993) ;
#11993=CIRCLE('',#34935,0.124999999999993) ;
#11994=CIRCLE('',#34936,0.124999999999993) ;
#11995=CIRCLE('',#34938,0.0634999999999941) ;
#11996=CIRCLE('',#34939,0.124999999999993) ;
#11997=CIRCLE('',#34941,0.124999999999993) ;
#11998=CIRCLE('',#34943,0.0634999999999764) ;
#11999=CIRCLE('',#34944,0.124999999999993) ;
#12000=CIRCLE('',#34946,0.0634999999999941) ;
#12001=CIRCLE('',#34947,0.124999999999993) ;
#12002=CIRCLE('',#34948,0.124999999999993) ;
#12003=CIRCLE('',#34951,0.125000000000028) ;
#12004=CIRCLE('',#34953,0.0634999999999941) ;
#12005=CIRCLE('',#34954,0.124999999999993) ;
#12006=CIRCLE('',#34956,0.124999999999993) ;
#12007=CIRCLE('',#34959,0.124999999999993) ;
#12008=CIRCLE('',#34962,0.124999999999993) ;
#12009=CIRCLE('',#34965,0.124999999999993) ;
#12010=CIRCLE('',#34966,0.124999999999993) ;
#12011=CIRCLE('',#34968,0.124999999999993) ;
#12012=CIRCLE('',#34975,0.124999999999993) ;
#12013=CIRCLE('',#34976,0.125000000000011) ;
#12014=CIRCLE('',#34977,0.125000000000006) ;
#12015=CIRCLE('',#34979,0.124999999999993) ;
#12016=CIRCLE('',#34980,0.125000000000002) ;
#12017=CIRCLE('',#34981,0.124999999999993) ;
#12018=CIRCLE('',#34984,0.124999999999993) ;
#12019=CIRCLE('',#34986,0.125000000000011) ;
#12020=CIRCLE('',#34988,0.124999999999993) ;
#12021=CIRCLE('',#34989,0.125000000000011) ;
#12022=CIRCLE('',#34993,0.124999999999993) ;
#12023=CIRCLE('',#34995,0.124999999999993) ;
#12024=CIRCLE('',#34996,0.124999999999993) ;
#12025=CIRCLE('',#34998,0.0634999999999941) ;
#12026=CIRCLE('',#34999,0.124999999999993) ;
#12027=CIRCLE('',#35001,0.124999999999993) ;
#12028=CIRCLE('',#35003,0.0634999999999764) ;
#12029=CIRCLE('',#35004,0.124999999999993) ;
#12030=CIRCLE('',#35006,0.0634999999999941) ;
#12031=CIRCLE('',#35007,0.124999999999993) ;
#12032=CIRCLE('',#35008,0.124999999999993) ;
#12033=CIRCLE('',#35011,0.125000000000028) ;
#12034=CIRCLE('',#35013,0.0634999999999941) ;
#12035=CIRCLE('',#35014,0.124999999999993) ;
#12036=CIRCLE('',#35016,0.124999999999993) ;
#12037=CIRCLE('',#35019,0.124999999999993) ;
#12038=CIRCLE('',#35022,0.124999999999993) ;
#12039=CIRCLE('',#35025,0.124999999999993) ;
#12040=CIRCLE('',#35026,0.124999999999993) ;
#12041=CIRCLE('',#35028,0.124999999999993) ;
#12042=CIRCLE('',#35035,0.124999999999993) ;
#12043=CIRCLE('',#35036,0.125000000000011) ;
#12044=CIRCLE('',#35037,0.125000000000006) ;
#12045=CIRCLE('',#35039,0.124999999999993) ;
#12046=CIRCLE('',#35040,0.125000000000002) ;
#12047=CIRCLE('',#35041,0.124999999999993) ;
#12048=CIRCLE('',#35044,0.124999999999993) ;
#12049=CIRCLE('',#35046,0.125000000000011) ;
#12050=CIRCLE('',#35048,0.124999999999993) ;
#12051=CIRCLE('',#35049,0.125000000000011) ;
#12052=CIRCLE('',#35053,0.124999999999993) ;
#12053=CIRCLE('',#35055,0.124999999999993) ;
#12054=CIRCLE('',#35056,0.124999999999993) ;
#12055=CIRCLE('',#35058,0.0634999999999941) ;
#12056=CIRCLE('',#35059,0.124999999999993) ;
#12057=CIRCLE('',#35061,0.124999999999993) ;
#12058=CIRCLE('',#35063,0.0634999999999764) ;
#12059=CIRCLE('',#35064,0.124999999999993) ;
#12060=CIRCLE('',#35066,0.0634999999999941) ;
#12061=CIRCLE('',#35067,0.124999999999993) ;
#12062=CIRCLE('',#35068,0.124999999999993) ;
#12063=CIRCLE('',#35071,0.125000000000028) ;
#12064=CIRCLE('',#35073,0.0634999999999941) ;
#12065=CIRCLE('',#35074,0.124999999999993) ;
#12066=CIRCLE('',#35076,0.124999999999993) ;
#12067=CIRCLE('',#35079,0.124999999999993) ;
#12068=CIRCLE('',#35082,0.124999999999993) ;
#12069=CIRCLE('',#35085,0.124999999999993) ;
#12070=CIRCLE('',#35086,0.124999999999993) ;
#12071=CIRCLE('',#35088,0.124999999999993) ;
#12072=CIRCLE('',#35095,0.124999999999993) ;
#12073=CIRCLE('',#35096,0.125000000000011) ;
#12074=CIRCLE('',#35097,0.125000000000006) ;
#12075=CIRCLE('',#35099,0.124999999999993) ;
#12076=CIRCLE('',#35100,0.125000000000002) ;
#12077=CIRCLE('',#35101,0.124999999999993) ;
#12078=CIRCLE('',#35104,0.124999999999993) ;
#12079=CIRCLE('',#35106,0.125000000000011) ;
#12080=CIRCLE('',#35108,0.124999999999993) ;
#12081=CIRCLE('',#35109,0.125000000000011) ;
#12082=CIRCLE('',#35113,0.124999999999993) ;
#12083=CIRCLE('',#35115,0.124999999999993) ;
#12084=CIRCLE('',#35116,0.124999999999993) ;
#12085=CIRCLE('',#35118,0.0634999999999941) ;
#12086=CIRCLE('',#35119,0.124999999999993) ;
#12087=CIRCLE('',#35121,0.124999999999993) ;
#12088=CIRCLE('',#35123,0.0634999999999764) ;
#12089=CIRCLE('',#35124,0.124999999999993) ;
#12090=CIRCLE('',#35126,0.0634999999999941) ;
#12091=CIRCLE('',#35127,0.124999999999993) ;
#12092=CIRCLE('',#35128,0.124999999999993) ;
#12093=CIRCLE('',#35131,0.125000000000028) ;
#12094=CIRCLE('',#35133,0.0634999999999941) ;
#12095=CIRCLE('',#35134,0.124999999999993) ;
#12096=CIRCLE('',#35136,0.124999999999993) ;
#12097=CIRCLE('',#35139,0.124999999999993) ;
#12098=CIRCLE('',#35142,0.124999999999993) ;
#12099=CIRCLE('',#35145,0.124999999999993) ;
#12100=CIRCLE('',#35146,0.124999999999993) ;
#12101=CIRCLE('',#35148,0.124999999999993) ;
#12102=CIRCLE('',#35155,0.124999999999993) ;
#12103=CIRCLE('',#35156,0.125000000000011) ;
#12104=CIRCLE('',#35157,0.125000000000006) ;
#12105=CIRCLE('',#35159,0.124999999999993) ;
#12106=CIRCLE('',#35160,0.125000000000002) ;
#12107=CIRCLE('',#35161,0.124999999999993) ;
#12108=CIRCLE('',#35164,0.124999999999993) ;
#12109=CIRCLE('',#35166,0.125000000000011) ;
#12110=CIRCLE('',#35168,0.124999999999993) ;
#12111=CIRCLE('',#35169,0.125000000000011) ;
#12112=CIRCLE('',#35173,0.124999999999993) ;
#12113=CIRCLE('',#35175,0.124999999999993) ;
#12114=CIRCLE('',#35176,0.124999999999993) ;
#12115=CIRCLE('',#35178,0.0634999999999941) ;
#12116=CIRCLE('',#35179,0.124999999999993) ;
#12117=CIRCLE('',#35181,0.124999999999993) ;
#12118=CIRCLE('',#35183,0.0634999999999764) ;
#12119=CIRCLE('',#35184,0.124999999999993) ;
#12120=CIRCLE('',#35186,0.0634999999999941) ;
#12121=CIRCLE('',#35187,0.124999999999993) ;
#12122=CIRCLE('',#35188,0.124999999999993) ;
#12123=CIRCLE('',#35191,0.125000000000028) ;
#12124=CIRCLE('',#35193,0.0634999999999941) ;
#12125=CIRCLE('',#35194,0.124999999999993) ;
#12126=CIRCLE('',#35196,0.124999999999993) ;
#12127=CIRCLE('',#35199,0.124999999999993) ;
#12128=CIRCLE('',#35202,0.124999999999993) ;
#12129=CIRCLE('',#35205,0.124999999999993) ;
#12130=CIRCLE('',#35206,0.124999999999993) ;
#12131=CIRCLE('',#35208,0.124999999999993) ;
#12132=CIRCLE('',#35215,0.124999999999993) ;
#12133=CIRCLE('',#35216,0.125000000000011) ;
#12134=CIRCLE('',#35217,0.125000000000006) ;
#12135=CIRCLE('',#35219,0.124999999999993) ;
#12136=CIRCLE('',#35220,0.125000000000002) ;
#12137=CIRCLE('',#35221,0.124999999999993) ;
#12138=CIRCLE('',#35224,0.124999999999993) ;
#12139=CIRCLE('',#35226,0.125000000000011) ;
#12140=CIRCLE('',#35228,0.124999999999993) ;
#12141=CIRCLE('',#35229,0.125000000000011) ;
#12142=CIRCLE('',#35329,2.88334137894263) ;
#12143=CIRCLE('',#35331,2.8575) ;
#12144=CIRCLE('',#35332,2.8575) ;
#12145=CIRCLE('',#35333,0.125) ;
#12146=CIRCLE('',#35335,2.8575) ;
#12147=CIRCLE('',#35337,0.125) ;
#12148=CIRCLE('',#35341,2.88334137894263) ;
#12149=CIRCLE('',#35343,2.8575) ;
#12150=CIRCLE('',#35344,2.8575) ;
#12151=CIRCLE('',#35345,0.125) ;
#12152=CIRCLE('',#35347,2.8575) ;
#12153=CIRCLE('',#35349,0.125) ;
#12154=CIRCLE('',#35353,2.88334137894263) ;
#12155=CIRCLE('',#35355,2.8575) ;
#12156=CIRCLE('',#35356,2.8575) ;
#12157=CIRCLE('',#35357,0.125) ;
#12158=CIRCLE('',#35359,2.8575) ;
#12159=CIRCLE('',#35361,0.125) ;
#12160=CIRCLE('',#35365,2.88334137894263) ;
#12161=CIRCLE('',#35367,2.8575) ;
#12162=CIRCLE('',#35368,2.8575) ;
#12163=CIRCLE('',#35369,0.125) ;
#12164=CIRCLE('',#35371,2.8575) ;
#12165=CIRCLE('',#35373,0.125) ;
#12166=CIRCLE('',#35377,2.88334137894263) ;
#12167=CIRCLE('',#35379,2.8575) ;
#12168=CIRCLE('',#35380,2.8575) ;
#12169=CIRCLE('',#35381,0.125) ;
#12170=CIRCLE('',#35383,2.8575) ;
#12171=CIRCLE('',#35385,0.125) ;
#12172=CIRCLE('',#35389,2.88334137894263) ;
#12173=CIRCLE('',#35391,2.8575) ;
#12174=CIRCLE('',#35392,2.8575) ;
#12175=CIRCLE('',#35393,0.125) ;
#12176=CIRCLE('',#35395,2.8575) ;
#12177=CIRCLE('',#35397,0.125) ;
#12178=CIRCLE('',#35401,2.88334137894263) ;
#12179=CIRCLE('',#35403,2.8575) ;
#12180=CIRCLE('',#35404,2.8575) ;
#12181=CIRCLE('',#35405,0.125) ;
#12182=CIRCLE('',#35407,2.8575) ;
#12183=CIRCLE('',#35409,0.125) ;
#12184=CIRCLE('',#35413,2.88334137894263) ;
#12185=CIRCLE('',#35415,2.8575) ;
#12186=CIRCLE('',#35416,2.8575) ;
#12187=CIRCLE('',#35417,0.125) ;
#12188=CIRCLE('',#35419,2.8575) ;
#12189=CIRCLE('',#35421,0.125) ;
#12190=CIRCLE('',#35425,2.8575) ;
#12191=CIRCLE('',#35426,2.8575) ;
#12192=CIRCLE('',#35427,0.125) ;
#12193=CIRCLE('',#35429,2.8575) ;
#12194=CIRCLE('',#35431,0.125) ;
#13694=VERTEX_POINT('',#69341) ;
#13695=VERTEX_POINT('',#69342) ;
#13696=VERTEX_POINT('',#69344) ;
#13697=VERTEX_POINT('',#69346) ;
#13698=VERTEX_POINT('',#69350) ;
#13699=VERTEX_POINT('',#69352) ;
#13700=VERTEX_POINT('',#69356) ;
#13701=VERTEX_POINT('',#69358) ;
#13702=VERTEX_POINT('',#69364) ;
#13703=VERTEX_POINT('',#69365) ;
#13704=VERTEX_POINT('',#69367) ;
#13705=VERTEX_POINT('',#69369) ;
#13706=VERTEX_POINT('',#69373) ;
#13707=VERTEX_POINT('',#69375) ;
#13708=VERTEX_POINT('',#69379) ;
#13709=VERTEX_POINT('',#69381) ;
#13710=VERTEX_POINT('',#69387) ;
#13711=VERTEX_POINT('',#69388) ;
#13712=VERTEX_POINT('',#69390) ;
#13713=VERTEX_POINT('',#69392) ;
#13714=VERTEX_POINT('',#69396) ;
#13715=VERTEX_POINT('',#69398) ;
#13716=VERTEX_POINT('',#69402) ;
#13717=VERTEX_POINT('',#69404) ;
#13718=VERTEX_POINT('',#69410) ;
#13719=VERTEX_POINT('',#69411) ;
#13720=VERTEX_POINT('',#69413) ;
#13721=VERTEX_POINT('',#69415) ;
#13722=VERTEX_POINT('',#69419) ;
#13723=VERTEX_POINT('',#69421) ;
#13724=VERTEX_POINT('',#69425) ;
#13725=VERTEX_POINT('',#69427) ;
#13726=VERTEX_POINT('',#69433) ;
#13727=VERTEX_POINT('',#69434) ;
#13728=VERTEX_POINT('',#69436) ;
#13729=VERTEX_POINT('',#69438) ;
#13730=VERTEX_POINT('',#69442) ;
#13731=VERTEX_POINT('',#69444) ;
#13732=VERTEX_POINT('',#69448) ;
#13733=VERTEX_POINT('',#69450) ;
#13734=VERTEX_POINT('',#69456) ;
#13735=VERTEX_POINT('',#69457) ;
#13736=VERTEX_POINT('',#69459) ;
#13737=VERTEX_POINT('',#69461) ;
#13738=VERTEX_POINT('',#69465) ;
#13739=VERTEX_POINT('',#69467) ;
#13740=VERTEX_POINT('',#69471) ;
#13741=VERTEX_POINT('',#69473) ;
#13742=VERTEX_POINT('',#69479) ;
#13743=VERTEX_POINT('',#69480) ;
#13744=VERTEX_POINT('',#69482) ;
#13745=VERTEX_POINT('',#69484) ;
#13746=VERTEX_POINT('',#69488) ;
#13747=VERTEX_POINT('',#69490) ;
#13748=VERTEX_POINT('',#69494) ;
#13749=VERTEX_POINT('',#69496) ;
#13750=VERTEX_POINT('',#69502) ;
#13751=VERTEX_POINT('',#69503) ;
#13752=VERTEX_POINT('',#69505) ;
#13753=VERTEX_POINT('',#69507) ;
#13754=VERTEX_POINT('',#69511) ;
#13755=VERTEX_POINT('',#69513) ;
#13756=VERTEX_POINT('',#69517) ;
#13757=VERTEX_POINT('',#69519) ;
#13758=VERTEX_POINT('',#69525) ;
#13759=VERTEX_POINT('',#69526) ;
#13760=VERTEX_POINT('',#69528) ;
#13761=VERTEX_POINT('',#69530) ;
#13762=VERTEX_POINT('',#69534) ;
#13763=VERTEX_POINT('',#69536) ;
#13764=VERTEX_POINT('',#69540) ;
#13765=VERTEX_POINT('',#69542) ;
#13766=VERTEX_POINT('',#69554) ;
#13767=VERTEX_POINT('',#69556) ;
#13768=VERTEX_POINT('',#69558) ;
#13769=VERTEX_POINT('',#69560) ;
#13770=VERTEX_POINT('',#69562) ;
#13771=VERTEX_POINT('',#69564) ;
#13772=VERTEX_POINT('',#69566) ;
#13773=VERTEX_POINT('',#69568) ;
#13774=VERTEX_POINT('',#69570) ;
#13775=VERTEX_POINT('',#69572) ;
#13776=VERTEX_POINT('',#69574) ;
#13777=VERTEX_POINT('',#69576) ;
#13778=VERTEX_POINT('',#69578) ;
#13779=VERTEX_POINT('',#69580) ;
#13780=VERTEX_POINT('',#69582) ;
#13781=VERTEX_POINT('',#69584) ;
#13782=VERTEX_POINT('',#69586) ;
#13783=VERTEX_POINT('',#69588) ;
#13784=VERTEX_POINT('',#69590) ;
#13785=VERTEX_POINT('',#69592) ;
#13786=VERTEX_POINT('',#69594) ;
#13787=VERTEX_POINT('',#69596) ;
#13788=VERTEX_POINT('',#69598) ;
#13789=VERTEX_POINT('',#69600) ;
#13790=VERTEX_POINT('',#69602) ;
#13791=VERTEX_POINT('',#69604) ;
#13792=VERTEX_POINT('',#69606) ;
#13793=VERTEX_POINT('',#69608) ;
#13794=VERTEX_POINT('',#69610) ;
#13795=VERTEX_POINT('',#69612) ;
#13796=VERTEX_POINT('',#69614) ;
#13797=VERTEX_POINT('',#69616) ;
#13798=VERTEX_POINT('',#69618) ;
#13799=VERTEX_POINT('',#69620) ;
#13800=VERTEX_POINT('',#69622) ;
#13801=VERTEX_POINT('',#69624) ;
#13802=VERTEX_POINT('',#69626) ;
#13803=VERTEX_POINT('',#69628) ;
#13804=VERTEX_POINT('',#69630) ;
#13805=VERTEX_POINT('',#69632) ;
#13806=VERTEX_POINT('',#69638) ;
#13807=VERTEX_POINT('',#69640) ;
#13808=VERTEX_POINT('',#69644) ;
#13809=VERTEX_POINT('',#69648) ;
#13810=VERTEX_POINT('',#69649) ;
#13811=VERTEX_POINT('',#69651) ;
#13812=VERTEX_POINT('',#69653) ;
#13813=VERTEX_POINT('',#69656) ;
#13814=VERTEX_POINT('',#69657) ;
#13815=VERTEX_POINT('',#69659) ;
#13816=VERTEX_POINT('',#69661) ;
#13817=VERTEX_POINT('',#69663) ;
#13818=VERTEX_POINT('',#69665) ;
#13819=VERTEX_POINT('',#69667) ;
#13820=VERTEX_POINT('',#69669) ;
#13821=VERTEX_POINT('',#69673) ;
#13822=VERTEX_POINT('',#69675) ;
#13823=VERTEX_POINT('',#69679) ;
#13824=VERTEX_POINT('',#69683) ;
#13825=VERTEX_POINT('',#69684) ;
#13826=VERTEX_POINT('',#69686) ;
#13827=VERTEX_POINT('',#69688) ;
#13828=VERTEX_POINT('',#69691) ;
#13829=VERTEX_POINT('',#69692) ;
#13830=VERTEX_POINT('',#69694) ;
#13831=VERTEX_POINT('',#69696) ;
#13832=VERTEX_POINT('',#69698) ;
#13833=VERTEX_POINT('',#69700) ;
#13834=VERTEX_POINT('',#69702) ;
#13835=VERTEX_POINT('',#69704) ;
#13836=VERTEX_POINT('',#69708) ;
#13837=VERTEX_POINT('',#69710) ;
#13838=VERTEX_POINT('',#69714) ;
#13839=VERTEX_POINT('',#69718) ;
#13840=VERTEX_POINT('',#69719) ;
#13841=VERTEX_POINT('',#69721) ;
#13842=VERTEX_POINT('',#69723) ;
#13843=VERTEX_POINT('',#69726) ;
#13844=VERTEX_POINT('',#69727) ;
#13845=VERTEX_POINT('',#69729) ;
#13846=VERTEX_POINT('',#69731) ;
#13847=VERTEX_POINT('',#69733) ;
#13848=VERTEX_POINT('',#69735) ;
#13849=VERTEX_POINT('',#69737) ;
#13850=VERTEX_POINT('',#69739) ;
#13851=VERTEX_POINT('',#69743) ;
#13852=VERTEX_POINT('',#69745) ;
#13853=VERTEX_POINT('',#69749) ;
#13854=VERTEX_POINT('',#69753) ;
#13855=VERTEX_POINT('',#69754) ;
#13856=VERTEX_POINT('',#69756) ;
#13857=VERTEX_POINT('',#69758) ;
#13858=VERTEX_POINT('',#69761) ;
#13859=VERTEX_POINT('',#69762) ;
#13860=VERTEX_POINT('',#69764) ;
#13861=VERTEX_POINT('',#69766) ;
#13862=VERTEX_POINT('',#69768) ;
#13863=VERTEX_POINT('',#69770) ;
#13864=VERTEX_POINT('',#69772) ;
#13865=VERTEX_POINT('',#69774) ;
#13866=VERTEX_POINT('',#69778) ;
#13867=VERTEX_POINT('',#69780) ;
#13868=VERTEX_POINT('',#69784) ;
#13869=VERTEX_POINT('',#69788) ;
#13870=VERTEX_POINT('',#69789) ;
#13871=VERTEX_POINT('',#69791) ;
#13872=VERTEX_POINT('',#69793) ;
#13873=VERTEX_POINT('',#69796) ;
#13874=VERTEX_POINT('',#69797) ;
#13875=VERTEX_POINT('',#69799) ;
#13876=VERTEX_POINT('',#69801) ;
#13877=VERTEX_POINT('',#69803) ;
#13878=VERTEX_POINT('',#69805) ;
#13879=VERTEX_POINT('',#69807) ;
#13880=VERTEX_POINT('',#69809) ;
#13881=VERTEX_POINT('',#69813) ;
#13882=VERTEX_POINT('',#69815) ;
#13883=VERTEX_POINT('',#69819) ;
#13884=VERTEX_POINT('',#69823) ;
#13885=VERTEX_POINT('',#69824) ;
#13886=VERTEX_POINT('',#69826) ;
#13887=VERTEX_POINT('',#69828) ;
#13888=VERTEX_POINT('',#69831) ;
#13889=VERTEX_POINT('',#69832) ;
#13890=VERTEX_POINT('',#69834) ;
#13891=VERTEX_POINT('',#69836) ;
#13892=VERTEX_POINT('',#69838) ;
#13893=VERTEX_POINT('',#69840) ;
#13894=VERTEX_POINT('',#69842) ;
#13895=VERTEX_POINT('',#69844) ;
#13896=VERTEX_POINT('',#69848) ;
#13897=VERTEX_POINT('',#69850) ;
#13898=VERTEX_POINT('',#69854) ;
#13899=VERTEX_POINT('',#69858) ;
#13900=VERTEX_POINT('',#69859) ;
#13901=VERTEX_POINT('',#69861) ;
#13902=VERTEX_POINT('',#69863) ;
#13903=VERTEX_POINT('',#69866) ;
#13904=VERTEX_POINT('',#69867) ;
#13905=VERTEX_POINT('',#69869) ;
#13906=VERTEX_POINT('',#69871) ;
#13907=VERTEX_POINT('',#69873) ;
#13908=VERTEX_POINT('',#69875) ;
#13909=VERTEX_POINT('',#69877) ;
#13910=VERTEX_POINT('',#69879) ;
#13911=VERTEX_POINT('',#69883) ;
#13912=VERTEX_POINT('',#69885) ;
#13913=VERTEX_POINT('',#69889) ;
#13914=VERTEX_POINT('',#69893) ;
#13915=VERTEX_POINT('',#69894) ;
#13916=VERTEX_POINT('',#69896) ;
#13917=VERTEX_POINT('',#69898) ;
#13918=VERTEX_POINT('',#69901) ;
#13919=VERTEX_POINT('',#69902) ;
#13920=VERTEX_POINT('',#69904) ;
#13921=VERTEX_POINT('',#69906) ;
#13922=VERTEX_POINT('',#69908) ;
#13923=VERTEX_POINT('',#69910) ;
#13924=VERTEX_POINT('',#69912) ;
#13925=VERTEX_POINT('',#69914) ;
#13926=VERTEX_POINT('',#69918) ;
#13927=VERTEX_POINT('',#69920) ;
#13928=VERTEX_POINT('',#69924) ;
#13929=VERTEX_POINT('',#69925) ;
#13930=VERTEX_POINT('',#69927) ;
#13931=VERTEX_POINT('',#69929) ;
#13932=VERTEX_POINT('',#69932) ;
#13933=VERTEX_POINT('',#69933) ;
#13934=VERTEX_POINT('',#69935) ;
#13935=VERTEX_POINT('',#69937) ;
#13936=VERTEX_POINT('',#69939) ;
#13937=VERTEX_POINT('',#69941) ;
#13938=VERTEX_POINT('',#69943) ;
#13939=VERTEX_POINT('',#69945) ;
#13940=VERTEX_POINT('',#69949) ;
#13941=VERTEX_POINT('',#69953) ;
#13942=VERTEX_POINT('',#69956) ;
#13943=VERTEX_POINT('',#69959) ;
#13944=VERTEX_POINT('',#69962) ;
#13945=VERTEX_POINT('',#69965) ;
#13946=VERTEX_POINT('',#69968) ;
#13947=VERTEX_POINT('',#69971) ;
#13948=VERTEX_POINT('',#69974) ;
#13949=VERTEX_POINT('',#69977) ;
#13950=VERTEX_POINT('',#69979) ;
#13951=VERTEX_POINT('',#69983) ;
#13952=VERTEX_POINT('',#69987) ;
#13953=VERTEX_POINT('',#69991) ;
#13954=VERTEX_POINT('',#69995) ;
#13955=VERTEX_POINT('',#69999) ;
#13956=VERTEX_POINT('',#70003) ;
#13957=VERTEX_POINT('',#70009) ;
#13958=VERTEX_POINT('',#70011) ;
#13959=VERTEX_POINT('',#70015) ;
#13960=VERTEX_POINT('',#70017) ;
#13961=VERTEX_POINT('',#70019) ;
#13962=VERTEX_POINT('',#70021) ;
#13963=VERTEX_POINT('',#70023) ;
#13964=VERTEX_POINT('',#70025) ;
#13965=VERTEX_POINT('',#70027) ;
#13966=VERTEX_POINT('',#70031) ;
#13967=VERTEX_POINT('',#70035) ;
#13968=VERTEX_POINT('',#70039) ;
#13969=VERTEX_POINT('',#70041) ;
#13970=VERTEX_POINT('',#70045) ;
#13971=VERTEX_POINT('',#70049) ;
#13972=VERTEX_POINT('',#70053) ;
#13973=VERTEX_POINT('',#70057) ;
#13974=VERTEX_POINT('',#70061) ;
#13975=VERTEX_POINT('',#70065) ;
#13976=VERTEX_POINT('',#70071) ;
#13977=VERTEX_POINT('',#70073) ;
#13978=VERTEX_POINT('',#70077) ;
#13979=VERTEX_POINT('',#70079) ;
#13980=VERTEX_POINT('',#70081) ;
#13981=VERTEX_POINT('',#70083) ;
#13982=VERTEX_POINT('',#70085) ;
#13983=VERTEX_POINT('',#70087) ;
#13984=VERTEX_POINT('',#70089) ;
#13985=VERTEX_POINT('',#70093) ;
#13986=VERTEX_POINT('',#70097) ;
#13987=VERTEX_POINT('',#70101) ;
#13988=VERTEX_POINT('',#70103) ;
#13989=VERTEX_POINT('',#70107) ;
#13990=VERTEX_POINT('',#70111) ;
#13991=VERTEX_POINT('',#70115) ;
#13992=VERTEX_POINT('',#70119) ;
#13993=VERTEX_POINT('',#70123) ;
#13994=VERTEX_POINT('',#70127) ;
#13995=VERTEX_POINT('',#70133) ;
#13996=VERTEX_POINT('',#70135) ;
#13997=VERTEX_POINT('',#70139) ;
#13998=VERTEX_POINT('',#70141) ;
#13999=VERTEX_POINT('',#70143) ;
#14000=VERTEX_POINT('',#70145) ;
#14001=VERTEX_POINT('',#70147) ;
#14002=VERTEX_POINT('',#70149) ;
#14003=VERTEX_POINT('',#70151) ;
#14004=VERTEX_POINT('',#70155) ;
#14005=VERTEX_POINT('',#70159) ;
#14006=VERTEX_POINT('',#70163) ;
#14007=VERTEX_POINT('',#70165) ;
#14008=VERTEX_POINT('',#70169) ;
#14009=VERTEX_POINT('',#70173) ;
#14010=VERTEX_POINT('',#70177) ;
#14011=VERTEX_POINT('',#70181) ;
#14012=VERTEX_POINT('',#70185) ;
#14013=VERTEX_POINT('',#70189) ;
#14014=VERTEX_POINT('',#70195) ;
#14015=VERTEX_POINT('',#70197) ;
#14016=VERTEX_POINT('',#70201) ;
#14017=VERTEX_POINT('',#70203) ;
#14018=VERTEX_POINT('',#70205) ;
#14019=VERTEX_POINT('',#70207) ;
#14020=VERTEX_POINT('',#70209) ;
#14021=VERTEX_POINT('',#70211) ;
#14022=VERTEX_POINT('',#70213) ;
#14023=VERTEX_POINT('',#70217) ;
#14024=VERTEX_POINT('',#70221) ;
#14025=VERTEX_POINT('',#70225) ;
#14026=VERTEX_POINT('',#70227) ;
#14027=VERTEX_POINT('',#70231) ;
#14028=VERTEX_POINT('',#70235) ;
#14029=VERTEX_POINT('',#70239) ;
#14030=VERTEX_POINT('',#70243) ;
#14031=VERTEX_POINT('',#70247) ;
#14032=VERTEX_POINT('',#70251) ;
#14033=VERTEX_POINT('',#70257) ;
#14034=VERTEX_POINT('',#70259) ;
#14035=VERTEX_POINT('',#70263) ;
#14036=VERTEX_POINT('',#70265) ;
#14037=VERTEX_POINT('',#70267) ;
#14038=VERTEX_POINT('',#70269) ;
#14039=VERTEX_POINT('',#70271) ;
#14040=VERTEX_POINT('',#70273) ;
#14041=VERTEX_POINT('',#70275) ;
#14042=VERTEX_POINT('',#70279) ;
#14043=VERTEX_POINT('',#70283) ;
#14044=VERTEX_POINT('',#70287) ;
#14045=VERTEX_POINT('',#70289) ;
#14046=VERTEX_POINT('',#70293) ;
#14047=VERTEX_POINT('',#70297) ;
#14048=VERTEX_POINT('',#70301) ;
#14049=VERTEX_POINT('',#70305) ;
#14050=VERTEX_POINT('',#70309) ;
#14051=VERTEX_POINT('',#70313) ;
#14052=VERTEX_POINT('',#70319) ;
#14053=VERTEX_POINT('',#70321) ;
#14054=VERTEX_POINT('',#70325) ;
#14055=VERTEX_POINT('',#70327) ;
#14056=VERTEX_POINT('',#70329) ;
#14057=VERTEX_POINT('',#70331) ;
#14058=VERTEX_POINT('',#70333) ;
#14059=VERTEX_POINT('',#70335) ;
#14060=VERTEX_POINT('',#70337) ;
#14061=VERTEX_POINT('',#70341) ;
#14062=VERTEX_POINT('',#70345) ;
#14063=VERTEX_POINT('',#70349) ;
#14064=VERTEX_POINT('',#70351) ;
#14065=VERTEX_POINT('',#70355) ;
#14066=VERTEX_POINT('',#70359) ;
#14067=VERTEX_POINT('',#70363) ;
#14068=VERTEX_POINT('',#70367) ;
#14069=VERTEX_POINT('',#70371) ;
#14070=VERTEX_POINT('',#70375) ;
#14071=VERTEX_POINT('',#70381) ;
#14072=VERTEX_POINT('',#70383) ;
#14073=VERTEX_POINT('',#70387) ;
#14074=VERTEX_POINT('',#70389) ;
#14075=VERTEX_POINT('',#70391) ;
#14076=VERTEX_POINT('',#70393) ;
#14077=VERTEX_POINT('',#70395) ;
#14078=VERTEX_POINT('',#70397) ;
#14079=VERTEX_POINT('',#70399) ;
#14080=VERTEX_POINT('',#70403) ;
#14081=VERTEX_POINT('',#70407) ;
#14082=VERTEX_POINT('',#70411) ;
#14083=VERTEX_POINT('',#70413) ;
#14084=VERTEX_POINT('',#70417) ;
#14085=VERTEX_POINT('',#70421) ;
#14086=VERTEX_POINT('',#70425) ;
#14087=VERTEX_POINT('',#70429) ;
#14088=VERTEX_POINT('',#70433) ;
#14089=VERTEX_POINT('',#70437) ;
#14090=VERTEX_POINT('',#70443) ;
#14091=VERTEX_POINT('',#70445) ;
#14092=VERTEX_POINT('',#70449) ;
#14093=VERTEX_POINT('',#70451) ;
#14094=VERTEX_POINT('',#70453) ;
#14095=VERTEX_POINT('',#70455) ;
#14096=VERTEX_POINT('',#70457) ;
#14097=VERTEX_POINT('',#70459) ;
#14098=VERTEX_POINT('',#70461) ;
#14099=VERTEX_POINT('',#70465) ;
#14100=VERTEX_POINT('',#70469) ;
#14101=VERTEX_POINT('',#70473) ;
#14102=VERTEX_POINT('',#70475) ;
#14103=VERTEX_POINT('',#70479) ;
#14104=VERTEX_POINT('',#70483) ;
#14105=VERTEX_POINT('',#70487) ;
#14106=VERTEX_POINT('',#70491) ;
#14107=VERTEX_POINT('',#70495) ;
#14108=VERTEX_POINT('',#70499) ;
#14109=VERTEX_POINT('',#70505) ;
#14110=VERTEX_POINT('',#70507) ;
#14111=VERTEX_POINT('',#70511) ;
#14112=VERTEX_POINT('',#70512) ;
#14113=VERTEX_POINT('',#70514) ;
#14114=VERTEX_POINT('',#70516) ;
#14115=VERTEX_POINT('',#70519) ;
#14116=VERTEX_POINT('',#70521) ;
#14117=VERTEX_POINT('',#70523) ;
#14118=VERTEX_POINT('',#70527) ;
#14119=VERTEX_POINT('',#70531) ;
#14120=VERTEX_POINT('',#70535) ;
#14121=VERTEX_POINT('',#70536) ;
#14122=VERTEX_POINT('',#70538) ;
#14123=VERTEX_POINT('',#70540) ;
#14124=VERTEX_POINT('',#70544) ;
#14125=VERTEX_POINT('',#70545) ;
#14126=VERTEX_POINT('',#70550) ;
#14127=VERTEX_POINT('',#70551) ;
#14128=VERTEX_POINT('',#70556) ;
#14129=VERTEX_POINT('',#70557) ;
#14130=VERTEX_POINT('',#70562) ;
#14131=VERTEX_POINT('',#70563) ;
#14132=VERTEX_POINT('',#70568) ;
#14133=VERTEX_POINT('',#70569) ;
#14134=VERTEX_POINT('',#70574) ;
#14135=VERTEX_POINT('',#70575) ;
#14136=VERTEX_POINT('',#70583) ;
#14137=VERTEX_POINT('',#70585) ;
#14138=VERTEX_POINT('',#70589) ;
#14139=VERTEX_POINT('',#70593) ;
#14140=VERTEX_POINT('',#70597) ;
#14141=VERTEX_POINT('',#70601) ;
#14142=VERTEX_POINT('',#70602) ;
#14143=VERTEX_POINT('',#70604) ;
#14144=VERTEX_POINT('',#70606) ;
#14145=VERTEX_POINT('',#70610) ;
#14146=VERTEX_POINT('',#70611) ;
#14147=VERTEX_POINT('',#70616) ;
#14148=VERTEX_POINT('',#70617) ;
#14149=VERTEX_POINT('',#70622) ;
#14150=VERTEX_POINT('',#70623) ;
#14151=VERTEX_POINT('',#70628) ;
#14152=VERTEX_POINT('',#70629) ;
#14153=VERTEX_POINT('',#70634) ;
#14154=VERTEX_POINT('',#70635) ;
#14155=VERTEX_POINT('',#70640) ;
#14156=VERTEX_POINT('',#70641) ;
#14157=VERTEX_POINT('',#70649) ;
#14158=VERTEX_POINT('',#70651) ;
#14159=VERTEX_POINT('',#70655) ;
#14160=VERTEX_POINT('',#70659) ;
#14161=VERTEX_POINT('',#70663) ;
#14162=VERTEX_POINT('',#70667) ;
#14163=VERTEX_POINT('',#70668) ;
#14164=VERTEX_POINT('',#70670) ;
#14165=VERTEX_POINT('',#70672) ;
#14166=VERTEX_POINT('',#70676) ;
#14167=VERTEX_POINT('',#70677) ;
#14168=VERTEX_POINT('',#70682) ;
#14169=VERTEX_POINT('',#70683) ;
#14170=VERTEX_POINT('',#70688) ;
#14171=VERTEX_POINT('',#70689) ;
#14172=VERTEX_POINT('',#70694) ;
#14173=VERTEX_POINT('',#70695) ;
#14174=VERTEX_POINT('',#70700) ;
#14175=VERTEX_POINT('',#70701) ;
#14176=VERTEX_POINT('',#70706) ;
#14177=VERTEX_POINT('',#70707) ;
#14178=VERTEX_POINT('',#70715) ;
#14179=VERTEX_POINT('',#70717) ;
#14180=VERTEX_POINT('',#70721) ;
#14181=VERTEX_POINT('',#70725) ;
#14182=VERTEX_POINT('',#70729) ;
#14183=VERTEX_POINT('',#70733) ;
#14184=VERTEX_POINT('',#70734) ;
#14185=VERTEX_POINT('',#70736) ;
#14186=VERTEX_POINT('',#70738) ;
#14187=VERTEX_POINT('',#70742) ;
#14188=VERTEX_POINT('',#70743) ;
#14189=VERTEX_POINT('',#70748) ;
#14190=VERTEX_POINT('',#70749) ;
#14191=VERTEX_POINT('',#70754) ;
#14192=VERTEX_POINT('',#70755) ;
#14193=VERTEX_POINT('',#70760) ;
#14194=VERTEX_POINT('',#70761) ;
#14195=VERTEX_POINT('',#70766) ;
#14196=VERTEX_POINT('',#70767) ;
#14197=VERTEX_POINT('',#70772) ;
#14198=VERTEX_POINT('',#70773) ;
#14199=VERTEX_POINT('',#70781) ;
#14200=VERTEX_POINT('',#70783) ;
#14201=VERTEX_POINT('',#70787) ;
#14202=VERTEX_POINT('',#70791) ;
#14203=VERTEX_POINT('',#70795) ;
#14204=VERTEX_POINT('',#70799) ;
#14205=VERTEX_POINT('',#70800) ;
#14206=VERTEX_POINT('',#70802) ;
#14207=VERTEX_POINT('',#70804) ;
#14208=VERTEX_POINT('',#70808) ;
#14209=VERTEX_POINT('',#70809) ;
#14210=VERTEX_POINT('',#70814) ;
#14211=VERTEX_POINT('',#70815) ;
#14212=VERTEX_POINT('',#70820) ;
#14213=VERTEX_POINT('',#70821) ;
#14214=VERTEX_POINT('',#70826) ;
#14215=VERTEX_POINT('',#70827) ;
#14216=VERTEX_POINT('',#70832) ;
#14217=VERTEX_POINT('',#70833) ;
#14218=VERTEX_POINT('',#70838) ;
#14219=VERTEX_POINT('',#70839) ;
#14220=VERTEX_POINT('',#70847) ;
#14221=VERTEX_POINT('',#70849) ;
#14222=VERTEX_POINT('',#70853) ;
#14223=VERTEX_POINT('',#70857) ;
#14224=VERTEX_POINT('',#70861) ;
#14225=VERTEX_POINT('',#70865) ;
#14226=VERTEX_POINT('',#70866) ;
#14227=VERTEX_POINT('',#70868) ;
#14228=VERTEX_POINT('',#70870) ;
#14229=VERTEX_POINT('',#70874) ;
#14230=VERTEX_POINT('',#70875) ;
#14231=VERTEX_POINT('',#70880) ;
#14232=VERTEX_POINT('',#70881) ;
#14233=VERTEX_POINT('',#70886) ;
#14234=VERTEX_POINT('',#70887) ;
#14235=VERTEX_POINT('',#70892) ;
#14236=VERTEX_POINT('',#70893) ;
#14237=VERTEX_POINT('',#70898) ;
#14238=VERTEX_POINT('',#70899) ;
#14239=VERTEX_POINT('',#70904) ;
#14240=VERTEX_POINT('',#70905) ;
#14241=VERTEX_POINT('',#70913) ;
#14242=VERTEX_POINT('',#70915) ;
#14243=VERTEX_POINT('',#70919) ;
#14244=VERTEX_POINT('',#70923) ;
#14245=VERTEX_POINT('',#70927) ;
#14246=VERTEX_POINT('',#70931) ;
#14247=VERTEX_POINT('',#70932) ;
#14248=VERTEX_POINT('',#70934) ;
#14249=VERTEX_POINT('',#70936) ;
#14250=VERTEX_POINT('',#70940) ;
#14251=VERTEX_POINT('',#70941) ;
#14252=VERTEX_POINT('',#70946) ;
#14253=VERTEX_POINT('',#70947) ;
#14254=VERTEX_POINT('',#70952) ;
#14255=VERTEX_POINT('',#70953) ;
#14256=VERTEX_POINT('',#70958) ;
#14257=VERTEX_POINT('',#70959) ;
#14258=VERTEX_POINT('',#70964) ;
#14259=VERTEX_POINT('',#70965) ;
#14260=VERTEX_POINT('',#70970) ;
#14261=VERTEX_POINT('',#70971) ;
#14262=VERTEX_POINT('',#70979) ;
#14263=VERTEX_POINT('',#70981) ;
#14264=VERTEX_POINT('',#70985) ;
#14265=VERTEX_POINT('',#70989) ;
#14266=VERTEX_POINT('',#70993) ;
#14267=VERTEX_POINT('',#70997) ;
#14268=VERTEX_POINT('',#70998) ;
#14269=VERTEX_POINT('',#71000) ;
#14270=VERTEX_POINT('',#71002) ;
#14271=VERTEX_POINT('',#71006) ;
#14272=VERTEX_POINT('',#71007) ;
#14273=VERTEX_POINT('',#71012) ;
#14274=VERTEX_POINT('',#71013) ;
#14275=VERTEX_POINT('',#71018) ;
#14276=VERTEX_POINT('',#71019) ;
#14277=VERTEX_POINT('',#71024) ;
#14278=VERTEX_POINT('',#71025) ;
#14279=VERTEX_POINT('',#71030) ;
#14280=VERTEX_POINT('',#71031) ;
#14281=VERTEX_POINT('',#71036) ;
#14282=VERTEX_POINT('',#71037) ;
#14283=VERTEX_POINT('',#71045) ;
#14284=VERTEX_POINT('',#71047) ;
#14285=VERTEX_POINT('',#71051) ;
#14286=VERTEX_POINT('',#71055) ;
#14287=VERTEX_POINT('',#71059) ;
#14288=VERTEX_POINT('',#71063) ;
#14289=VERTEX_POINT('',#71064) ;
#14290=VERTEX_POINT('',#71066) ;
#14291=VERTEX_POINT('',#71068) ;
#14292=VERTEX_POINT('',#71072) ;
#14293=VERTEX_POINT('',#71073) ;
#14294=VERTEX_POINT('',#71078) ;
#14295=VERTEX_POINT('',#71079) ;
#14296=VERTEX_POINT('',#71084) ;
#14297=VERTEX_POINT('',#71085) ;
#14298=VERTEX_POINT('',#71090) ;
#14299=VERTEX_POINT('',#71091) ;
#14300=VERTEX_POINT('',#71096) ;
#14301=VERTEX_POINT('',#71101) ;
#14302=VERTEX_POINT('',#71108) ;
#14303=VERTEX_POINT('',#71110) ;
#14304=VERTEX_POINT('',#71114) ;
#14305=VERTEX_POINT('',#71116) ;
#14306=VERTEX_POINT('',#71119) ;
#14307=VERTEX_POINT('',#71121) ;
#14308=VERTEX_POINT('',#71123) ;
#14309=VERTEX_POINT('',#71127) ;
#14310=VERTEX_POINT('',#71131) ;
#14311=VERTEX_POINT('',#71135) ;
#14312=VERTEX_POINT('',#71136) ;
#14313=VERTEX_POINT('',#71138) ;
#14314=VERTEX_POINT('',#71140) ;
#14315=VERTEX_POINT('',#71144) ;
#14316=VERTEX_POINT('',#71145) ;
#14317=VERTEX_POINT('',#71150) ;
#14318=VERTEX_POINT('',#71151) ;
#14319=VERTEX_POINT('',#71156) ;
#14320=VERTEX_POINT('',#71157) ;
#14321=VERTEX_POINT('',#71162) ;
#14322=VERTEX_POINT('',#71163) ;
#14323=VERTEX_POINT('',#71168) ;
#14324=VERTEX_POINT('',#71173) ;
#14325=VERTEX_POINT('',#71180) ;
#14326=VERTEX_POINT('',#71182) ;
#14327=VERTEX_POINT('',#71186) ;
#14328=VERTEX_POINT('',#71188) ;
#14329=VERTEX_POINT('',#71191) ;
#14330=VERTEX_POINT('',#71193) ;
#14331=VERTEX_POINT('',#71195) ;
#14332=VERTEX_POINT('',#71199) ;
#14333=VERTEX_POINT('',#71203) ;
#14334=VERTEX_POINT('',#71207) ;
#14335=VERTEX_POINT('',#71208) ;
#14336=VERTEX_POINT('',#71210) ;
#14337=VERTEX_POINT('',#71212) ;
#14338=VERTEX_POINT('',#71216) ;
#14339=VERTEX_POINT('',#71217) ;
#14340=VERTEX_POINT('',#71222) ;
#14341=VERTEX_POINT('',#71223) ;
#14342=VERTEX_POINT('',#71228) ;
#14343=VERTEX_POINT('',#71229) ;
#14344=VERTEX_POINT('',#71234) ;
#14345=VERTEX_POINT('',#71235) ;
#14346=VERTEX_POINT('',#71240) ;
#14347=VERTEX_POINT('',#71245) ;
#14348=VERTEX_POINT('',#71252) ;
#14349=VERTEX_POINT('',#71254) ;
#14350=VERTEX_POINT('',#71258) ;
#14351=VERTEX_POINT('',#71260) ;
#14352=VERTEX_POINT('',#71263) ;
#14353=VERTEX_POINT('',#71265) ;
#14354=VERTEX_POINT('',#71267) ;
#14355=VERTEX_POINT('',#71271) ;
#14356=VERTEX_POINT('',#71275) ;
#14357=VERTEX_POINT('',#71279) ;
#14358=VERTEX_POINT('',#71280) ;
#14359=VERTEX_POINT('',#71282) ;
#14360=VERTEX_POINT('',#71284) ;
#14361=VERTEX_POINT('',#71288) ;
#14362=VERTEX_POINT('',#71289) ;
#14363=VERTEX_POINT('',#71294) ;
#14364=VERTEX_POINT('',#71295) ;
#14365=VERTEX_POINT('',#71300) ;
#14366=VERTEX_POINT('',#71301) ;
#14367=VERTEX_POINT('',#71306) ;
#14368=VERTEX_POINT('',#71307) ;
#14369=VERTEX_POINT('',#71312) ;
#14370=VERTEX_POINT('',#71317) ;
#14371=VERTEX_POINT('',#71324) ;
#14372=VERTEX_POINT('',#71326) ;
#14373=VERTEX_POINT('',#71330) ;
#14374=VERTEX_POINT('',#71332) ;
#14375=VERTEX_POINT('',#71335) ;
#14376=VERTEX_POINT('',#71337) ;
#14377=VERTEX_POINT('',#71339) ;
#14378=VERTEX_POINT('',#71343) ;
#14379=VERTEX_POINT('',#71347) ;
#14380=VERTEX_POINT('',#71351) ;
#14381=VERTEX_POINT('',#71352) ;
#14382=VERTEX_POINT('',#71354) ;
#14383=VERTEX_POINT('',#71356) ;
#14384=VERTEX_POINT('',#71360) ;
#14385=VERTEX_POINT('',#71361) ;
#14386=VERTEX_POINT('',#71366) ;
#14387=VERTEX_POINT('',#71367) ;
#14388=VERTEX_POINT('',#71372) ;
#14389=VERTEX_POINT('',#71373) ;
#14390=VERTEX_POINT('',#71378) ;
#14391=VERTEX_POINT('',#71379) ;
#14392=VERTEX_POINT('',#71384) ;
#14393=VERTEX_POINT('',#71389) ;
#14394=VERTEX_POINT('',#71396) ;
#14395=VERTEX_POINT('',#71398) ;
#14396=VERTEX_POINT('',#71402) ;
#14397=VERTEX_POINT('',#71404) ;
#14398=VERTEX_POINT('',#71407) ;
#14399=VERTEX_POINT('',#71409) ;
#14400=VERTEX_POINT('',#71411) ;
#14401=VERTEX_POINT('',#71415) ;
#14402=VERTEX_POINT('',#71419) ;
#14403=VERTEX_POINT('',#71423) ;
#14404=VERTEX_POINT('',#71424) ;
#14405=VERTEX_POINT('',#71426) ;
#14406=VERTEX_POINT('',#71428) ;
#14407=VERTEX_POINT('',#71432) ;
#14408=VERTEX_POINT('',#71433) ;
#14409=VERTEX_POINT('',#71438) ;
#14410=VERTEX_POINT('',#71439) ;
#14411=VERTEX_POINT('',#71444) ;
#14412=VERTEX_POINT('',#71445) ;
#14413=VERTEX_POINT('',#71450) ;
#14414=VERTEX_POINT('',#71451) ;
#14415=VERTEX_POINT('',#71456) ;
#14416=VERTEX_POINT('',#71461) ;
#14417=VERTEX_POINT('',#71468) ;
#14418=VERTEX_POINT('',#71470) ;
#14419=VERTEX_POINT('',#71474) ;
#14420=VERTEX_POINT('',#71476) ;
#14421=VERTEX_POINT('',#71479) ;
#14422=VERTEX_POINT('',#71481) ;
#14423=VERTEX_POINT('',#71483) ;
#14424=VERTEX_POINT('',#71487) ;
#14425=VERTEX_POINT('',#71491) ;
#14426=VERTEX_POINT('',#71495) ;
#14427=VERTEX_POINT('',#71496) ;
#14428=VERTEX_POINT('',#71498) ;
#14429=VERTEX_POINT('',#71500) ;
#14430=VERTEX_POINT('',#71504) ;
#14431=VERTEX_POINT('',#71505) ;
#14432=VERTEX_POINT('',#71510) ;
#14433=VERTEX_POINT('',#71511) ;
#14434=VERTEX_POINT('',#71516) ;
#14435=VERTEX_POINT('',#71517) ;
#14436=VERTEX_POINT('',#71522) ;
#14437=VERTEX_POINT('',#71523) ;
#14438=VERTEX_POINT('',#71528) ;
#14439=VERTEX_POINT('',#71533) ;
#14440=VERTEX_POINT('',#71540) ;
#14441=VERTEX_POINT('',#71542) ;
#14442=VERTEX_POINT('',#71546) ;
#14443=VERTEX_POINT('',#71548) ;
#14444=VERTEX_POINT('',#71551) ;
#14445=VERTEX_POINT('',#71553) ;
#14446=VERTEX_POINT('',#71555) ;
#14447=VERTEX_POINT('',#71559) ;
#14448=VERTEX_POINT('',#71563) ;
#14449=VERTEX_POINT('',#71567) ;
#14450=VERTEX_POINT('',#71568) ;
#14451=VERTEX_POINT('',#71570) ;
#14452=VERTEX_POINT('',#71572) ;
#14453=VERTEX_POINT('',#71576) ;
#14454=VERTEX_POINT('',#71577) ;
#14455=VERTEX_POINT('',#71582) ;
#14456=VERTEX_POINT('',#71583) ;
#14457=VERTEX_POINT('',#71588) ;
#14458=VERTEX_POINT('',#71589) ;
#14459=VERTEX_POINT('',#71594) ;
#14460=VERTEX_POINT('',#71595) ;
#14461=VERTEX_POINT('',#71600) ;
#14462=VERTEX_POINT('',#71605) ;
#14463=VERTEX_POINT('',#71612) ;
#14464=VERTEX_POINT('',#71614) ;
#14465=VERTEX_POINT('',#71618) ;
#14466=VERTEX_POINT('',#71620) ;
#14467=VERTEX_POINT('',#71623) ;
#14468=VERTEX_POINT('',#71625) ;
#14469=VERTEX_POINT('',#71627) ;
#14470=VERTEX_POINT('',#71631) ;
#14471=VERTEX_POINT('',#71635) ;
#14472=VERTEX_POINT('',#71639) ;
#14473=VERTEX_POINT('',#71640) ;
#14474=VERTEX_POINT('',#71642) ;
#14475=VERTEX_POINT('',#71644) ;
#14476=VERTEX_POINT('',#71648) ;
#14477=VERTEX_POINT('',#71649) ;
#14478=VERTEX_POINT('',#71654) ;
#14479=VERTEX_POINT('',#71655) ;
#14480=VERTEX_POINT('',#71660) ;
#14481=VERTEX_POINT('',#71661) ;
#14482=VERTEX_POINT('',#71666) ;
#14483=VERTEX_POINT('',#71667) ;
#14484=VERTEX_POINT('',#71672) ;
#14485=VERTEX_POINT('',#71673) ;
#14486=VERTEX_POINT('',#71678) ;
#14487=VERTEX_POINT('',#71679) ;
#14488=VERTEX_POINT('',#71687) ;
#14489=VERTEX_POINT('',#71689) ;
#14490=VERTEX_POINT('',#71693) ;
#14491=VERTEX_POINT('',#71697) ;
#14492=VERTEX_POINT('',#71701) ;
#14493=VERTEX_POINT('',#71705) ;
#14494=VERTEX_POINT('',#71706) ;
#14495=VERTEX_POINT('',#71708) ;
#14496=VERTEX_POINT('',#71710) ;
#14497=VERTEX_POINT('',#71713) ;
#14498=VERTEX_POINT('',#71714) ;
#14499=VERTEX_POINT('',#71716) ;
#14500=VERTEX_POINT('',#71718) ;
#14501=VERTEX_POINT('',#71720) ;
#14502=VERTEX_POINT('',#71722) ;
#14503=VERTEX_POINT('',#71724) ;
#14504=VERTEX_POINT('',#71726) ;
#14505=VERTEX_POINT('',#71729) ;
#14506=VERTEX_POINT('',#71732) ;
#14507=VERTEX_POINT('',#71734) ;
#14508=VERTEX_POINT('',#71738) ;
#14509=VERTEX_POINT('',#71742) ;
#14510=VERTEX_POINT('',#71746) ;
#14511=VERTEX_POINT('',#71750) ;
#14512=VERTEX_POINT('',#71761) ;
#14513=VERTEX_POINT('',#71763) ;
#14514=VERTEX_POINT('',#71767) ;
#14515=VERTEX_POINT('',#71769) ;
#14516=VERTEX_POINT('',#71771) ;
#14517=VERTEX_POINT('',#71774) ;
#14518=VERTEX_POINT('',#71776) ;
#14519=VERTEX_POINT('',#71780) ;
#14520=VERTEX_POINT('',#71784) ;
#14521=VERTEX_POINT('',#71788) ;
#14522=VERTEX_POINT('',#71796) ;
#14523=VERTEX_POINT('',#71800) ;
#14524=VERTEX_POINT('',#71804) ;
#14525=VERTEX_POINT('',#71810) ;
#14526=VERTEX_POINT('',#71815) ;
#14527=VERTEX_POINT('',#71817) ;
#14528=VERTEX_POINT('',#71821) ;
#14529=VERTEX_POINT('',#71825) ;
#14530=VERTEX_POINT('',#71829) ;
#14531=VERTEX_POINT('',#71833) ;
#14532=VERTEX_POINT('',#71834) ;
#14533=VERTEX_POINT('',#71844) ;
#14534=VERTEX_POINT('',#71854) ;
#14535=VERTEX_POINT('',#71871) ;
#14536=VERTEX_POINT('',#71872) ;
#14537=VERTEX_POINT('',#71874) ;
#14538=VERTEX_POINT('',#71876) ;
#14539=VERTEX_POINT('',#71898) ;
#14540=VERTEX_POINT('',#71899) ;
#14541=VERTEX_POINT('',#71902) ;
#14542=VERTEX_POINT('',#71906) ;
#14543=VERTEX_POINT('',#71910) ;
#14544=VERTEX_POINT('',#71914) ;
#14545=VERTEX_POINT('',#71918) ;
#14546=VERTEX_POINT('',#71919) ;
#14547=VERTEX_POINT('',#71929) ;
#14548=VERTEX_POINT('',#71939) ;
#14549=VERTEX_POINT('',#71958) ;
#14550=VERTEX_POINT('',#71959) ;
#14551=VERTEX_POINT('',#71961) ;
#14552=VERTEX_POINT('',#71963) ;
#14553=VERTEX_POINT('',#71967) ;
#14554=VERTEX_POINT('',#71969) ;
#14555=VERTEX_POINT('',#71973) ;
#14556=VERTEX_POINT('',#71992) ;
#14557=VERTEX_POINT('',#71993) ;
#14558=VERTEX_POINT('',#71996) ;
#14559=VERTEX_POINT('',#72000) ;
#14560=VERTEX_POINT('',#72004) ;
#14561=VERTEX_POINT('',#72008) ;
#14562=VERTEX_POINT('',#72012) ;
#14563=VERTEX_POINT('',#72013) ;
#14564=VERTEX_POINT('',#72023) ;
#14565=VERTEX_POINT('',#72033) ;
#14566=VERTEX_POINT('',#72052) ;
#14567=VERTEX_POINT('',#72053) ;
#14568=VERTEX_POINT('',#72055) ;
#14569=VERTEX_POINT('',#72057) ;
#14570=VERTEX_POINT('',#72061) ;
#14571=VERTEX_POINT('',#72063) ;
#14572=VERTEX_POINT('',#72067) ;
#14573=VERTEX_POINT('',#72086) ;
#14574=VERTEX_POINT('',#72087) ;
#14575=VERTEX_POINT('',#72090) ;
#14576=VERTEX_POINT('',#72094) ;
#14577=VERTEX_POINT('',#72098) ;
#14578=VERTEX_POINT('',#72102) ;
#14579=VERTEX_POINT('',#72106) ;
#14580=VERTEX_POINT('',#72107) ;
#14581=VERTEX_POINT('',#72117) ;
#14582=VERTEX_POINT('',#72127) ;
#14583=VERTEX_POINT('',#72146) ;
#14584=VERTEX_POINT('',#72147) ;
#14585=VERTEX_POINT('',#72149) ;
#14586=VERTEX_POINT('',#72151) ;
#14587=VERTEX_POINT('',#72155) ;
#14588=VERTEX_POINT('',#72157) ;
#14589=VERTEX_POINT('',#72161) ;
#14590=VERTEX_POINT('',#72180) ;
#14591=VERTEX_POINT('',#72181) ;
#14592=VERTEX_POINT('',#72184) ;
#14593=VERTEX_POINT('',#72188) ;
#14594=VERTEX_POINT('',#72192) ;
#14595=VERTEX_POINT('',#72196) ;
#14596=VERTEX_POINT('',#72200) ;
#14597=VERTEX_POINT('',#72201) ;
#14598=VERTEX_POINT('',#72211) ;
#14599=VERTEX_POINT('',#72221) ;
#14600=VERTEX_POINT('',#72240) ;
#14601=VERTEX_POINT('',#72241) ;
#14602=VERTEX_POINT('',#72243) ;
#14603=VERTEX_POINT('',#72245) ;
#14604=VERTEX_POINT('',#72249) ;
#14605=VERTEX_POINT('',#72251) ;
#14606=VERTEX_POINT('',#72255) ;
#14607=VERTEX_POINT('',#72274) ;
#14608=VERTEX_POINT('',#72275) ;
#14609=VERTEX_POINT('',#72278) ;
#14610=VERTEX_POINT('',#72282) ;
#14611=VERTEX_POINT('',#72286) ;
#14612=VERTEX_POINT('',#72290) ;
#14613=VERTEX_POINT('',#72294) ;
#14614=VERTEX_POINT('',#72295) ;
#14615=VERTEX_POINT('',#72305) ;
#14616=VERTEX_POINT('',#72315) ;
#14617=VERTEX_POINT('',#72334) ;
#14618=VERTEX_POINT('',#72335) ;
#14619=VERTEX_POINT('',#72337) ;
#14620=VERTEX_POINT('',#72339) ;
#14621=VERTEX_POINT('',#72343) ;
#14622=VERTEX_POINT('',#72345) ;
#14623=VERTEX_POINT('',#72349) ;
#14624=VERTEX_POINT('',#72368) ;
#14625=VERTEX_POINT('',#72369) ;
#14626=VERTEX_POINT('',#72372) ;
#14627=VERTEX_POINT('',#72376) ;
#14628=VERTEX_POINT('',#72380) ;
#14629=VERTEX_POINT('',#72384) ;
#14630=VERTEX_POINT('',#72388) ;
#14631=VERTEX_POINT('',#72389) ;
#14632=VERTEX_POINT('',#72399) ;
#14633=VERTEX_POINT('',#72409) ;
#14634=VERTEX_POINT('',#72428) ;
#14635=VERTEX_POINT('',#72429) ;
#14636=VERTEX_POINT('',#72431) ;
#14637=VERTEX_POINT('',#72433) ;
#14638=VERTEX_POINT('',#72437) ;
#14639=VERTEX_POINT('',#72439) ;
#14640=VERTEX_POINT('',#72443) ;
#14641=VERTEX_POINT('',#72462) ;
#14642=VERTEX_POINT('',#72463) ;
#14643=VERTEX_POINT('',#72466) ;
#14644=VERTEX_POINT('',#72470) ;
#14645=VERTEX_POINT('',#72474) ;
#14646=VERTEX_POINT('',#72478) ;
#14647=VERTEX_POINT('',#72482) ;
#14648=VERTEX_POINT('',#72483) ;
#14649=VERTEX_POINT('',#72493) ;
#14650=VERTEX_POINT('',#72503) ;
#14651=VERTEX_POINT('',#72522) ;
#14652=VERTEX_POINT('',#72523) ;
#14653=VERTEX_POINT('',#72525) ;
#14654=VERTEX_POINT('',#72527) ;
#14655=VERTEX_POINT('',#72531) ;
#14656=VERTEX_POINT('',#72533) ;
#14657=VERTEX_POINT('',#72537) ;
#14658=VERTEX_POINT('',#72556) ;
#14659=VERTEX_POINT('',#72557) ;
#14660=VERTEX_POINT('',#72560) ;
#14661=VERTEX_POINT('',#72564) ;
#14662=VERTEX_POINT('',#72568) ;
#14663=VERTEX_POINT('',#72572) ;
#14664=VERTEX_POINT('',#72576) ;
#14665=VERTEX_POINT('',#72577) ;
#14666=VERTEX_POINT('',#72587) ;
#14667=VERTEX_POINT('',#72597) ;
#14668=VERTEX_POINT('',#72616) ;
#14669=VERTEX_POINT('',#72617) ;
#14670=VERTEX_POINT('',#72619) ;
#14671=VERTEX_POINT('',#72621) ;
#14672=VERTEX_POINT('',#72625) ;
#14673=VERTEX_POINT('',#72627) ;
#14674=VERTEX_POINT('',#72631) ;
#14675=VERTEX_POINT('',#72711) ;
#14676=VERTEX_POINT('',#72712) ;
#14677=VERTEX_POINT('',#72714) ;
#14678=VERTEX_POINT('',#72716) ;
#14679=VERTEX_POINT('',#72718) ;
#14680=VERTEX_POINT('',#72720) ;
#14681=VERTEX_POINT('',#72722) ;
#14682=VERTEX_POINT('',#72724) ;
#14683=VERTEX_POINT('',#72726) ;
#14684=VERTEX_POINT('',#72728) ;
#14685=VERTEX_POINT('',#72730) ;
#14686=VERTEX_POINT('',#72732) ;
#14687=VERTEX_POINT('',#72734) ;
#14688=VERTEX_POINT('',#72736) ;
#14689=VERTEX_POINT('',#72738) ;
#14690=VERTEX_POINT('',#72740) ;
#14691=VERTEX_POINT('',#72742) ;
#14692=VERTEX_POINT('',#72744) ;
#14693=VERTEX_POINT('',#72746) ;
#14694=VERTEX_POINT('',#72748) ;
#14695=VERTEX_POINT('',#72750) ;
#14696=VERTEX_POINT('',#72752) ;
#14697=VERTEX_POINT('',#72754) ;
#14698=VERTEX_POINT('',#72756) ;
#14699=VERTEX_POINT('',#72758) ;
#14700=VERTEX_POINT('',#72760) ;
#14701=VERTEX_POINT('',#72762) ;
#14702=VERTEX_POINT('',#72764) ;
#14703=VERTEX_POINT('',#72766) ;
#14704=VERTEX_POINT('',#72768) ;
#14705=VERTEX_POINT('',#72770) ;
#14706=VERTEX_POINT('',#72772) ;
#14707=VERTEX_POINT('',#72774) ;
#14708=VERTEX_POINT('',#72776) ;
#14709=VERTEX_POINT('',#72778) ;
#14710=VERTEX_POINT('',#72780) ;
#14711=VERTEX_POINT('',#72782) ;
#14712=VERTEX_POINT('',#72784) ;
#14713=VERTEX_POINT('',#72786) ;
#14714=VERTEX_POINT('',#72788) ;
#14715=VERTEX_POINT('',#72792) ;
#14716=VERTEX_POINT('',#72794) ;
#14717=VERTEX_POINT('',#72799) ;
#14718=VERTEX_POINT('',#72803) ;
#14719=VERTEX_POINT('',#72804) ;
#14720=VERTEX_POINT('',#72809) ;
#14721=VERTEX_POINT('',#72811) ;
#14722=VERTEX_POINT('',#72815) ;
#14723=VERTEX_POINT('',#72817) ;
#14724=VERTEX_POINT('',#72821) ;
#14725=VERTEX_POINT('',#72822) ;
#14726=VERTEX_POINT('',#72827) ;
#14727=VERTEX_POINT('',#72828) ;
#14728=VERTEX_POINT('',#72833) ;
#14729=VERTEX_POINT('',#72834) ;
#14730=VERTEX_POINT('',#72839) ;
#14731=VERTEX_POINT('',#72841) ;
#14732=VERTEX_POINT('',#72845) ;
#14733=VERTEX_POINT('',#72846) ;
#14734=VERTEX_POINT('',#72851) ;
#14735=VERTEX_POINT('',#72853) ;
#14736=VERTEX_POINT('',#72858) ;
#14737=VERTEX_POINT('',#72864) ;
#14738=VERTEX_POINT('',#72865) ;
#14739=VERTEX_POINT('',#72867) ;
#14740=VERTEX_POINT('',#72869) ;
#14741=VERTEX_POINT('',#72873) ;
#14742=VERTEX_POINT('',#72874) ;
#14743=VERTEX_POINT('',#72876) ;
#14744=VERTEX_POINT('',#72878) ;
#14745=VERTEX_POINT('',#72882) ;
#14746=VERTEX_POINT('',#72883) ;
#14747=VERTEX_POINT('',#72885) ;
#14748=VERTEX_POINT('',#72887) ;
#14749=VERTEX_POINT('',#72891) ;
#14750=VERTEX_POINT('',#72892) ;
#14751=VERTEX_POINT('',#72894) ;
#14752=VERTEX_POINT('',#72896) ;
#14753=VERTEX_POINT('',#72900) ;
#14754=VERTEX_POINT('',#72901) ;
#14755=VERTEX_POINT('',#72903) ;
#14756=VERTEX_POINT('',#72905) ;
#14757=VERTEX_POINT('',#72909) ;
#14758=VERTEX_POINT('',#72910) ;
#14759=VERTEX_POINT('',#72912) ;
#14760=VERTEX_POINT('',#72914) ;
#14761=VERTEX_POINT('',#72918) ;
#14762=VERTEX_POINT('',#72919) ;
#14763=VERTEX_POINT('',#72921) ;
#14764=VERTEX_POINT('',#72923) ;
#14765=VERTEX_POINT('',#72927) ;
#14766=VERTEX_POINT('',#72928) ;
#14767=VERTEX_POINT('',#72930) ;
#14768=VERTEX_POINT('',#72932) ;
#14769=VERTEX_POINT('',#72940) ;
#14770=VERTEX_POINT('',#72944) ;
#14771=VERTEX_POINT('',#72950) ;
#14772=VERTEX_POINT('',#72954) ;
#14773=VERTEX_POINT('',#72960) ;
#14774=VERTEX_POINT('',#72964) ;
#14775=VERTEX_POINT('',#72970) ;
#14776=VERTEX_POINT('',#72974) ;
#14777=VERTEX_POINT('',#72980) ;
#14778=VERTEX_POINT('',#72984) ;
#14779=VERTEX_POINT('',#72990) ;
#14780=VERTEX_POINT('',#72994) ;
#14781=VERTEX_POINT('',#73000) ;
#14782=VERTEX_POINT('',#73004) ;
#14783=VERTEX_POINT('',#73010) ;
#14784=VERTEX_POINT('',#73014) ;
#14785=VERTEX_POINT('',#73038) ;
#14786=VERTEX_POINT('',#73041) ;
#14787=VERTEX_POINT('',#73042) ;
#14788=VERTEX_POINT('',#73047) ;
#14789=VERTEX_POINT('',#73056) ;
#14790=VERTEX_POINT('',#73059) ;
#14791=VERTEX_POINT('',#73060) ;
#14792=VERTEX_POINT('',#73065) ;
#14793=VERTEX_POINT('',#73074) ;
#14794=VERTEX_POINT('',#73077) ;
#14795=VERTEX_POINT('',#73078) ;
#14796=VERTEX_POINT('',#73083) ;
#14797=VERTEX_POINT('',#73092) ;
#14798=VERTEX_POINT('',#73095) ;
#14799=VERTEX_POINT('',#73096) ;
#14800=VERTEX_POINT('',#73101) ;
#14801=VERTEX_POINT('',#73110) ;
#14802=VERTEX_POINT('',#73113) ;
#14803=VERTEX_POINT('',#73114) ;
#14804=VERTEX_POINT('',#73119) ;
#14805=VERTEX_POINT('',#73128) ;
#14806=VERTEX_POINT('',#73131) ;
#14807=VERTEX_POINT('',#73132) ;
#14808=VERTEX_POINT('',#73137) ;
#14809=VERTEX_POINT('',#73146) ;
#14810=VERTEX_POINT('',#73149) ;
#14811=VERTEX_POINT('',#73150) ;
#14812=VERTEX_POINT('',#73155) ;
#14813=VERTEX_POINT('',#73164) ;
#14814=VERTEX_POINT('',#73167) ;
#14815=VERTEX_POINT('',#73168) ;
#14816=VERTEX_POINT('',#73173) ;
#14817=VERTEX_POINT('',#73182) ;
#14818=VERTEX_POINT('',#73183) ;
#14819=VERTEX_POINT('',#73188) ;
#17138=EDGE_CURVE('',#13694,#13695,#7022,.T.) ;
#17139=EDGE_CURVE('',#13694,#13696,#7023,.T.) ;
#17140=EDGE_CURVE('',#13696,#13697,#7024,.T.) ;
#17141=EDGE_CURVE('',#13695,#13697,#7025,.T.) ;
#17142=EDGE_CURVE('',#13698,#13694,#7026,.T.) ;
#17143=EDGE_CURVE('',#13699,#13698,#7027,.T.) ;
#17144=EDGE_CURVE('',#13699,#13696,#7028,.T.) ;
#17145=EDGE_CURVE('',#13695,#13700,#7029,.T.) ;
#17146=EDGE_CURVE('',#13697,#13701,#7030,.T.) ;
#17147=EDGE_CURVE('',#13700,#13701,#7031,.T.) ;
#17148=EDGE_CURVE('',#13701,#13699,#7032,.T.) ;
#17149=EDGE_CURVE('',#13702,#13703,#7033,.T.) ;
#17150=EDGE_CURVE('',#13702,#13704,#7034,.T.) ;
#17151=EDGE_CURVE('',#13704,#13705,#7035,.T.) ;
#17152=EDGE_CURVE('',#13703,#13705,#7036,.T.) ;
#17153=EDGE_CURVE('',#13706,#13702,#7037,.T.) ;
#17154=EDGE_CURVE('',#13707,#13706,#7038,.T.) ;
#17155=EDGE_CURVE('',#13707,#13704,#7039,.T.) ;
#17156=EDGE_CURVE('',#13703,#13708,#7040,.T.) ;
#17157=EDGE_CURVE('',#13705,#13709,#7041,.T.) ;
#17158=EDGE_CURVE('',#13708,#13709,#7042,.T.) ;
#17159=EDGE_CURVE('',#13709,#13707,#7043,.T.) ;
#17160=EDGE_CURVE('',#13710,#13711,#7044,.T.) ;
#17161=EDGE_CURVE('',#13710,#13712,#7045,.T.) ;
#17162=EDGE_CURVE('',#13712,#13713,#7046,.T.) ;
#17163=EDGE_CURVE('',#13711,#13713,#7047,.T.) ;
#17164=EDGE_CURVE('',#13714,#13710,#7048,.T.) ;
#17165=EDGE_CURVE('',#13714,#13715,#7049,.T.) ;
#17166=EDGE_CURVE('',#13715,#13712,#7050,.T.) ;
#17167=EDGE_CURVE('',#13716,#13714,#7051,.T.) ;
#17168=EDGE_CURVE('',#13717,#13716,#7052,.T.) ;
#17169=EDGE_CURVE('',#13717,#13715,#7053,.T.) ;
#17170=EDGE_CURVE('',#13713,#13717,#7054,.T.) ;
#17171=EDGE_CURVE('',#13718,#13719,#7055,.T.) ;
#17172=EDGE_CURVE('',#13718,#13720,#7056,.T.) ;
#17173=EDGE_CURVE('',#13720,#13721,#7057,.T.) ;
#17174=EDGE_CURVE('',#13719,#13721,#7058,.T.) ;
#17175=EDGE_CURVE('',#13722,#13718,#7059,.T.) ;
#17176=EDGE_CURVE('',#13723,#13722,#7060,.T.) ;
#17177=EDGE_CURVE('',#13723,#13720,#7061,.T.) ;
#17178=EDGE_CURVE('',#13719,#13724,#7062,.T.) ;
#17179=EDGE_CURVE('',#13721,#13725,#7063,.T.) ;
#17180=EDGE_CURVE('',#13724,#13725,#7064,.T.) ;
#17181=EDGE_CURVE('',#13725,#13723,#7065,.T.) ;
#17182=EDGE_CURVE('',#13726,#13727,#7066,.T.) ;
#17183=EDGE_CURVE('',#13726,#13728,#7067,.T.) ;
#17184=EDGE_CURVE('',#13728,#13729,#7068,.T.) ;
#17185=EDGE_CURVE('',#13727,#13729,#7069,.T.) ;
#17186=EDGE_CURVE('',#13730,#13726,#7070,.T.) ;
#17187=EDGE_CURVE('',#13731,#13730,#7071,.T.) ;
#17188=EDGE_CURVE('',#13731,#13728,#7072,.T.) ;
#17189=EDGE_CURVE('',#13727,#13732,#7073,.T.) ;
#17190=EDGE_CURVE('',#13729,#13733,#7074,.T.) ;
#17191=EDGE_CURVE('',#13732,#13733,#7075,.T.) ;
#17192=EDGE_CURVE('',#13733,#13731,#7076,.T.) ;
#17193=EDGE_CURVE('',#13734,#13735,#7077,.T.) ;
#17194=EDGE_CURVE('',#13734,#13736,#7078,.T.) ;
#17195=EDGE_CURVE('',#13736,#13737,#7079,.T.) ;
#17196=EDGE_CURVE('',#13735,#13737,#7080,.T.) ;
#17197=EDGE_CURVE('',#13738,#13734,#7081,.T.) ;
#17198=EDGE_CURVE('',#13739,#13738,#7082,.T.) ;
#17199=EDGE_CURVE('',#13739,#13736,#7083,.T.) ;
#17200=EDGE_CURVE('',#13735,#13740,#7084,.T.) ;
#17201=EDGE_CURVE('',#13737,#13741,#7085,.T.) ;
#17202=EDGE_CURVE('',#13740,#13741,#7086,.T.) ;
#17203=EDGE_CURVE('',#13741,#13739,#7087,.T.) ;
#17204=EDGE_CURVE('',#13742,#13743,#7088,.T.) ;
#17205=EDGE_CURVE('',#13742,#13744,#7089,.T.) ;
#17206=EDGE_CURVE('',#13744,#13745,#7090,.T.) ;
#17207=EDGE_CURVE('',#13743,#13745,#7091,.T.) ;
#17208=EDGE_CURVE('',#13746,#13742,#7092,.T.) ;
#17209=EDGE_CURVE('',#13746,#13747,#7093,.T.) ;
#17210=EDGE_CURVE('',#13747,#13744,#7094,.T.) ;
#17211=EDGE_CURVE('',#13748,#13746,#7095,.T.) ;
#17212=EDGE_CURVE('',#13749,#13748,#7096,.T.) ;
#17213=EDGE_CURVE('',#13749,#13747,#7097,.T.) ;
#17214=EDGE_CURVE('',#13745,#13749,#7098,.T.) ;
#17215=EDGE_CURVE('',#13750,#13751,#7099,.T.) ;
#17216=EDGE_CURVE('',#13750,#13752,#7100,.T.) ;
#17217=EDGE_CURVE('',#13752,#13753,#7101,.T.) ;
#17218=EDGE_CURVE('',#13751,#13753,#7102,.T.) ;
#17219=EDGE_CURVE('',#13754,#13750,#7103,.T.) ;
#17220=EDGE_CURVE('',#13755,#13754,#7104,.T.) ;
#17221=EDGE_CURVE('',#13755,#13752,#7105,.T.) ;
#17222=EDGE_CURVE('',#13751,#13756,#7106,.T.) ;
#17223=EDGE_CURVE('',#13753,#13757,#7107,.T.) ;
#17224=EDGE_CURVE('',#13756,#13757,#7108,.T.) ;
#17225=EDGE_CURVE('',#13757,#13755,#7109,.T.) ;
#17226=EDGE_CURVE('',#13758,#13759,#7110,.T.) ;
#17227=EDGE_CURVE('',#13758,#13760,#7111,.T.) ;
#17228=EDGE_CURVE('',#13760,#13761,#7112,.T.) ;
#17229=EDGE_CURVE('',#13759,#13761,#7113,.T.) ;
#17230=EDGE_CURVE('',#13762,#13758,#7114,.T.) ;
#17231=EDGE_CURVE('',#13763,#13762,#7115,.T.) ;
#17232=EDGE_CURVE('',#13763,#13760,#7116,.T.) ;
#17233=EDGE_CURVE('',#13759,#13764,#7117,.T.) ;
#17234=EDGE_CURVE('',#13761,#13765,#7118,.T.) ;
#17235=EDGE_CURVE('',#13764,#13765,#7119,.T.) ;
#17236=EDGE_CURVE('',#13765,#13763,#7120,.T.) ;
#17237=EDGE_CURVE('',#13724,#13698,#7121,.T.) ;
#17238=EDGE_CURVE('',#13756,#13722,#7122,.T.) ;
#17239=EDGE_CURVE('',#13740,#13754,#7123,.T.) ;
#17240=EDGE_CURVE('',#13708,#13738,#7124,.T.) ;
#17241=EDGE_CURVE('',#13711,#13706,#7125,.T.) ;
#17242=EDGE_CURVE('',#13743,#13716,#7126,.T.) ;
#17243=EDGE_CURVE('',#13766,#13748,#7127,.T.) ;
#17244=EDGE_CURVE('',#13767,#13766,#7128,.T.) ;
#17245=EDGE_CURVE('',#13767,#13768,#7129,.T.) ;
#17246=EDGE_CURVE('',#13768,#13769,#7130,.T.) ;
#17247=EDGE_CURVE('',#13769,#13770,#7131,.T.) ;
#17248=EDGE_CURVE('',#13770,#13771,#7132,.T.) ;
#17249=EDGE_CURVE('',#13771,#13772,#7133,.T.) ;
#17250=EDGE_CURVE('',#13772,#13773,#7134,.T.) ;
#17251=EDGE_CURVE('',#13773,#13774,#7135,.T.) ;
#17252=EDGE_CURVE('',#13774,#13775,#7136,.T.) ;
#17253=EDGE_CURVE('',#13775,#13776,#7137,.T.) ;
#17254=EDGE_CURVE('',#13776,#13777,#7138,.T.) ;
#17255=EDGE_CURVE('',#13777,#13778,#7139,.T.) ;
#17256=EDGE_CURVE('',#13778,#13779,#7140,.T.) ;
#17257=EDGE_CURVE('',#13779,#13780,#7141,.T.) ;
#17258=EDGE_CURVE('',#13780,#13781,#7142,.T.) ;
#17259=EDGE_CURVE('',#13781,#13782,#7143,.T.) ;
#17260=EDGE_CURVE('',#13782,#13783,#7144,.T.) ;
#17261=EDGE_CURVE('',#13783,#13784,#7145,.T.) ;
#17262=EDGE_CURVE('',#13784,#13785,#7146,.T.) ;
#17263=EDGE_CURVE('',#13785,#13786,#7147,.T.) ;
#17264=EDGE_CURVE('',#13786,#13787,#7148,.T.) ;
#17265=EDGE_CURVE('',#13787,#13788,#7149,.T.) ;
#17266=EDGE_CURVE('',#13788,#13789,#7150,.T.) ;
#17267=EDGE_CURVE('',#13789,#13790,#7151,.T.) ;
#17268=EDGE_CURVE('',#13790,#13791,#7152,.T.) ;
#17269=EDGE_CURVE('',#13791,#13792,#7153,.T.) ;
#17270=EDGE_CURVE('',#13792,#13793,#7154,.T.) ;
#17271=EDGE_CURVE('',#13793,#13794,#7155,.T.) ;
#17272=EDGE_CURVE('',#13794,#13795,#7156,.T.) ;
#17273=EDGE_CURVE('',#13795,#13796,#7157,.T.) ;
#17274=EDGE_CURVE('',#13796,#13797,#7158,.T.) ;
#17275=EDGE_CURVE('',#13797,#13798,#7159,.T.) ;
#17276=EDGE_CURVE('',#13798,#13799,#7160,.T.) ;
#17277=EDGE_CURVE('',#13799,#13800,#7161,.T.) ;
#17278=EDGE_CURVE('',#13800,#13801,#7162,.T.) ;
#17279=EDGE_CURVE('',#13801,#13802,#7163,.T.) ;
#17280=EDGE_CURVE('',#13802,#13803,#7164,.T.) ;
#17281=EDGE_CURVE('',#13803,#13804,#7165,.T.) ;
#17282=EDGE_CURVE('',#13804,#13805,#7166,.T.) ;
#17283=EDGE_CURVE('',#13764,#13805,#7167,.T.) ;
#17284=EDGE_CURVE('',#13732,#13762,#7168,.T.) ;
#17285=EDGE_CURVE('',#13700,#13730,#7169,.T.) ;
#17286=EDGE_CURVE('',#13806,#13806,#11304,.T.) ;
#17287=EDGE_CURVE('',#13806,#13807,#11305,.T.) ;
#17288=EDGE_CURVE('',#13807,#13807,#11306,.T.) ;
#17289=EDGE_CURVE('',#13808,#13808,#11307,.T.) ;
#17290=EDGE_CURVE('',#13808,#13806,#7170,.T.) ;
#17291=EDGE_CURVE('',#13809,#13810,#7171,.T.) ;
#17292=EDGE_CURVE('',#13811,#13809,#7172,.T.) ;
#17293=EDGE_CURVE('',#13812,#13811,#7173,.T.) ;
#17294=EDGE_CURVE('',#13810,#13812,#7174,.T.) ;
#17295=EDGE_CURVE('',#13813,#13814,#7175,.T.) ;
#17296=EDGE_CURVE('',#13815,#13814,#11308,.T.) ;
#17297=EDGE_CURVE('',#13815,#13816,#7176,.T.) ;
#17298=EDGE_CURVE('',#13817,#13816,#11309,.T.) ;
#17299=EDGE_CURVE('',#13817,#13818,#7177,.T.) ;
#17300=EDGE_CURVE('',#13819,#13818,#11310,.T.) ;
#17301=EDGE_CURVE('',#13819,#13820,#7178,.T.) ;
#17302=EDGE_CURVE('',#13813,#13820,#11311,.T.) ;
#17303=EDGE_CURVE('',#13821,#13821,#11312,.T.) ;
#17304=EDGE_CURVE('',#13821,#13822,#11313,.T.) ;
#17305=EDGE_CURVE('',#13822,#13822,#11314,.T.) ;
#17306=EDGE_CURVE('',#13823,#13823,#11315,.T.) ;
#17307=EDGE_CURVE('',#13823,#13821,#7179,.T.) ;
#17308=EDGE_CURVE('',#13824,#13825,#7180,.T.) ;
#17309=EDGE_CURVE('',#13826,#13824,#7181,.T.) ;
#17310=EDGE_CURVE('',#13827,#13826,#7182,.T.) ;
#17311=EDGE_CURVE('',#13825,#13827,#7183,.T.) ;
#17312=EDGE_CURVE('',#13828,#13829,#7184,.T.) ;
#17313=EDGE_CURVE('',#13830,#13829,#11316,.T.) ;
#17314=EDGE_CURVE('',#13830,#13831,#7185,.T.) ;
#17315=EDGE_CURVE('',#13832,#13831,#11317,.T.) ;
#17316=EDGE_CURVE('',#13832,#13833,#7186,.T.) ;
#17317=EDGE_CURVE('',#13834,#13833,#11318,.T.) ;
#17318=EDGE_CURVE('',#13834,#13835,#7187,.T.) ;
#17319=EDGE_CURVE('',#13828,#13835,#11319,.T.) ;
#17320=EDGE_CURVE('',#13836,#13836,#11320,.T.) ;
#17321=EDGE_CURVE('',#13836,#13837,#11321,.T.) ;
#17322=EDGE_CURVE('',#13837,#13837,#11322,.T.) ;
#17323=EDGE_CURVE('',#13838,#13838,#11323,.T.) ;
#17324=EDGE_CURVE('',#13838,#13836,#7188,.T.) ;
#17325=EDGE_CURVE('',#13839,#13840,#7189,.T.) ;
#17326=EDGE_CURVE('',#13841,#13839,#7190,.T.) ;
#17327=EDGE_CURVE('',#13842,#13841,#7191,.T.) ;
#17328=EDGE_CURVE('',#13840,#13842,#7192,.T.) ;
#17329=EDGE_CURVE('',#13843,#13844,#7193,.T.) ;
#17330=EDGE_CURVE('',#13845,#13844,#11324,.T.) ;
#17331=EDGE_CURVE('',#13845,#13846,#7194,.T.) ;
#17332=EDGE_CURVE('',#13847,#13846,#11325,.T.) ;
#17333=EDGE_CURVE('',#13847,#13848,#7195,.T.) ;
#17334=EDGE_CURVE('',#13849,#13848,#11326,.T.) ;
#17335=EDGE_CURVE('',#13849,#13850,#7196,.T.) ;
#17336=EDGE_CURVE('',#13843,#13850,#11327,.T.) ;
#17337=EDGE_CURVE('',#13851,#13851,#11328,.T.) ;
#17338=EDGE_CURVE('',#13851,#13852,#11329,.T.) ;
#17339=EDGE_CURVE('',#13852,#13852,#11330,.T.) ;
#17340=EDGE_CURVE('',#13853,#13853,#11331,.T.) ;
#17341=EDGE_CURVE('',#13853,#13851,#7197,.T.) ;
#17342=EDGE_CURVE('',#13854,#13855,#7198,.T.) ;
#17343=EDGE_CURVE('',#13856,#13854,#7199,.T.) ;
#17344=EDGE_CURVE('',#13857,#13856,#7200,.T.) ;
#17345=EDGE_CURVE('',#13855,#13857,#7201,.T.) ;
#17346=EDGE_CURVE('',#13858,#13859,#7202,.T.) ;
#17347=EDGE_CURVE('',#13860,#13859,#11332,.T.) ;
#17348=EDGE_CURVE('',#13860,#13861,#7203,.T.) ;
#17349=EDGE_CURVE('',#13862,#13861,#11333,.T.) ;
#17350=EDGE_CURVE('',#13862,#13863,#7204,.T.) ;
#17351=EDGE_CURVE('',#13864,#13863,#11334,.T.) ;
#17352=EDGE_CURVE('',#13864,#13865,#7205,.T.) ;
#17353=EDGE_CURVE('',#13858,#13865,#11335,.T.) ;
#17354=EDGE_CURVE('',#13866,#13866,#11336,.T.) ;
#17355=EDGE_CURVE('',#13866,#13867,#11337,.T.) ;
#17356=EDGE_CURVE('',#13867,#13867,#11338,.T.) ;
#17357=EDGE_CURVE('',#13868,#13868,#11339,.T.) ;
#17358=EDGE_CURVE('',#13868,#13866,#7206,.T.) ;
#17359=EDGE_CURVE('',#13869,#13870,#7207,.T.) ;
#17360=EDGE_CURVE('',#13871,#13869,#7208,.T.) ;
#17361=EDGE_CURVE('',#13872,#13871,#7209,.T.) ;
#17362=EDGE_CURVE('',#13870,#13872,#7210,.T.) ;
#17363=EDGE_CURVE('',#13873,#13874,#7211,.T.) ;
#17364=EDGE_CURVE('',#13875,#13874,#11340,.T.) ;
#17365=EDGE_CURVE('',#13875,#13876,#7212,.T.) ;
#17366=EDGE_CURVE('',#13877,#13876,#11341,.T.) ;
#17367=EDGE_CURVE('',#13877,#13878,#7213,.T.) ;
#17368=EDGE_CURVE('',#13879,#13878,#11342,.T.) ;
#17369=EDGE_CURVE('',#13879,#13880,#7214,.T.) ;
#17370=EDGE_CURVE('',#13873,#13880,#11343,.T.) ;
#17371=EDGE_CURVE('',#13881,#13881,#11344,.T.) ;
#17372=EDGE_CURVE('',#13881,#13882,#11345,.T.) ;
#17373=EDGE_CURVE('',#13882,#13882,#11346,.T.) ;
#17374=EDGE_CURVE('',#13883,#13883,#11347,.T.) ;
#17375=EDGE_CURVE('',#13883,#13881,#7215,.T.) ;
#17376=EDGE_CURVE('',#13884,#13885,#7216,.T.) ;
#17377=EDGE_CURVE('',#13886,#13884,#7217,.T.) ;
#17378=EDGE_CURVE('',#13887,#13886,#7218,.T.) ;
#17379=EDGE_CURVE('',#13885,#13887,#7219,.T.) ;
#17380=EDGE_CURVE('',#13888,#13889,#7220,.T.) ;
#17381=EDGE_CURVE('',#13890,#13889,#11348,.T.) ;
#17382=EDGE_CURVE('',#13890,#13891,#7221,.T.) ;
#17383=EDGE_CURVE('',#13892,#13891,#11349,.T.) ;
#17384=EDGE_CURVE('',#13892,#13893,#7222,.T.) ;
#17385=EDGE_CURVE('',#13894,#13893,#11350,.T.) ;
#17386=EDGE_CURVE('',#13894,#13895,#7223,.T.) ;
#17387=EDGE_CURVE('',#13888,#13895,#11351,.T.) ;
#17388=EDGE_CURVE('',#13896,#13896,#11352,.T.) ;
#17389=EDGE_CURVE('',#13896,#13897,#11353,.T.) ;
#17390=EDGE_CURVE('',#13897,#13897,#11354,.T.) ;
#17391=EDGE_CURVE('',#13898,#13898,#11355,.T.) ;
#17392=EDGE_CURVE('',#13898,#13896,#7224,.T.) ;
#17393=EDGE_CURVE('',#13899,#13900,#7225,.T.) ;
#17394=EDGE_CURVE('',#13901,#13899,#7226,.T.) ;
#17395=EDGE_CURVE('',#13902,#13901,#7227,.T.) ;
#17396=EDGE_CURVE('',#13900,#13902,#7228,.T.) ;
#17397=EDGE_CURVE('',#13903,#13904,#7229,.T.) ;
#17398=EDGE_CURVE('',#13905,#13904,#11356,.T.) ;
#17399=EDGE_CURVE('',#13905,#13906,#7230,.T.) ;
#17400=EDGE_CURVE('',#13907,#13906,#11357,.T.) ;
#17401=EDGE_CURVE('',#13907,#13908,#7231,.T.) ;
#17402=EDGE_CURVE('',#13909,#13908,#11358,.T.) ;
#17403=EDGE_CURVE('',#13909,#13910,#7232,.T.) ;
#17404=EDGE_CURVE('',#13903,#13910,#11359,.T.) ;
#17405=EDGE_CURVE('',#13911,#13911,#11360,.T.) ;
#17406=EDGE_CURVE('',#13911,#13912,#11361,.T.) ;
#17407=EDGE_CURVE('',#13912,#13912,#11362,.T.) ;
#17408=EDGE_CURVE('',#13913,#13913,#11363,.T.) ;
#17409=EDGE_CURVE('',#13913,#13911,#7233,.T.) ;
#17410=EDGE_CURVE('',#13914,#13915,#7234,.T.) ;
#17411=EDGE_CURVE('',#13916,#13914,#7235,.T.) ;
#17412=EDGE_CURVE('',#13917,#13916,#7236,.T.) ;
#17413=EDGE_CURVE('',#13915,#13917,#7237,.T.) ;
#17414=EDGE_CURVE('',#13918,#13919,#7238,.T.) ;
#17415=EDGE_CURVE('',#13920,#13919,#11364,.T.) ;
#17416=EDGE_CURVE('',#13920,#13921,#7239,.T.) ;
#17417=EDGE_CURVE('',#13922,#13921,#11365,.T.) ;
#17418=EDGE_CURVE('',#13922,#13923,#7240,.T.) ;
#17419=EDGE_CURVE('',#13924,#13923,#11366,.T.) ;
#17420=EDGE_CURVE('',#13924,#13925,#7241,.T.) ;
#17421=EDGE_CURVE('',#13918,#13925,#11367,.T.) ;
#17422=EDGE_CURVE('',#13926,#13926,#11368,.T.) ;
#17423=EDGE_CURVE('',#13926,#13927,#11369,.T.) ;
#17424=EDGE_CURVE('',#13927,#13927,#11370,.T.) ;
#17425=EDGE_CURVE('',#13928,#13929,#7242,.T.) ;
#17426=EDGE_CURVE('',#13930,#13928,#7243,.T.) ;
#17427=EDGE_CURVE('',#13931,#13930,#7244,.T.) ;
#17428=EDGE_CURVE('',#13929,#13931,#7245,.T.) ;
#17429=EDGE_CURVE('',#13932,#13933,#7246,.T.) ;
#17430=EDGE_CURVE('',#13934,#13932,#11371,.T.) ;
#17431=EDGE_CURVE('',#13935,#13934,#7247,.T.) ;
#17432=EDGE_CURVE('',#13936,#13935,#11372,.T.) ;
#17433=EDGE_CURVE('',#13937,#13936,#7248,.T.) ;
#17434=EDGE_CURVE('',#13938,#13937,#11373,.T.) ;
#17435=EDGE_CURVE('',#13939,#13938,#7249,.T.) ;
#17436=EDGE_CURVE('',#13933,#13939,#11374,.T.) ;
#17437=EDGE_CURVE('',#13940,#13940,#11375,.F.) ;
#17438=EDGE_CURVE('',#13940,#13926,#7250,.T.) ;
#17439=EDGE_CURVE('',#13941,#13941,#11376,.T.) ;
#17440=EDGE_CURVE('',#13942,#13942,#11377,.T.) ;
#17441=EDGE_CURVE('',#13943,#13943,#11378,.T.) ;
#17442=EDGE_CURVE('',#13944,#13944,#11379,.T.) ;
#17443=EDGE_CURVE('',#13945,#13945,#11380,.T.) ;
#17444=EDGE_CURVE('',#13946,#13946,#11381,.T.) ;
#17445=EDGE_CURVE('',#13947,#13947,#11382,.T.) ;
#17446=EDGE_CURVE('',#13948,#13948,#11383,.T.) ;
#17447=EDGE_CURVE('',#13813,#13949,#11384,.T.) ;
#17448=EDGE_CURVE('',#13949,#13950,#7251,.T.) ;
#17449=EDGE_CURVE('',#13950,#13814,#11385,.T.) ;
#17450=EDGE_CURVE('',#13951,#13815,#11386,.T.) ;
#17451=EDGE_CURVE('',#13951,#13950,#11387,.T.) ;
#17452=EDGE_CURVE('',#13952,#13816,#11388,.T.) ;
#17453=EDGE_CURVE('',#13951,#13952,#7252,.T.) ;
#17454=EDGE_CURVE('',#13953,#13817,#11389,.T.) ;
#17455=EDGE_CURVE('',#13952,#13953,#11390,.T.) ;
#17456=EDGE_CURVE('',#13954,#13818,#11391,.T.) ;
#17457=EDGE_CURVE('',#13953,#13954,#7253,.T.) ;
#17458=EDGE_CURVE('',#13955,#13819,#11392,.T.) ;
#17459=EDGE_CURVE('',#13955,#13954,#11393,.T.) ;
#17460=EDGE_CURVE('',#13956,#13820,#11394,.T.) ;
#17461=EDGE_CURVE('',#13955,#13956,#7254,.T.) ;
#17462=EDGE_CURVE('',#13956,#13949,#11395,.T.) ;
#17463=EDGE_CURVE('',#13957,#13952,#7255,.T.) ;
#17464=EDGE_CURVE('',#13958,#13957,#11396,.T.) ;
#17465=EDGE_CURVE('',#13953,#13958,#7256,.T.) ;
#17466=EDGE_CURVE('',#13951,#13959,#7257,.T.) ;
#17467=EDGE_CURVE('',#13959,#13960,#11397,.T.) ;
#17468=EDGE_CURVE('',#13960,#13961,#7258,.T.) ;
#17469=EDGE_CURVE('',#13961,#13962,#7259,.T.) ;
#17470=EDGE_CURVE('',#13963,#13962,#7260,.T.) ;
#17471=EDGE_CURVE('',#13963,#13964,#7261,.T.) ;
#17472=EDGE_CURVE('',#13964,#13965,#7262,.T.) ;
#17473=EDGE_CURVE('',#13965,#13957,#11398,.T.) ;
#17474=EDGE_CURVE('',#13966,#13950,#7263,.T.) ;
#17475=EDGE_CURVE('',#13959,#13966,#11399,.T.) ;
#17476=EDGE_CURVE('',#13949,#13967,#7264,.T.) ;
#17477=EDGE_CURVE('',#13967,#13966,#7265,.T.) ;
#17478=EDGE_CURVE('',#13828,#13968,#11400,.T.) ;
#17479=EDGE_CURVE('',#13968,#13969,#7266,.T.) ;
#17480=EDGE_CURVE('',#13969,#13829,#11401,.T.) ;
#17481=EDGE_CURVE('',#13970,#13830,#11402,.T.) ;
#17482=EDGE_CURVE('',#13970,#13969,#11403,.T.) ;
#17483=EDGE_CURVE('',#13971,#13831,#11404,.T.) ;
#17484=EDGE_CURVE('',#13970,#13971,#7267,.T.) ;
#17485=EDGE_CURVE('',#13972,#13832,#11405,.T.) ;
#17486=EDGE_CURVE('',#13971,#13972,#11406,.T.) ;
#17487=EDGE_CURVE('',#13973,#13833,#11407,.T.) ;
#17488=EDGE_CURVE('',#13972,#13973,#7268,.T.) ;
#17489=EDGE_CURVE('',#13974,#13834,#11408,.T.) ;
#17490=EDGE_CURVE('',#13974,#13973,#11409,.T.) ;
#17491=EDGE_CURVE('',#13975,#13835,#11410,.T.) ;
#17492=EDGE_CURVE('',#13974,#13975,#7269,.T.) ;
#17493=EDGE_CURVE('',#13975,#13968,#11411,.T.) ;
#17494=EDGE_CURVE('',#13976,#13971,#7270,.T.) ;
#17495=EDGE_CURVE('',#13977,#13976,#11412,.T.) ;
#17496=EDGE_CURVE('',#13972,#13977,#7271,.T.) ;
#17497=EDGE_CURVE('',#13970,#13978,#7272,.T.) ;
#17498=EDGE_CURVE('',#13978,#13979,#11413,.T.) ;
#17499=EDGE_CURVE('',#13979,#13980,#7273,.T.) ;
#17500=EDGE_CURVE('',#13980,#13981,#7274,.T.) ;
#17501=EDGE_CURVE('',#13982,#13981,#7275,.T.) ;
#17502=EDGE_CURVE('',#13982,#13983,#7276,.T.) ;
#17503=EDGE_CURVE('',#13983,#13984,#7277,.T.) ;
#17504=EDGE_CURVE('',#13984,#13976,#11414,.T.) ;
#17505=EDGE_CURVE('',#13985,#13969,#7278,.T.) ;
#17506=EDGE_CURVE('',#13978,#13985,#11415,.T.) ;
#17507=EDGE_CURVE('',#13968,#13986,#7279,.T.) ;
#17508=EDGE_CURVE('',#13986,#13985,#7280,.T.) ;
#17509=EDGE_CURVE('',#13843,#13987,#11416,.T.) ;
#17510=EDGE_CURVE('',#13987,#13988,#7281,.T.) ;
#17511=EDGE_CURVE('',#13988,#13844,#11417,.T.) ;
#17512=EDGE_CURVE('',#13989,#13845,#11418,.T.) ;
#17513=EDGE_CURVE('',#13989,#13988,#11419,.T.) ;
#17514=EDGE_CURVE('',#13990,#13846,#11420,.T.) ;
#17515=EDGE_CURVE('',#13989,#13990,#7282,.T.) ;
#17516=EDGE_CURVE('',#13991,#13847,#11421,.T.) ;
#17517=EDGE_CURVE('',#13990,#13991,#11422,.T.) ;
#17518=EDGE_CURVE('',#13992,#13848,#11423,.T.) ;
#17519=EDGE_CURVE('',#13991,#13992,#7283,.T.) ;
#17520=EDGE_CURVE('',#13993,#13849,#11424,.T.) ;
#17521=EDGE_CURVE('',#13993,#13992,#11425,.T.) ;
#17522=EDGE_CURVE('',#13994,#13850,#11426,.T.) ;
#17523=EDGE_CURVE('',#13993,#13994,#7284,.T.) ;
#17524=EDGE_CURVE('',#13994,#13987,#11427,.T.) ;
#17525=EDGE_CURVE('',#13995,#13990,#7285,.T.) ;
#17526=EDGE_CURVE('',#13996,#13995,#11428,.T.) ;
#17527=EDGE_CURVE('',#13991,#13996,#7286,.T.) ;
#17528=EDGE_CURVE('',#13989,#13997,#7287,.T.) ;
#17529=EDGE_CURVE('',#13997,#13998,#11429,.T.) ;
#17530=EDGE_CURVE('',#13998,#13999,#7288,.T.) ;
#17531=EDGE_CURVE('',#13999,#14000,#7289,.T.) ;
#17532=EDGE_CURVE('',#14001,#14000,#7290,.T.) ;
#17533=EDGE_CURVE('',#14001,#14002,#7291,.T.) ;
#17534=EDGE_CURVE('',#14002,#14003,#7292,.T.) ;
#17535=EDGE_CURVE('',#14003,#13995,#11430,.T.) ;
#17536=EDGE_CURVE('',#14004,#13988,#7293,.T.) ;
#17537=EDGE_CURVE('',#13997,#14004,#11431,.T.) ;
#17538=EDGE_CURVE('',#13987,#14005,#7294,.T.) ;
#17539=EDGE_CURVE('',#14005,#14004,#7295,.T.) ;
#17540=EDGE_CURVE('',#13858,#14006,#11432,.T.) ;
#17541=EDGE_CURVE('',#14006,#14007,#7296,.T.) ;
#17542=EDGE_CURVE('',#14007,#13859,#11433,.T.) ;
#17543=EDGE_CURVE('',#14008,#13860,#11434,.T.) ;
#17544=EDGE_CURVE('',#14008,#14007,#11435,.T.) ;
#17545=EDGE_CURVE('',#14009,#13861,#11436,.T.) ;
#17546=EDGE_CURVE('',#14008,#14009,#7297,.T.) ;
#17547=EDGE_CURVE('',#14010,#13862,#11437,.T.) ;
#17548=EDGE_CURVE('',#14009,#14010,#11438,.T.) ;
#17549=EDGE_CURVE('',#14011,#13863,#11439,.T.) ;
#17550=EDGE_CURVE('',#14010,#14011,#7298,.T.) ;
#17551=EDGE_CURVE('',#14012,#13864,#11440,.T.) ;
#17552=EDGE_CURVE('',#14012,#14011,#11441,.T.) ;
#17553=EDGE_CURVE('',#14013,#13865,#11442,.T.) ;
#17554=EDGE_CURVE('',#14012,#14013,#7299,.T.) ;
#17555=EDGE_CURVE('',#14013,#14006,#11443,.T.) ;
#17556=EDGE_CURVE('',#14014,#14009,#7300,.T.) ;
#17557=EDGE_CURVE('',#14015,#14014,#11444,.T.) ;
#17558=EDGE_CURVE('',#14010,#14015,#7301,.T.) ;
#17559=EDGE_CURVE('',#14008,#14016,#7302,.T.) ;
#17560=EDGE_CURVE('',#14016,#14017,#11445,.T.) ;
#17561=EDGE_CURVE('',#14017,#14018,#7303,.T.) ;
#17562=EDGE_CURVE('',#14018,#14019,#7304,.T.) ;
#17563=EDGE_CURVE('',#14020,#14019,#7305,.T.) ;
#17564=EDGE_CURVE('',#14020,#14021,#7306,.T.) ;
#17565=EDGE_CURVE('',#14021,#14022,#7307,.T.) ;
#17566=EDGE_CURVE('',#14022,#14014,#11446,.T.) ;
#17567=EDGE_CURVE('',#14023,#14007,#7308,.T.) ;
#17568=EDGE_CURVE('',#14016,#14023,#11447,.T.) ;
#17569=EDGE_CURVE('',#14006,#14024,#7309,.T.) ;
#17570=EDGE_CURVE('',#14024,#14023,#7310,.T.) ;
#17571=EDGE_CURVE('',#13873,#14025,#11448,.T.) ;
#17572=EDGE_CURVE('',#14025,#14026,#7311,.T.) ;
#17573=EDGE_CURVE('',#14026,#13874,#11449,.T.) ;
#17574=EDGE_CURVE('',#14027,#13875,#11450,.T.) ;
#17575=EDGE_CURVE('',#14027,#14026,#11451,.T.) ;
#17576=EDGE_CURVE('',#14028,#13876,#11452,.T.) ;
#17577=EDGE_CURVE('',#14027,#14028,#7312,.T.) ;
#17578=EDGE_CURVE('',#14029,#13877,#11453,.T.) ;
#17579=EDGE_CURVE('',#14028,#14029,#11454,.T.) ;
#17580=EDGE_CURVE('',#14030,#13878,#11455,.T.) ;
#17581=EDGE_CURVE('',#14029,#14030,#7313,.T.) ;
#17582=EDGE_CURVE('',#14031,#13879,#11456,.T.) ;
#17583=EDGE_CURVE('',#14031,#14030,#11457,.T.) ;
#17584=EDGE_CURVE('',#14032,#13880,#11458,.T.) ;
#17585=EDGE_CURVE('',#14031,#14032,#7314,.T.) ;
#17586=EDGE_CURVE('',#14032,#14025,#11459,.T.) ;
#17587=EDGE_CURVE('',#14033,#14028,#7315,.T.) ;
#17588=EDGE_CURVE('',#14034,#14033,#11460,.T.) ;
#17589=EDGE_CURVE('',#14029,#14034,#7316,.T.) ;
#17590=EDGE_CURVE('',#14027,#14035,#7317,.T.) ;
#17591=EDGE_CURVE('',#14035,#14036,#11461,.T.) ;
#17592=EDGE_CURVE('',#14036,#14037,#7318,.T.) ;
#17593=EDGE_CURVE('',#14037,#14038,#7319,.T.) ;
#17594=EDGE_CURVE('',#14039,#14038,#7320,.T.) ;
#17595=EDGE_CURVE('',#14039,#14040,#7321,.T.) ;
#17596=EDGE_CURVE('',#14040,#14041,#7322,.T.) ;
#17597=EDGE_CURVE('',#14041,#14033,#11462,.T.) ;
#17598=EDGE_CURVE('',#14042,#14026,#7323,.T.) ;
#17599=EDGE_CURVE('',#14035,#14042,#11463,.T.) ;
#17600=EDGE_CURVE('',#14025,#14043,#7324,.T.) ;
#17601=EDGE_CURVE('',#14043,#14042,#7325,.T.) ;
#17602=EDGE_CURVE('',#13888,#14044,#11464,.T.) ;
#17603=EDGE_CURVE('',#14044,#14045,#7326,.T.) ;
#17604=EDGE_CURVE('',#14045,#13889,#11465,.T.) ;
#17605=EDGE_CURVE('',#14046,#13890,#11466,.T.) ;
#17606=EDGE_CURVE('',#14046,#14045,#11467,.T.) ;
#17607=EDGE_CURVE('',#14047,#13891,#11468,.T.) ;
#17608=EDGE_CURVE('',#14046,#14047,#7327,.T.) ;
#17609=EDGE_CURVE('',#14048,#13892,#11469,.T.) ;
#17610=EDGE_CURVE('',#14047,#14048,#11470,.T.) ;
#17611=EDGE_CURVE('',#14049,#13893,#11471,.T.) ;
#17612=EDGE_CURVE('',#14048,#14049,#7328,.T.) ;
#17613=EDGE_CURVE('',#14050,#13894,#11472,.T.) ;
#17614=EDGE_CURVE('',#14050,#14049,#11473,.T.) ;
#17615=EDGE_CURVE('',#14051,#13895,#11474,.T.) ;
#17616=EDGE_CURVE('',#14050,#14051,#7329,.T.) ;
#17617=EDGE_CURVE('',#14051,#14044,#11475,.T.) ;
#17618=EDGE_CURVE('',#14052,#14047,#7330,.T.) ;
#17619=EDGE_CURVE('',#14053,#14052,#11476,.T.) ;
#17620=EDGE_CURVE('',#14048,#14053,#7331,.T.) ;
#17621=EDGE_CURVE('',#14046,#14054,#7332,.T.) ;
#17622=EDGE_CURVE('',#14054,#14055,#11477,.T.) ;
#17623=EDGE_CURVE('',#14055,#14056,#7333,.T.) ;
#17624=EDGE_CURVE('',#14056,#14057,#7334,.T.) ;
#17625=EDGE_CURVE('',#14058,#14057,#7335,.T.) ;
#17626=EDGE_CURVE('',#14058,#14059,#7336,.T.) ;
#17627=EDGE_CURVE('',#14059,#14060,#7337,.T.) ;
#17628=EDGE_CURVE('',#14060,#14052,#11478,.T.) ;
#17629=EDGE_CURVE('',#14061,#14045,#7338,.T.) ;
#17630=EDGE_CURVE('',#14054,#14061,#11479,.T.) ;
#17631=EDGE_CURVE('',#14044,#14062,#7339,.T.) ;
#17632=EDGE_CURVE('',#14062,#14061,#7340,.T.) ;
#17633=EDGE_CURVE('',#13903,#14063,#11480,.T.) ;
#17634=EDGE_CURVE('',#14063,#14064,#7341,.T.) ;
#17635=EDGE_CURVE('',#14064,#13904,#11481,.T.) ;
#17636=EDGE_CURVE('',#14065,#13905,#11482,.T.) ;
#17637=EDGE_CURVE('',#14065,#14064,#11483,.T.) ;
#17638=EDGE_CURVE('',#14066,#13906,#11484,.T.) ;
#17639=EDGE_CURVE('',#14065,#14066,#7342,.T.) ;
#17640=EDGE_CURVE('',#14067,#13907,#11485,.T.) ;
#17641=EDGE_CURVE('',#14066,#14067,#11486,.T.) ;
#17642=EDGE_CURVE('',#14068,#13908,#11487,.T.) ;
#17643=EDGE_CURVE('',#14067,#14068,#7343,.T.) ;
#17644=EDGE_CURVE('',#14069,#13909,#11488,.T.) ;
#17645=EDGE_CURVE('',#14069,#14068,#11489,.T.) ;
#17646=EDGE_CURVE('',#14070,#13910,#11490,.T.) ;
#17647=EDGE_CURVE('',#14069,#14070,#7344,.T.) ;
#17648=EDGE_CURVE('',#14070,#14063,#11491,.T.) ;
#17649=EDGE_CURVE('',#14071,#14066,#7345,.T.) ;
#17650=EDGE_CURVE('',#14072,#14071,#11492,.T.) ;
#17651=EDGE_CURVE('',#14067,#14072,#7346,.T.) ;
#17652=EDGE_CURVE('',#14065,#14073,#7347,.T.) ;
#17653=EDGE_CURVE('',#14073,#14074,#11493,.T.) ;
#17654=EDGE_CURVE('',#14074,#14075,#7348,.T.) ;
#17655=EDGE_CURVE('',#14075,#14076,#7349,.T.) ;
#17656=EDGE_CURVE('',#14077,#14076,#7350,.T.) ;
#17657=EDGE_CURVE('',#14077,#14078,#7351,.T.) ;
#17658=EDGE_CURVE('',#14078,#14079,#7352,.T.) ;
#17659=EDGE_CURVE('',#14079,#14071,#11494,.T.) ;
#17660=EDGE_CURVE('',#14080,#14064,#7353,.T.) ;
#17661=EDGE_CURVE('',#14073,#14080,#11495,.T.) ;
#17662=EDGE_CURVE('',#14063,#14081,#7354,.T.) ;
#17663=EDGE_CURVE('',#14081,#14080,#7355,.T.) ;
#17664=EDGE_CURVE('',#13918,#14082,#11496,.T.) ;
#17665=EDGE_CURVE('',#14082,#14083,#7356,.T.) ;
#17666=EDGE_CURVE('',#14083,#13919,#11497,.T.) ;
#17667=EDGE_CURVE('',#14084,#13920,#11498,.T.) ;
#17668=EDGE_CURVE('',#14084,#14083,#11499,.T.) ;
#17669=EDGE_CURVE('',#14085,#13921,#11500,.T.) ;
#17670=EDGE_CURVE('',#14084,#14085,#7357,.T.) ;
#17671=EDGE_CURVE('',#14086,#13922,#11501,.T.) ;
#17672=EDGE_CURVE('',#14085,#14086,#11502,.T.) ;
#17673=EDGE_CURVE('',#14087,#13923,#11503,.T.) ;
#17674=EDGE_CURVE('',#14086,#14087,#7358,.T.) ;
#17675=EDGE_CURVE('',#14088,#13924,#11504,.T.) ;
#17676=EDGE_CURVE('',#14088,#14087,#11505,.T.) ;
#17677=EDGE_CURVE('',#14089,#13925,#11506,.T.) ;
#17678=EDGE_CURVE('',#14088,#14089,#7359,.T.) ;
#17679=EDGE_CURVE('',#14089,#14082,#11507,.T.) ;
#17680=EDGE_CURVE('',#14090,#14085,#7360,.T.) ;
#17681=EDGE_CURVE('',#14091,#14090,#11508,.T.) ;
#17682=EDGE_CURVE('',#14086,#14091,#7361,.T.) ;
#17683=EDGE_CURVE('',#14084,#14092,#7362,.T.) ;
#17684=EDGE_CURVE('',#14092,#14093,#11509,.T.) ;
#17685=EDGE_CURVE('',#14093,#14094,#7363,.T.) ;
#17686=EDGE_CURVE('',#14094,#14095,#7364,.T.) ;
#17687=EDGE_CURVE('',#14096,#14095,#7365,.T.) ;
#17688=EDGE_CURVE('',#14096,#14097,#7366,.T.) ;
#17689=EDGE_CURVE('',#14097,#14098,#7367,.T.) ;
#17690=EDGE_CURVE('',#14098,#14090,#11510,.T.) ;
#17691=EDGE_CURVE('',#14099,#14083,#7368,.T.) ;
#17692=EDGE_CURVE('',#14092,#14099,#11511,.T.) ;
#17693=EDGE_CURVE('',#14082,#14100,#7369,.T.) ;
#17694=EDGE_CURVE('',#14100,#14099,#7370,.T.) ;
#17695=EDGE_CURVE('',#13933,#14101,#11512,.T.) ;
#17696=EDGE_CURVE('',#14101,#14102,#7371,.T.) ;
#17697=EDGE_CURVE('',#14102,#13932,#11513,.T.) ;
#17698=EDGE_CURVE('',#14103,#13934,#11514,.T.) ;
#17699=EDGE_CURVE('',#14102,#14103,#11515,.T.) ;
#17700=EDGE_CURVE('',#14104,#13935,#11516,.T.) ;
#17701=EDGE_CURVE('',#14103,#14104,#7372,.T.) ;
#17702=EDGE_CURVE('',#14105,#13936,#11517,.T.) ;
#17703=EDGE_CURVE('',#14104,#14105,#11518,.T.) ;
#17704=EDGE_CURVE('',#14106,#13937,#11519,.T.) ;
#17705=EDGE_CURVE('',#14105,#14106,#7373,.T.) ;
#17706=EDGE_CURVE('',#14107,#13938,#11520,.T.) ;
#17707=EDGE_CURVE('',#14106,#14107,#11521,.T.) ;
#17708=EDGE_CURVE('',#14108,#13939,#11522,.T.) ;
#17709=EDGE_CURVE('',#14107,#14108,#7374,.T.) ;
#17710=EDGE_CURVE('',#14108,#14101,#11523,.T.) ;
#17711=EDGE_CURVE('',#14109,#14104,#7375,.T.) ;
#17712=EDGE_CURVE('',#14110,#14109,#11524,.T.) ;
#17713=EDGE_CURVE('',#14105,#14110,#7376,.T.) ;
#17714=EDGE_CURVE('',#14111,#14112,#7377,.T.) ;
#17715=EDGE_CURVE('',#14111,#14113,#7378,.T.) ;
#17716=EDGE_CURVE('',#14113,#14114,#7379,.T.) ;
#17717=EDGE_CURVE('',#14114,#14109,#11525,.T.) ;
#17718=EDGE_CURVE('',#14103,#14115,#7380,.T.) ;
#17719=EDGE_CURVE('',#14115,#14116,#11526,.T.) ;
#17720=EDGE_CURVE('',#14116,#14117,#7381,.T.) ;
#17721=EDGE_CURVE('',#14117,#14112,#7382,.T.) ;
#17722=EDGE_CURVE('',#14118,#14102,#7383,.T.) ;
#17723=EDGE_CURVE('',#14115,#14118,#11527,.T.) ;
#17724=EDGE_CURVE('',#14101,#14119,#7384,.T.) ;
#17725=EDGE_CURVE('',#14119,#14118,#7385,.T.) ;
#17726=EDGE_CURVE('',#14120,#14121,#11528,.T.) ;
#17727=EDGE_CURVE('',#14121,#14122,#7386,.T.) ;
#17728=EDGE_CURVE('',#14122,#14123,#11529,.T.) ;
#17729=EDGE_CURVE('',#14120,#14123,#7387,.T.) ;
#17730=EDGE_CURVE('',#14124,#14125,#11530,.T.) ;
#17731=EDGE_CURVE('',#14125,#14123,#11531,.T.) ;
#17732=EDGE_CURVE('',#14122,#14124,#11532,.T.) ;
#17733=EDGE_CURVE('',#14126,#14127,#11533,.T.) ;
#17734=EDGE_CURVE('',#14125,#14127,#7388,.T.) ;
#17735=EDGE_CURVE('',#14124,#14126,#7389,.T.) ;
#17736=EDGE_CURVE('',#14128,#14129,#11534,.T.) ;
#17737=EDGE_CURVE('',#14129,#14127,#11535,.T.) ;
#17738=EDGE_CURVE('',#14128,#14126,#11536,.T.) ;
#17739=EDGE_CURVE('',#14130,#14131,#11537,.T.) ;
#17740=EDGE_CURVE('',#14129,#14131,#7390,.T.) ;
#17741=EDGE_CURVE('',#14128,#14130,#7391,.T.) ;
#17742=EDGE_CURVE('',#14132,#14133,#11538,.T.) ;
#17743=EDGE_CURVE('',#14133,#14131,#11539,.T.) ;
#17744=EDGE_CURVE('',#14130,#14132,#11540,.T.) ;
#17745=EDGE_CURVE('',#14134,#14135,#11541,.T.) ;
#17746=EDGE_CURVE('',#14133,#14135,#7392,.T.) ;
#17747=EDGE_CURVE('',#14132,#14134,#7393,.T.) ;
#17748=EDGE_CURVE('',#14120,#14135,#11542,.T.) ;
#17749=EDGE_CURVE('',#14121,#14134,#11543,.T.) ;
#17750=EDGE_CURVE('',#14136,#14126,#7394,.T.) ;
#17751=EDGE_CURVE('',#14137,#14136,#11544,.F.) ;
#17752=EDGE_CURVE('',#14128,#14137,#7395,.T.) ;
#17753=EDGE_CURVE('',#14124,#14138,#7396,.T.) ;
#17754=EDGE_CURVE('',#14138,#14136,#7397,.T.) ;
#17755=EDGE_CURVE('',#14139,#14122,#7398,.T.) ;
#17756=EDGE_CURVE('',#14138,#14139,#11545,.F.) ;
#17757=EDGE_CURVE('',#14121,#14140,#7399,.T.) ;
#17758=EDGE_CURVE('',#14140,#14139,#7400,.T.) ;
#17759=EDGE_CURVE('',#14141,#14142,#11546,.T.) ;
#17760=EDGE_CURVE('',#14142,#14143,#7401,.T.) ;
#17761=EDGE_CURVE('',#14143,#14144,#11547,.T.) ;
#17762=EDGE_CURVE('',#14141,#14144,#7402,.T.) ;
#17763=EDGE_CURVE('',#14145,#14146,#11548,.T.) ;
#17764=EDGE_CURVE('',#14146,#14144,#11549,.T.) ;
#17765=EDGE_CURVE('',#14143,#14145,#11550,.T.) ;
#17766=EDGE_CURVE('',#14147,#14148,#11551,.T.) ;
#17767=EDGE_CURVE('',#14146,#14148,#7403,.T.) ;
#17768=EDGE_CURVE('',#14145,#14147,#7404,.T.) ;
#17769=EDGE_CURVE('',#14149,#14150,#11552,.T.) ;
#17770=EDGE_CURVE('',#14150,#14148,#11553,.T.) ;
#17771=EDGE_CURVE('',#14149,#14147,#11554,.T.) ;
#17772=EDGE_CURVE('',#14151,#14152,#11555,.T.) ;
#17773=EDGE_CURVE('',#14150,#14152,#7405,.T.) ;
#17774=EDGE_CURVE('',#14149,#14151,#7406,.T.) ;
#17775=EDGE_CURVE('',#14153,#14154,#11556,.T.) ;
#17776=EDGE_CURVE('',#14154,#14152,#11557,.T.) ;
#17777=EDGE_CURVE('',#14151,#14153,#11558,.T.) ;
#17778=EDGE_CURVE('',#14155,#14156,#11559,.T.) ;
#17779=EDGE_CURVE('',#14154,#14156,#7407,.T.) ;
#17780=EDGE_CURVE('',#14153,#14155,#7408,.T.) ;
#17781=EDGE_CURVE('',#14141,#14156,#11560,.T.) ;
#17782=EDGE_CURVE('',#14142,#14155,#11561,.T.) ;
#17783=EDGE_CURVE('',#14157,#14147,#7409,.T.) ;
#17784=EDGE_CURVE('',#14158,#14157,#11562,.F.) ;
#17785=EDGE_CURVE('',#14149,#14158,#7410,.T.) ;
#17786=EDGE_CURVE('',#14145,#14159,#7411,.T.) ;
#17787=EDGE_CURVE('',#14159,#14157,#7412,.T.) ;
#17788=EDGE_CURVE('',#14160,#14143,#7413,.T.) ;
#17789=EDGE_CURVE('',#14159,#14160,#11563,.F.) ;
#17790=EDGE_CURVE('',#14142,#14161,#7414,.T.) ;
#17791=EDGE_CURVE('',#14161,#14160,#7415,.T.) ;
#17792=EDGE_CURVE('',#14162,#14163,#11564,.T.) ;
#17793=EDGE_CURVE('',#14163,#14164,#7416,.T.) ;
#17794=EDGE_CURVE('',#14164,#14165,#11565,.T.) ;
#17795=EDGE_CURVE('',#14162,#14165,#7417,.T.) ;
#17796=EDGE_CURVE('',#14166,#14167,#11566,.T.) ;
#17797=EDGE_CURVE('',#14167,#14165,#11567,.T.) ;
#17798=EDGE_CURVE('',#14164,#14166,#11568,.T.) ;
#17799=EDGE_CURVE('',#14168,#14169,#11569,.T.) ;
#17800=EDGE_CURVE('',#14167,#14169,#7418,.T.) ;
#17801=EDGE_CURVE('',#14166,#14168,#7419,.T.) ;
#17802=EDGE_CURVE('',#14170,#14171,#11570,.T.) ;
#17803=EDGE_CURVE('',#14171,#14169,#11571,.T.) ;
#17804=EDGE_CURVE('',#14170,#14168,#11572,.T.) ;
#17805=EDGE_CURVE('',#14172,#14173,#11573,.T.) ;
#17806=EDGE_CURVE('',#14171,#14173,#7420,.T.) ;
#17807=EDGE_CURVE('',#14170,#14172,#7421,.T.) ;
#17808=EDGE_CURVE('',#14174,#14175,#11574,.T.) ;
#17809=EDGE_CURVE('',#14175,#14173,#11575,.T.) ;
#17810=EDGE_CURVE('',#14172,#14174,#11576,.T.) ;
#17811=EDGE_CURVE('',#14176,#14177,#11577,.T.) ;
#17812=EDGE_CURVE('',#14175,#14177,#7422,.T.) ;
#17813=EDGE_CURVE('',#14174,#14176,#7423,.T.) ;
#17814=EDGE_CURVE('',#14162,#14177,#11578,.T.) ;
#17815=EDGE_CURVE('',#14163,#14176,#11579,.T.) ;
#17816=EDGE_CURVE('',#14178,#14168,#7424,.T.) ;
#17817=EDGE_CURVE('',#14179,#14178,#11580,.F.) ;
#17818=EDGE_CURVE('',#14170,#14179,#7425,.T.) ;
#17819=EDGE_CURVE('',#14166,#14180,#7426,.T.) ;
#17820=EDGE_CURVE('',#14180,#14178,#7427,.T.) ;
#17821=EDGE_CURVE('',#14181,#14164,#7428,.T.) ;
#17822=EDGE_CURVE('',#14180,#14181,#11581,.F.) ;
#17823=EDGE_CURVE('',#14163,#14182,#7429,.T.) ;
#17824=EDGE_CURVE('',#14182,#14181,#7430,.T.) ;
#17825=EDGE_CURVE('',#14183,#14184,#11582,.T.) ;
#17826=EDGE_CURVE('',#14184,#14185,#7431,.T.) ;
#17827=EDGE_CURVE('',#14185,#14186,#11583,.T.) ;
#17828=EDGE_CURVE('',#14183,#14186,#7432,.T.) ;
#17829=EDGE_CURVE('',#14187,#14188,#11584,.T.) ;
#17830=EDGE_CURVE('',#14188,#14186,#11585,.T.) ;
#17831=EDGE_CURVE('',#14185,#14187,#11586,.T.) ;
#17832=EDGE_CURVE('',#14189,#14190,#11587,.T.) ;
#17833=EDGE_CURVE('',#14188,#14190,#7433,.T.) ;
#17834=EDGE_CURVE('',#14187,#14189,#7434,.T.) ;
#17835=EDGE_CURVE('',#14191,#14192,#11588,.T.) ;
#17836=EDGE_CURVE('',#14192,#14190,#11589,.T.) ;
#17837=EDGE_CURVE('',#14191,#14189,#11590,.T.) ;
#17838=EDGE_CURVE('',#14193,#14194,#11591,.T.) ;
#17839=EDGE_CURVE('',#14192,#14194,#7435,.T.) ;
#17840=EDGE_CURVE('',#14191,#14193,#7436,.T.) ;
#17841=EDGE_CURVE('',#14195,#14196,#11592,.T.) ;
#17842=EDGE_CURVE('',#14196,#14194,#11593,.T.) ;
#17843=EDGE_CURVE('',#14193,#14195,#11594,.T.) ;
#17844=EDGE_CURVE('',#14197,#14198,#11595,.T.) ;
#17845=EDGE_CURVE('',#14196,#14198,#7437,.T.) ;
#17846=EDGE_CURVE('',#14195,#14197,#7438,.T.) ;
#17847=EDGE_CURVE('',#14183,#14198,#11596,.T.) ;
#17848=EDGE_CURVE('',#14184,#14197,#11597,.T.) ;
#17849=EDGE_CURVE('',#14199,#14189,#7439,.T.) ;
#17850=EDGE_CURVE('',#14200,#14199,#11598,.F.) ;
#17851=EDGE_CURVE('',#14191,#14200,#7440,.T.) ;
#17852=EDGE_CURVE('',#14187,#14201,#7441,.T.) ;
#17853=EDGE_CURVE('',#14201,#14199,#7442,.T.) ;
#17854=EDGE_CURVE('',#14202,#14185,#7443,.T.) ;
#17855=EDGE_CURVE('',#14201,#14202,#11599,.F.) ;
#17856=EDGE_CURVE('',#14184,#14203,#7444,.T.) ;
#17857=EDGE_CURVE('',#14203,#14202,#7445,.T.) ;
#17858=EDGE_CURVE('',#14204,#14205,#11600,.T.) ;
#17859=EDGE_CURVE('',#14205,#14206,#7446,.T.) ;
#17860=EDGE_CURVE('',#14206,#14207,#11601,.T.) ;
#17861=EDGE_CURVE('',#14204,#14207,#7447,.T.) ;
#17862=EDGE_CURVE('',#14208,#14209,#11602,.T.) ;
#17863=EDGE_CURVE('',#14209,#14207,#11603,.T.) ;
#17864=EDGE_CURVE('',#14206,#14208,#11604,.T.) ;
#17865=EDGE_CURVE('',#14210,#14211,#11605,.T.) ;
#17866=EDGE_CURVE('',#14209,#14211,#7448,.T.) ;
#17867=EDGE_CURVE('',#14208,#14210,#7449,.T.) ;
#17868=EDGE_CURVE('',#14212,#14213,#11606,.T.) ;
#17869=EDGE_CURVE('',#14213,#14211,#11607,.T.) ;
#17870=EDGE_CURVE('',#14212,#14210,#11608,.T.) ;
#17871=EDGE_CURVE('',#14214,#14215,#11609,.T.) ;
#17872=EDGE_CURVE('',#14213,#14215,#7450,.T.) ;
#17873=EDGE_CURVE('',#14212,#14214,#7451,.T.) ;
#17874=EDGE_CURVE('',#14216,#14217,#11610,.T.) ;
#17875=EDGE_CURVE('',#14217,#14215,#11611,.T.) ;
#17876=EDGE_CURVE('',#14214,#14216,#11612,.T.) ;
#17877=EDGE_CURVE('',#14218,#14219,#11613,.T.) ;
#17878=EDGE_CURVE('',#14217,#14219,#7452,.T.) ;
#17879=EDGE_CURVE('',#14216,#14218,#7453,.T.) ;
#17880=EDGE_CURVE('',#14204,#14219,#11614,.T.) ;
#17881=EDGE_CURVE('',#14205,#14218,#11615,.T.) ;
#17882=EDGE_CURVE('',#14220,#14210,#7454,.T.) ;
#17883=EDGE_CURVE('',#14221,#14220,#11616,.F.) ;
#17884=EDGE_CURVE('',#14212,#14221,#7455,.T.) ;
#17885=EDGE_CURVE('',#14208,#14222,#7456,.T.) ;
#17886=EDGE_CURVE('',#14222,#14220,#7457,.T.) ;
#17887=EDGE_CURVE('',#14223,#14206,#7458,.T.) ;
#17888=EDGE_CURVE('',#14222,#14223,#11617,.F.) ;
#17889=EDGE_CURVE('',#14205,#14224,#7459,.T.) ;
#17890=EDGE_CURVE('',#14224,#14223,#7460,.T.) ;
#17891=EDGE_CURVE('',#14225,#14226,#11618,.T.) ;
#17892=EDGE_CURVE('',#14226,#14227,#7461,.T.) ;
#17893=EDGE_CURVE('',#14227,#14228,#11619,.T.) ;
#17894=EDGE_CURVE('',#14225,#14228,#7462,.T.) ;
#17895=EDGE_CURVE('',#14229,#14230,#11620,.T.) ;
#17896=EDGE_CURVE('',#14230,#14228,#11621,.T.) ;
#17897=EDGE_CURVE('',#14227,#14229,#11622,.T.) ;
#17898=EDGE_CURVE('',#14231,#14232,#11623,.T.) ;
#17899=EDGE_CURVE('',#14230,#14232,#7463,.T.) ;
#17900=EDGE_CURVE('',#14229,#14231,#7464,.T.) ;
#17901=EDGE_CURVE('',#14233,#14234,#11624,.T.) ;
#17902=EDGE_CURVE('',#14234,#14232,#11625,.T.) ;
#17903=EDGE_CURVE('',#14233,#14231,#11626,.T.) ;
#17904=EDGE_CURVE('',#14235,#14236,#11627,.T.) ;
#17905=EDGE_CURVE('',#14234,#14236,#7465,.T.) ;
#17906=EDGE_CURVE('',#14233,#14235,#7466,.T.) ;
#17907=EDGE_CURVE('',#14237,#14238,#11628,.T.) ;
#17908=EDGE_CURVE('',#14238,#14236,#11629,.T.) ;
#17909=EDGE_CURVE('',#14235,#14237,#11630,.T.) ;
#17910=EDGE_CURVE('',#14239,#14240,#11631,.T.) ;
#17911=EDGE_CURVE('',#14238,#14240,#7467,.T.) ;
#17912=EDGE_CURVE('',#14237,#14239,#7468,.T.) ;
#17913=EDGE_CURVE('',#14225,#14240,#11632,.T.) ;
#17914=EDGE_CURVE('',#14226,#14239,#11633,.T.) ;
#17915=EDGE_CURVE('',#14241,#14231,#7469,.T.) ;
#17916=EDGE_CURVE('',#14242,#14241,#11634,.F.) ;
#17917=EDGE_CURVE('',#14233,#14242,#7470,.T.) ;
#17918=EDGE_CURVE('',#14229,#14243,#7471,.T.) ;
#17919=EDGE_CURVE('',#14243,#14241,#7472,.T.) ;
#17920=EDGE_CURVE('',#14244,#14227,#7473,.T.) ;
#17921=EDGE_CURVE('',#14243,#14244,#11635,.F.) ;
#17922=EDGE_CURVE('',#14226,#14245,#7474,.T.) ;
#17923=EDGE_CURVE('',#14245,#14244,#7475,.T.) ;
#17924=EDGE_CURVE('',#14246,#14247,#11636,.T.) ;
#17925=EDGE_CURVE('',#14247,#14248,#7476,.T.) ;
#17926=EDGE_CURVE('',#14248,#14249,#11637,.T.) ;
#17927=EDGE_CURVE('',#14246,#14249,#7477,.T.) ;
#17928=EDGE_CURVE('',#14250,#14251,#11638,.T.) ;
#17929=EDGE_CURVE('',#14251,#14249,#11639,.T.) ;
#17930=EDGE_CURVE('',#14248,#14250,#11640,.T.) ;
#17931=EDGE_CURVE('',#14252,#14253,#11641,.T.) ;
#17932=EDGE_CURVE('',#14251,#14253,#7478,.T.) ;
#17933=EDGE_CURVE('',#14250,#14252,#7479,.T.) ;
#17934=EDGE_CURVE('',#14254,#14255,#11642,.T.) ;
#17935=EDGE_CURVE('',#14255,#14253,#11643,.T.) ;
#17936=EDGE_CURVE('',#14254,#14252,#11644,.T.) ;
#17937=EDGE_CURVE('',#14256,#14257,#11645,.T.) ;
#17938=EDGE_CURVE('',#14255,#14257,#7480,.T.) ;
#17939=EDGE_CURVE('',#14254,#14256,#7481,.T.) ;
#17940=EDGE_CURVE('',#14258,#14259,#11646,.T.) ;
#17941=EDGE_CURVE('',#14259,#14257,#11647,.T.) ;
#17942=EDGE_CURVE('',#14256,#14258,#11648,.T.) ;
#17943=EDGE_CURVE('',#14260,#14261,#11649,.T.) ;
#17944=EDGE_CURVE('',#14259,#14261,#7482,.T.) ;
#17945=EDGE_CURVE('',#14258,#14260,#7483,.T.) ;
#17946=EDGE_CURVE('',#14246,#14261,#11650,.T.) ;
#17947=EDGE_CURVE('',#14247,#14260,#11651,.T.) ;
#17948=EDGE_CURVE('',#14262,#14252,#7484,.T.) ;
#17949=EDGE_CURVE('',#14263,#14262,#11652,.F.) ;
#17950=EDGE_CURVE('',#14254,#14263,#7485,.T.) ;
#17951=EDGE_CURVE('',#14250,#14264,#7486,.T.) ;
#17952=EDGE_CURVE('',#14264,#14262,#7487,.T.) ;
#17953=EDGE_CURVE('',#14265,#14248,#7488,.T.) ;
#17954=EDGE_CURVE('',#14264,#14265,#11653,.F.) ;
#17955=EDGE_CURVE('',#14247,#14266,#7489,.T.) ;
#17956=EDGE_CURVE('',#14266,#14265,#7490,.T.) ;
#17957=EDGE_CURVE('',#14267,#14268,#11654,.T.) ;
#17958=EDGE_CURVE('',#14268,#14269,#7491,.T.) ;
#17959=EDGE_CURVE('',#14269,#14270,#11655,.T.) ;
#17960=EDGE_CURVE('',#14267,#14270,#7492,.T.) ;
#17961=EDGE_CURVE('',#14271,#14272,#11656,.T.) ;
#17962=EDGE_CURVE('',#14272,#14270,#11657,.T.) ;
#17963=EDGE_CURVE('',#14269,#14271,#11658,.T.) ;
#17964=EDGE_CURVE('',#14273,#14274,#11659,.T.) ;
#17965=EDGE_CURVE('',#14272,#14274,#7493,.T.) ;
#17966=EDGE_CURVE('',#14271,#14273,#7494,.T.) ;
#17967=EDGE_CURVE('',#14275,#14276,#11660,.T.) ;
#17968=EDGE_CURVE('',#14276,#14274,#11661,.T.) ;
#17969=EDGE_CURVE('',#14275,#14273,#11662,.T.) ;
#17970=EDGE_CURVE('',#14277,#14278,#11663,.T.) ;
#17971=EDGE_CURVE('',#14276,#14278,#7495,.T.) ;
#17972=EDGE_CURVE('',#14275,#14277,#7496,.T.) ;
#17973=EDGE_CURVE('',#14279,#14280,#11664,.T.) ;
#17974=EDGE_CURVE('',#14280,#14278,#11665,.T.) ;
#17975=EDGE_CURVE('',#14277,#14279,#11666,.T.) ;
#17976=EDGE_CURVE('',#14281,#14282,#11667,.T.) ;
#17977=EDGE_CURVE('',#14280,#14282,#7497,.T.) ;
#17978=EDGE_CURVE('',#14279,#14281,#7498,.T.) ;
#17979=EDGE_CURVE('',#14267,#14282,#11668,.T.) ;
#17980=EDGE_CURVE('',#14268,#14281,#11669,.T.) ;
#17981=EDGE_CURVE('',#14283,#14273,#7499,.T.) ;
#17982=EDGE_CURVE('',#14284,#14283,#11670,.F.) ;
#17983=EDGE_CURVE('',#14275,#14284,#7500,.T.) ;
#17984=EDGE_CURVE('',#14271,#14285,#7501,.T.) ;
#17985=EDGE_CURVE('',#14285,#14283,#7502,.T.) ;
#17986=EDGE_CURVE('',#14286,#14269,#7503,.T.) ;
#17987=EDGE_CURVE('',#14285,#14286,#11671,.F.) ;
#17988=EDGE_CURVE('',#14268,#14287,#7504,.T.) ;
#17989=EDGE_CURVE('',#14287,#14286,#7505,.T.) ;
#17990=EDGE_CURVE('',#14288,#14289,#11672,.T.) ;
#17991=EDGE_CURVE('',#14289,#14290,#7506,.T.) ;
#17992=EDGE_CURVE('',#14290,#14291,#11673,.T.) ;
#17993=EDGE_CURVE('',#14288,#14291,#7507,.T.) ;
#17994=EDGE_CURVE('',#14292,#14293,#11674,.T.) ;
#17995=EDGE_CURVE('',#14293,#14291,#11675,.T.) ;
#17996=EDGE_CURVE('',#14290,#14292,#11676,.T.) ;
#17997=EDGE_CURVE('',#14294,#14295,#11677,.T.) ;
#17998=EDGE_CURVE('',#14293,#14295,#7508,.T.) ;
#17999=EDGE_CURVE('',#14292,#14294,#7509,.T.) ;
#18000=EDGE_CURVE('',#14296,#14297,#11678,.T.) ;
#18001=EDGE_CURVE('',#14297,#14295,#11679,.T.) ;
#18002=EDGE_CURVE('',#14296,#14294,#11680,.T.) ;
#18003=EDGE_CURVE('',#14298,#14299,#11681,.T.) ;
#18004=EDGE_CURVE('',#14297,#14299,#7510,.T.) ;
#18005=EDGE_CURVE('',#14296,#14298,#7511,.T.) ;
#18006=EDGE_CURVE('',#13963,#14300,#11682,.T.) ;
#18007=EDGE_CURVE('',#14300,#14299,#11683,.T.) ;
#18008=EDGE_CURVE('',#14298,#13963,#11684,.T.) ;
#18009=EDGE_CURVE('',#13962,#14301,#11685,.T.) ;
#18010=EDGE_CURVE('',#14300,#14301,#7512,.T.) ;
#18011=EDGE_CURVE('',#14288,#14301,#11686,.T.) ;
#18012=EDGE_CURVE('',#14289,#13962,#11687,.T.) ;
#18013=EDGE_CURVE('',#14302,#14294,#7513,.T.) ;
#18014=EDGE_CURVE('',#14302,#14303,#11688,.T.) ;
#18015=EDGE_CURVE('',#14303,#14296,#7514,.T.) ;
#18016=EDGE_CURVE('',#13955,#14304,#7515,.T.) ;
#18017=EDGE_CURVE('',#14304,#14305,#11689,.T.) ;
#18018=EDGE_CURVE('',#14305,#14302,#7516,.T.) ;
#18019=EDGE_CURVE('',#14292,#14306,#7517,.T.) ;
#18020=EDGE_CURVE('',#14306,#14307,#7518,.T.) ;
#18021=EDGE_CURVE('',#14307,#14308,#11690,.T.) ;
#18022=EDGE_CURVE('',#14308,#13956,#7519,.T.) ;
#18023=EDGE_CURVE('',#14309,#14290,#7520,.T.) ;
#18024=EDGE_CURVE('',#14309,#14306,#11691,.T.) ;
#18025=EDGE_CURVE('',#14289,#14310,#7521,.T.) ;
#18026=EDGE_CURVE('',#14310,#14309,#7522,.T.) ;
#18027=EDGE_CURVE('',#14311,#14312,#11692,.T.) ;
#18028=EDGE_CURVE('',#14312,#14313,#7523,.T.) ;
#18029=EDGE_CURVE('',#14313,#14314,#11693,.T.) ;
#18030=EDGE_CURVE('',#14311,#14314,#7524,.T.) ;
#18031=EDGE_CURVE('',#14315,#14316,#11694,.T.) ;
#18032=EDGE_CURVE('',#14316,#14314,#11695,.T.) ;
#18033=EDGE_CURVE('',#14313,#14315,#11696,.T.) ;
#18034=EDGE_CURVE('',#14317,#14318,#11697,.T.) ;
#18035=EDGE_CURVE('',#14316,#14318,#7525,.T.) ;
#18036=EDGE_CURVE('',#14315,#14317,#7526,.T.) ;
#18037=EDGE_CURVE('',#14319,#14320,#11698,.T.) ;
#18038=EDGE_CURVE('',#14320,#14318,#11699,.T.) ;
#18039=EDGE_CURVE('',#14319,#14317,#11700,.T.) ;
#18040=EDGE_CURVE('',#14321,#14322,#11701,.T.) ;
#18041=EDGE_CURVE('',#14320,#14322,#7527,.T.) ;
#18042=EDGE_CURVE('',#14319,#14321,#7528,.T.) ;
#18043=EDGE_CURVE('',#13982,#14323,#11702,.T.) ;
#18044=EDGE_CURVE('',#14323,#14322,#11703,.T.) ;
#18045=EDGE_CURVE('',#14321,#13982,#11704,.T.) ;
#18046=EDGE_CURVE('',#13981,#14324,#11705,.T.) ;
#18047=EDGE_CURVE('',#14323,#14324,#7529,.T.) ;
#18048=EDGE_CURVE('',#14311,#14324,#11706,.T.) ;
#18049=EDGE_CURVE('',#14312,#13981,#11707,.T.) ;
#18050=EDGE_CURVE('',#14325,#14317,#7530,.T.) ;
#18051=EDGE_CURVE('',#14325,#14326,#11708,.T.) ;
#18052=EDGE_CURVE('',#14326,#14319,#7531,.T.) ;
#18053=EDGE_CURVE('',#13974,#14327,#7532,.T.) ;
#18054=EDGE_CURVE('',#14327,#14328,#11709,.T.) ;
#18055=EDGE_CURVE('',#14328,#14325,#7533,.T.) ;
#18056=EDGE_CURVE('',#14315,#14329,#7534,.T.) ;
#18057=EDGE_CURVE('',#14329,#14330,#7535,.T.) ;
#18058=EDGE_CURVE('',#14330,#14331,#11710,.T.) ;
#18059=EDGE_CURVE('',#14331,#13975,#7536,.T.) ;
#18060=EDGE_CURVE('',#14332,#14313,#7537,.T.) ;
#18061=EDGE_CURVE('',#14332,#14329,#11711,.T.) ;
#18062=EDGE_CURVE('',#14312,#14333,#7538,.T.) ;
#18063=EDGE_CURVE('',#14333,#14332,#7539,.T.) ;
#18064=EDGE_CURVE('',#14334,#14335,#11712,.T.) ;
#18065=EDGE_CURVE('',#14335,#14336,#7540,.T.) ;
#18066=EDGE_CURVE('',#14336,#14337,#11713,.T.) ;
#18067=EDGE_CURVE('',#14334,#14337,#7541,.T.) ;
#18068=EDGE_CURVE('',#14338,#14339,#11714,.T.) ;
#18069=EDGE_CURVE('',#14339,#14337,#11715,.T.) ;
#18070=EDGE_CURVE('',#14336,#14338,#11716,.T.) ;
#18071=EDGE_CURVE('',#14340,#14341,#11717,.T.) ;
#18072=EDGE_CURVE('',#14339,#14341,#7542,.T.) ;
#18073=EDGE_CURVE('',#14338,#14340,#7543,.T.) ;
#18074=EDGE_CURVE('',#14342,#14343,#11718,.T.) ;
#18075=EDGE_CURVE('',#14343,#14341,#11719,.T.) ;
#18076=EDGE_CURVE('',#14342,#14340,#11720,.T.) ;
#18077=EDGE_CURVE('',#14344,#14345,#11721,.T.) ;
#18078=EDGE_CURVE('',#14343,#14345,#7544,.T.) ;
#18079=EDGE_CURVE('',#14342,#14344,#7545,.T.) ;
#18080=EDGE_CURVE('',#14001,#14346,#11722,.T.) ;
#18081=EDGE_CURVE('',#14346,#14345,#11723,.T.) ;
#18082=EDGE_CURVE('',#14344,#14001,#11724,.T.) ;
#18083=EDGE_CURVE('',#14000,#14347,#11725,.T.) ;
#18084=EDGE_CURVE('',#14346,#14347,#7546,.T.) ;
#18085=EDGE_CURVE('',#14334,#14347,#11726,.T.) ;
#18086=EDGE_CURVE('',#14335,#14000,#11727,.T.) ;
#18087=EDGE_CURVE('',#14348,#14340,#7547,.T.) ;
#18088=EDGE_CURVE('',#14348,#14349,#11728,.T.) ;
#18089=EDGE_CURVE('',#14349,#14342,#7548,.T.) ;
#18090=EDGE_CURVE('',#13993,#14350,#7549,.T.) ;
#18091=EDGE_CURVE('',#14350,#14351,#11729,.T.) ;
#18092=EDGE_CURVE('',#14351,#14348,#7550,.T.) ;
#18093=EDGE_CURVE('',#14338,#14352,#7551,.T.) ;
#18094=EDGE_CURVE('',#14352,#14353,#7552,.T.) ;
#18095=EDGE_CURVE('',#14353,#14354,#11730,.T.) ;
#18096=EDGE_CURVE('',#14354,#13994,#7553,.T.) ;
#18097=EDGE_CURVE('',#14355,#14336,#7554,.T.) ;
#18098=EDGE_CURVE('',#14355,#14352,#11731,.T.) ;
#18099=EDGE_CURVE('',#14335,#14356,#7555,.T.) ;
#18100=EDGE_CURVE('',#14356,#14355,#7556,.T.) ;
#18101=EDGE_CURVE('',#14357,#14358,#11732,.T.) ;
#18102=EDGE_CURVE('',#14358,#14359,#7557,.T.) ;
#18103=EDGE_CURVE('',#14359,#14360,#11733,.T.) ;
#18104=EDGE_CURVE('',#14357,#14360,#7558,.T.) ;
#18105=EDGE_CURVE('',#14361,#14362,#11734,.T.) ;
#18106=EDGE_CURVE('',#14362,#14360,#11735,.T.) ;
#18107=EDGE_CURVE('',#14359,#14361,#11736,.T.) ;
#18108=EDGE_CURVE('',#14363,#14364,#11737,.T.) ;
#18109=EDGE_CURVE('',#14362,#14364,#7559,.T.) ;
#18110=EDGE_CURVE('',#14361,#14363,#7560,.T.) ;
#18111=EDGE_CURVE('',#14365,#14366,#11738,.T.) ;
#18112=EDGE_CURVE('',#14366,#14364,#11739,.T.) ;
#18113=EDGE_CURVE('',#14365,#14363,#11740,.T.) ;
#18114=EDGE_CURVE('',#14367,#14368,#11741,.T.) ;
#18115=EDGE_CURVE('',#14366,#14368,#7561,.T.) ;
#18116=EDGE_CURVE('',#14365,#14367,#7562,.T.) ;
#18117=EDGE_CURVE('',#14020,#14369,#11742,.T.) ;
#18118=EDGE_CURVE('',#14369,#14368,#11743,.T.) ;
#18119=EDGE_CURVE('',#14367,#14020,#11744,.T.) ;
#18120=EDGE_CURVE('',#14019,#14370,#11745,.T.) ;
#18121=EDGE_CURVE('',#14369,#14370,#7563,.T.) ;
#18122=EDGE_CURVE('',#14357,#14370,#11746,.T.) ;
#18123=EDGE_CURVE('',#14358,#14019,#11747,.T.) ;
#18124=EDGE_CURVE('',#14371,#14363,#7564,.T.) ;
#18125=EDGE_CURVE('',#14371,#14372,#11748,.T.) ;
#18126=EDGE_CURVE('',#14372,#14365,#7565,.T.) ;
#18127=EDGE_CURVE('',#14012,#14373,#7566,.T.) ;
#18128=EDGE_CURVE('',#14373,#14374,#11749,.T.) ;
#18129=EDGE_CURVE('',#14374,#14371,#7567,.T.) ;
#18130=EDGE_CURVE('',#14361,#14375,#7568,.T.) ;
#18131=EDGE_CURVE('',#14375,#14376,#7569,.T.) ;
#18132=EDGE_CURVE('',#14376,#14377,#11750,.T.) ;
#18133=EDGE_CURVE('',#14377,#14013,#7570,.T.) ;
#18134=EDGE_CURVE('',#14378,#14359,#7571,.T.) ;
#18135=EDGE_CURVE('',#14378,#14375,#11751,.T.) ;
#18136=EDGE_CURVE('',#14358,#14379,#7572,.T.) ;
#18137=EDGE_CURVE('',#14379,#14378,#7573,.T.) ;
#18138=EDGE_CURVE('',#14380,#14381,#11752,.T.) ;
#18139=EDGE_CURVE('',#14381,#14382,#7574,.T.) ;
#18140=EDGE_CURVE('',#14382,#14383,#11753,.T.) ;
#18141=EDGE_CURVE('',#14380,#14383,#7575,.T.) ;
#18142=EDGE_CURVE('',#14384,#14385,#11754,.T.) ;
#18143=EDGE_CURVE('',#14385,#14383,#11755,.T.) ;
#18144=EDGE_CURVE('',#14382,#14384,#11756,.T.) ;
#18145=EDGE_CURVE('',#14386,#14387,#11757,.T.) ;
#18146=EDGE_CURVE('',#14385,#14387,#7576,.T.) ;
#18147=EDGE_CURVE('',#14384,#14386,#7577,.T.) ;
#18148=EDGE_CURVE('',#14388,#14389,#11758,.T.) ;
#18149=EDGE_CURVE('',#14389,#14387,#11759,.T.) ;
#18150=EDGE_CURVE('',#14388,#14386,#11760,.T.) ;
#18151=EDGE_CURVE('',#14390,#14391,#11761,.T.) ;
#18152=EDGE_CURVE('',#14389,#14391,#7578,.T.) ;
#18153=EDGE_CURVE('',#14388,#14390,#7579,.T.) ;
#18154=EDGE_CURVE('',#14039,#14392,#11762,.T.) ;
#18155=EDGE_CURVE('',#14392,#14391,#11763,.T.) ;
#18156=EDGE_CURVE('',#14390,#14039,#11764,.T.) ;
#18157=EDGE_CURVE('',#14038,#14393,#11765,.T.) ;
#18158=EDGE_CURVE('',#14392,#14393,#7580,.T.) ;
#18159=EDGE_CURVE('',#14380,#14393,#11766,.T.) ;
#18160=EDGE_CURVE('',#14381,#14038,#11767,.T.) ;
#18161=EDGE_CURVE('',#14394,#14386,#7581,.T.) ;
#18162=EDGE_CURVE('',#14394,#14395,#11768,.T.) ;
#18163=EDGE_CURVE('',#14395,#14388,#7582,.T.) ;
#18164=EDGE_CURVE('',#14031,#14396,#7583,.T.) ;
#18165=EDGE_CURVE('',#14396,#14397,#11769,.T.) ;
#18166=EDGE_CURVE('',#14397,#14394,#7584,.T.) ;
#18167=EDGE_CURVE('',#14384,#14398,#7585,.T.) ;
#18168=EDGE_CURVE('',#14398,#14399,#7586,.T.) ;
#18169=EDGE_CURVE('',#14399,#14400,#11770,.T.) ;
#18170=EDGE_CURVE('',#14400,#14032,#7587,.T.) ;
#18171=EDGE_CURVE('',#14401,#14382,#7588,.T.) ;
#18172=EDGE_CURVE('',#14401,#14398,#11771,.T.) ;
#18173=EDGE_CURVE('',#14381,#14402,#7589,.T.) ;
#18174=EDGE_CURVE('',#14402,#14401,#7590,.T.) ;
#18175=EDGE_CURVE('',#14403,#14404,#11772,.T.) ;
#18176=EDGE_CURVE('',#14404,#14405,#7591,.T.) ;
#18177=EDGE_CURVE('',#14405,#14406,#11773,.T.) ;
#18178=EDGE_CURVE('',#14403,#14406,#7592,.T.) ;
#18179=EDGE_CURVE('',#14407,#14408,#11774,.T.) ;
#18180=EDGE_CURVE('',#14408,#14406,#11775,.T.) ;
#18181=EDGE_CURVE('',#14405,#14407,#11776,.T.) ;
#18182=EDGE_CURVE('',#14409,#14410,#11777,.T.) ;
#18183=EDGE_CURVE('',#14408,#14410,#7593,.T.) ;
#18184=EDGE_CURVE('',#14407,#14409,#7594,.T.) ;
#18185=EDGE_CURVE('',#14411,#14412,#11778,.T.) ;
#18186=EDGE_CURVE('',#14412,#14410,#11779,.T.) ;
#18187=EDGE_CURVE('',#14411,#14409,#11780,.T.) ;
#18188=EDGE_CURVE('',#14413,#14414,#11781,.T.) ;
#18189=EDGE_CURVE('',#14412,#14414,#7595,.T.) ;
#18190=EDGE_CURVE('',#14411,#14413,#7596,.T.) ;
#18191=EDGE_CURVE('',#14058,#14415,#11782,.T.) ;
#18192=EDGE_CURVE('',#14415,#14414,#11783,.T.) ;
#18193=EDGE_CURVE('',#14413,#14058,#11784,.T.) ;
#18194=EDGE_CURVE('',#14057,#14416,#11785,.T.) ;
#18195=EDGE_CURVE('',#14415,#14416,#7597,.T.) ;
#18196=EDGE_CURVE('',#14403,#14416,#11786,.T.) ;
#18197=EDGE_CURVE('',#14404,#14057,#11787,.T.) ;
#18198=EDGE_CURVE('',#14417,#14409,#7598,.T.) ;
#18199=EDGE_CURVE('',#14417,#14418,#11788,.T.) ;
#18200=EDGE_CURVE('',#14418,#14411,#7599,.T.) ;
#18201=EDGE_CURVE('',#14050,#14419,#7600,.T.) ;
#18202=EDGE_CURVE('',#14419,#14420,#11789,.T.) ;
#18203=EDGE_CURVE('',#14420,#14417,#7601,.T.) ;
#18204=EDGE_CURVE('',#14407,#14421,#7602,.T.) ;
#18205=EDGE_CURVE('',#14421,#14422,#7603,.T.) ;
#18206=EDGE_CURVE('',#14422,#14423,#11790,.T.) ;
#18207=EDGE_CURVE('',#14423,#14051,#7604,.T.) ;
#18208=EDGE_CURVE('',#14424,#14405,#7605,.T.) ;
#18209=EDGE_CURVE('',#14424,#14421,#11791,.T.) ;
#18210=EDGE_CURVE('',#14404,#14425,#7606,.T.) ;
#18211=EDGE_CURVE('',#14425,#14424,#7607,.T.) ;
#18212=EDGE_CURVE('',#14426,#14427,#11792,.T.) ;
#18213=EDGE_CURVE('',#14427,#14428,#7608,.T.) ;
#18214=EDGE_CURVE('',#14428,#14429,#11793,.T.) ;
#18215=EDGE_CURVE('',#14426,#14429,#7609,.T.) ;
#18216=EDGE_CURVE('',#14430,#14431,#11794,.T.) ;
#18217=EDGE_CURVE('',#14431,#14429,#11795,.T.) ;
#18218=EDGE_CURVE('',#14428,#14430,#11796,.T.) ;
#18219=EDGE_CURVE('',#14432,#14433,#11797,.T.) ;
#18220=EDGE_CURVE('',#14431,#14433,#7610,.T.) ;
#18221=EDGE_CURVE('',#14430,#14432,#7611,.T.) ;
#18222=EDGE_CURVE('',#14434,#14435,#11798,.T.) ;
#18223=EDGE_CURVE('',#14435,#14433,#11799,.T.) ;
#18224=EDGE_CURVE('',#14434,#14432,#11800,.T.) ;
#18225=EDGE_CURVE('',#14436,#14437,#11801,.T.) ;
#18226=EDGE_CURVE('',#14435,#14437,#7612,.T.) ;
#18227=EDGE_CURVE('',#14434,#14436,#7613,.T.) ;
#18228=EDGE_CURVE('',#14077,#14438,#11802,.T.) ;
#18229=EDGE_CURVE('',#14438,#14437,#11803,.T.) ;
#18230=EDGE_CURVE('',#14436,#14077,#11804,.T.) ;
#18231=EDGE_CURVE('',#14076,#14439,#11805,.T.) ;
#18232=EDGE_CURVE('',#14438,#14439,#7614,.T.) ;
#18233=EDGE_CURVE('',#14426,#14439,#11806,.T.) ;
#18234=EDGE_CURVE('',#14427,#14076,#11807,.T.) ;
#18235=EDGE_CURVE('',#14440,#14432,#7615,.T.) ;
#18236=EDGE_CURVE('',#14440,#14441,#11808,.T.) ;
#18237=EDGE_CURVE('',#14441,#14434,#7616,.T.) ;
#18238=EDGE_CURVE('',#14069,#14442,#7617,.T.) ;
#18239=EDGE_CURVE('',#14442,#14443,#11809,.T.) ;
#18240=EDGE_CURVE('',#14443,#14440,#7618,.T.) ;
#18241=EDGE_CURVE('',#14430,#14444,#7619,.T.) ;
#18242=EDGE_CURVE('',#14444,#14445,#7620,.T.) ;
#18243=EDGE_CURVE('',#14445,#14446,#11810,.T.) ;
#18244=EDGE_CURVE('',#14446,#14070,#7621,.T.) ;
#18245=EDGE_CURVE('',#14447,#14428,#7622,.T.) ;
#18246=EDGE_CURVE('',#14447,#14444,#11811,.T.) ;
#18247=EDGE_CURVE('',#14427,#14448,#7623,.T.) ;
#18248=EDGE_CURVE('',#14448,#14447,#7624,.T.) ;
#18249=EDGE_CURVE('',#14449,#14450,#11812,.T.) ;
#18250=EDGE_CURVE('',#14450,#14451,#7625,.T.) ;
#18251=EDGE_CURVE('',#14451,#14452,#11813,.T.) ;
#18252=EDGE_CURVE('',#14449,#14452,#7626,.T.) ;
#18253=EDGE_CURVE('',#14453,#14454,#11814,.T.) ;
#18254=EDGE_CURVE('',#14454,#14452,#11815,.T.) ;
#18255=EDGE_CURVE('',#14451,#14453,#11816,.T.) ;
#18256=EDGE_CURVE('',#14455,#14456,#11817,.T.) ;
#18257=EDGE_CURVE('',#14454,#14456,#7627,.T.) ;
#18258=EDGE_CURVE('',#14453,#14455,#7628,.T.) ;
#18259=EDGE_CURVE('',#14457,#14458,#11818,.T.) ;
#18260=EDGE_CURVE('',#14458,#14456,#11819,.T.) ;
#18261=EDGE_CURVE('',#14457,#14455,#11820,.T.) ;
#18262=EDGE_CURVE('',#14459,#14460,#11821,.T.) ;
#18263=EDGE_CURVE('',#14458,#14460,#7629,.T.) ;
#18264=EDGE_CURVE('',#14457,#14459,#7630,.T.) ;
#18265=EDGE_CURVE('',#14096,#14461,#11822,.T.) ;
#18266=EDGE_CURVE('',#14461,#14460,#11823,.T.) ;
#18267=EDGE_CURVE('',#14459,#14096,#11824,.T.) ;
#18268=EDGE_CURVE('',#14095,#14462,#11825,.T.) ;
#18269=EDGE_CURVE('',#14461,#14462,#7631,.T.) ;
#18270=EDGE_CURVE('',#14449,#14462,#11826,.T.) ;
#18271=EDGE_CURVE('',#14450,#14095,#11827,.T.) ;
#18272=EDGE_CURVE('',#14463,#14455,#7632,.T.) ;
#18273=EDGE_CURVE('',#14463,#14464,#11828,.T.) ;
#18274=EDGE_CURVE('',#14464,#14457,#7633,.T.) ;
#18275=EDGE_CURVE('',#14088,#14465,#7634,.T.) ;
#18276=EDGE_CURVE('',#14465,#14466,#11829,.T.) ;
#18277=EDGE_CURVE('',#14466,#14463,#7635,.T.) ;
#18278=EDGE_CURVE('',#14453,#14467,#7636,.T.) ;
#18279=EDGE_CURVE('',#14467,#14468,#7637,.T.) ;
#18280=EDGE_CURVE('',#14468,#14469,#11830,.T.) ;
#18281=EDGE_CURVE('',#14469,#14089,#7638,.T.) ;
#18282=EDGE_CURVE('',#14470,#14451,#7639,.T.) ;
#18283=EDGE_CURVE('',#14470,#14467,#11831,.T.) ;
#18284=EDGE_CURVE('',#14450,#14471,#7640,.T.) ;
#18285=EDGE_CURVE('',#14471,#14470,#7641,.T.) ;
#18286=EDGE_CURVE('',#14472,#14473,#11832,.T.) ;
#18287=EDGE_CURVE('',#14473,#14474,#7642,.T.) ;
#18288=EDGE_CURVE('',#14474,#14475,#11833,.T.) ;
#18289=EDGE_CURVE('',#14475,#14472,#7643,.T.) ;
#18290=EDGE_CURVE('',#14476,#14477,#11834,.T.) ;
#18291=EDGE_CURVE('',#14477,#14475,#11835,.T.) ;
#18292=EDGE_CURVE('',#14474,#14476,#11836,.T.) ;
#18293=EDGE_CURVE('',#14478,#14479,#11837,.T.) ;
#18294=EDGE_CURVE('',#14479,#14477,#7644,.T.) ;
#18295=EDGE_CURVE('',#14476,#14478,#7645,.T.) ;
#18296=EDGE_CURVE('',#14480,#14481,#11838,.T.) ;
#18297=EDGE_CURVE('',#14481,#14479,#11839,.T.) ;
#18298=EDGE_CURVE('',#14478,#14480,#11840,.T.) ;
#18299=EDGE_CURVE('',#14482,#14483,#11841,.T.) ;
#18300=EDGE_CURVE('',#14483,#14481,#7646,.T.) ;
#18301=EDGE_CURVE('',#14480,#14482,#7647,.T.) ;
#18302=EDGE_CURVE('',#14484,#14485,#11842,.T.) ;
#18303=EDGE_CURVE('',#14485,#14483,#11843,.T.) ;
#18304=EDGE_CURVE('',#14482,#14484,#11844,.T.) ;
#18305=EDGE_CURVE('',#14486,#14487,#11845,.T.) ;
#18306=EDGE_CURVE('',#14487,#14485,#7648,.T.) ;
#18307=EDGE_CURVE('',#14484,#14486,#7649,.T.) ;
#18308=EDGE_CURVE('',#14472,#14487,#11846,.T.) ;
#18309=EDGE_CURVE('',#14486,#14473,#11847,.T.) ;
#18310=EDGE_CURVE('',#14488,#14478,#7650,.T.) ;
#18311=EDGE_CURVE('',#14489,#14488,#11848,.F.) ;
#18312=EDGE_CURVE('',#14480,#14489,#7651,.T.) ;
#18313=EDGE_CURVE('',#14476,#14490,#7652,.T.) ;
#18314=EDGE_CURVE('',#14490,#14488,#7653,.T.) ;
#18315=EDGE_CURVE('',#14491,#14474,#7654,.T.) ;
#18316=EDGE_CURVE('',#14490,#14491,#11849,.F.) ;
#18317=EDGE_CURVE('',#14473,#14492,#7655,.T.) ;
#18318=EDGE_CURVE('',#14492,#14491,#7656,.T.) ;
#18319=EDGE_CURVE('',#14493,#14494,#7657,.T.) ;
#18320=EDGE_CURVE('',#14495,#14494,#7658,.T.) ;
#18321=EDGE_CURVE('',#14495,#14496,#7659,.T.) ;
#18322=EDGE_CURVE('',#14493,#14496,#7660,.T.) ;
#18323=EDGE_CURVE('',#14497,#14498,#7661,.T.) ;
#18324=EDGE_CURVE('',#14499,#14497,#11850,.T.) ;
#18325=EDGE_CURVE('',#14500,#14499,#7662,.T.) ;
#18326=EDGE_CURVE('',#14501,#14500,#11851,.T.) ;
#18327=EDGE_CURVE('',#14502,#14501,#7663,.T.) ;
#18328=EDGE_CURVE('',#14503,#14502,#11852,.T.) ;
#18329=EDGE_CURVE('',#14504,#14503,#7664,.T.) ;
#18330=EDGE_CURVE('',#14498,#14504,#11853,.T.) ;
#18331=EDGE_CURVE('',#14505,#14505,#11854,.T.) ;
#18332=EDGE_CURVE('',#14498,#14506,#11855,.T.) ;
#18333=EDGE_CURVE('',#14506,#14507,#7665,.T.) ;
#18334=EDGE_CURVE('',#14507,#14497,#11856,.T.) ;
#18335=EDGE_CURVE('',#14508,#14499,#11857,.T.) ;
#18336=EDGE_CURVE('',#14507,#14508,#11858,.T.) ;
#18337=EDGE_CURVE('',#14509,#14500,#11859,.T.) ;
#18338=EDGE_CURVE('',#14508,#14509,#7666,.T.) ;
#18339=EDGE_CURVE('',#14510,#14501,#11860,.T.) ;
#18340=EDGE_CURVE('',#14509,#14510,#11861,.T.) ;
#18341=EDGE_CURVE('',#14511,#14502,#11862,.T.) ;
#18342=EDGE_CURVE('',#14510,#14511,#7667,.T.) ;
#18343=EDGE_CURVE('',#14111,#14503,#11863,.T.) ;
#18344=EDGE_CURVE('',#14511,#14111,#11864,.T.) ;
#18345=EDGE_CURVE('',#14112,#14504,#11865,.T.) ;
#18346=EDGE_CURVE('',#14112,#14506,#11866,.T.) ;
#18347=EDGE_CURVE('',#14512,#14509,#7668,.T.) ;
#18348=EDGE_CURVE('',#14512,#14513,#11867,.T.) ;
#18349=EDGE_CURVE('',#14513,#14510,#7669,.T.) ;
#18350=EDGE_CURVE('',#14508,#14514,#7670,.T.) ;
#18351=EDGE_CURVE('',#14514,#14515,#7671,.T.) ;
#18352=EDGE_CURVE('',#14515,#14516,#11868,.T.) ;
#18353=EDGE_CURVE('',#14516,#14108,#7672,.T.) ;
#18354=EDGE_CURVE('',#14107,#14517,#7673,.T.) ;
#18355=EDGE_CURVE('',#14517,#14518,#11869,.T.) ;
#18356=EDGE_CURVE('',#14518,#14512,#7674,.T.) ;
#18357=EDGE_CURVE('',#14507,#14519,#7675,.T.) ;
#18358=EDGE_CURVE('',#14519,#14514,#11870,.T.) ;
#18359=EDGE_CURVE('',#14506,#14520,#7676,.T.) ;
#18360=EDGE_CURVE('',#14520,#14519,#7677,.T.) ;
#18361=EDGE_CURVE('',#14513,#14521,#7678,.T.) ;
#18362=EDGE_CURVE('',#14521,#14511,#7679,.T.) ;
#18363=EDGE_CURVE('',#14521,#14113,#11871,.T.) ;
#18364=EDGE_CURVE('',#14117,#14520,#11872,.T.) ;
#18365=EDGE_CURVE('',#14489,#14522,#7680,.T.) ;
#18366=EDGE_CURVE('',#14522,#14482,#7681,.T.) ;
#18367=EDGE_CURVE('',#14522,#14523,#11873,.T.) ;
#18368=EDGE_CURVE('',#14484,#14523,#7682,.T.) ;
#18369=EDGE_CURVE('',#14524,#14486,#7683,.T.) ;
#18370=EDGE_CURVE('',#14524,#14492,#11874,.T.) ;
#18371=EDGE_CURVE('',#14523,#14524,#7684,.T.) ;
#18372=EDGE_CURVE('',#14525,#14525,#11875,.T.) ;
#18373=EDGE_CURVE('',#14119,#14516,#11876,.T.) ;
#18374=EDGE_CURVE('',#14521,#14526,#11877,.T.) ;
#18375=EDGE_CURVE('',#14527,#14513,#11878,.T.) ;
#18376=EDGE_CURVE('',#14526,#14527,#7685,.T.) ;
#18377=EDGE_CURVE('',#14528,#14119,#11879,.F.) ;
#18378=EDGE_CURVE('',#14515,#14528,#11880,.T.) ;
#18379=EDGE_CURVE('',#14529,#14514,#11881,.T.) ;
#18380=EDGE_CURVE('',#14528,#14529,#7686,.T.) ;
#18381=EDGE_CURVE('',#14118,#14530,#11882,.F.) ;
#18382=EDGE_CURVE('',#14530,#14116,#11883,.T.) ;
#18383=EDGE_CURVE('',#14531,#14532,#11884,.F.) ;
#18384=EDGE_CURVE('',#14532,#14518,#11885,.T.) ;
#18385=EDGE_CURVE('',#14517,#14531,#11886,.T.) ;
#18386=EDGE_CURVE('',#14531,#14106,#7687,.T.) ;
#18387=EDGE_CURVE('',#14512,#14527,#11887,.T.) ;
#18388=EDGE_CURVE('',#14527,#14532,#7688,.T.) ;
#18389=EDGE_CURVE('',#14533,#14110,#11888,.F.) ;
#18390=EDGE_CURVE('',#14114,#14533,#11889,.T.) ;
#18391=EDGE_CURVE('',#14526,#14113,#11890,.T.) ;
#18392=EDGE_CURVE('',#14533,#14526,#7689,.T.) ;
#18393=EDGE_CURVE('',#14532,#14533,#7690,.T.) ;
#18394=EDGE_CURVE('',#14110,#14531,#7691,.T.) ;
#18395=EDGE_CURVE('',#14117,#14534,#11891,.T.) ;
#18396=EDGE_CURVE('',#14534,#14530,#7692,.T.) ;
#18397=EDGE_CURVE('',#14530,#14528,#7693,.T.) ;
#18398=EDGE_CURVE('',#14534,#14520,#11892,.T.) ;
#18399=EDGE_CURVE('',#14529,#14534,#7694,.T.) ;
#18400=EDGE_CURVE('',#14519,#14529,#11893,.T.) ;
#18401=EDGE_CURVE('',#14535,#14536,#7695,.T.) ;
#18402=EDGE_CURVE('',#14536,#14537,#7696,.T.) ;
#18403=EDGE_CURVE('',#14537,#14538,#7697,.T.) ;
#18404=EDGE_CURVE('',#14538,#14535,#7698,.T.) ;
#18405=EDGE_CURVE('',#14522,#14536,#11894,.T.) ;
#18406=EDGE_CURVE('',#14536,#14523,#11895,.T.) ;
#18407=EDGE_CURVE('',#14524,#14535,#11896,.T.) ;
#18408=EDGE_CURVE('',#14535,#14492,#11897,.T.) ;
#18409=EDGE_CURVE('',#14491,#14538,#11898,.F.) ;
#18410=EDGE_CURVE('',#14537,#14489,#11899,.F.) ;
#18411=EDGE_CURVE('',#14488,#14537,#11900,.F.) ;
#18412=EDGE_CURVE('',#14538,#14490,#11901,.F.) ;
#18413=EDGE_CURVE('',#14100,#14469,#11902,.T.) ;
#18414=EDGE_CURVE('',#14539,#14540,#11903,.T.) ;
#18415=EDGE_CURVE('',#14464,#14539,#7699,.T.) ;
#18416=EDGE_CURVE('',#14541,#14464,#11904,.T.) ;
#18417=EDGE_CURVE('',#14540,#14541,#7700,.T.) ;
#18418=EDGE_CURVE('',#14542,#14100,#11905,.F.) ;
#18419=EDGE_CURVE('',#14468,#14542,#11906,.T.) ;
#18420=EDGE_CURVE('',#14543,#14467,#11907,.T.) ;
#18421=EDGE_CURVE('',#14542,#14543,#7701,.T.) ;
#18422=EDGE_CURVE('',#14099,#14544,#11908,.F.) ;
#18423=EDGE_CURVE('',#14544,#14093,#11909,.T.) ;
#18424=EDGE_CURVE('',#14545,#14546,#11910,.F.) ;
#18425=EDGE_CURVE('',#14546,#14466,#11911,.T.) ;
#18426=EDGE_CURVE('',#14465,#14545,#11912,.T.) ;
#18427=EDGE_CURVE('',#14545,#14087,#7702,.T.) ;
#18428=EDGE_CURVE('',#14463,#14541,#11913,.T.) ;
#18429=EDGE_CURVE('',#14541,#14546,#7703,.T.) ;
#18430=EDGE_CURVE('',#14547,#14091,#11914,.F.) ;
#18431=EDGE_CURVE('',#14098,#14547,#11915,.T.) ;
#18432=EDGE_CURVE('',#14540,#14097,#11916,.T.) ;
#18433=EDGE_CURVE('',#14547,#14540,#7704,.T.) ;
#18434=EDGE_CURVE('',#14546,#14547,#7705,.T.) ;
#18435=EDGE_CURVE('',#14091,#14545,#7706,.T.) ;
#18436=EDGE_CURVE('',#14094,#14548,#11917,.T.) ;
#18437=EDGE_CURVE('',#14548,#14544,#7707,.T.) ;
#18438=EDGE_CURVE('',#14544,#14542,#7708,.T.) ;
#18439=EDGE_CURVE('',#14539,#14097,#11918,.T.) ;
#18440=EDGE_CURVE('',#14548,#14471,#11919,.T.) ;
#18441=EDGE_CURVE('',#14543,#14548,#7709,.T.) ;
#18442=EDGE_CURVE('',#14470,#14543,#11920,.T.) ;
#18443=EDGE_CURVE('',#14094,#14471,#11921,.T.) ;
#18444=EDGE_CURVE('',#14549,#14550,#7710,.T.) ;
#18445=EDGE_CURVE('',#14550,#14551,#7711,.T.) ;
#18446=EDGE_CURVE('',#14551,#14552,#7712,.T.) ;
#18447=EDGE_CURVE('',#14552,#14549,#7713,.T.) ;
#18448=EDGE_CURVE('',#14553,#14550,#11922,.T.) ;
#18449=EDGE_CURVE('',#14550,#14554,#11923,.T.) ;
#18450=EDGE_CURVE('',#14553,#14554,#11924,.T.) ;
#18451=EDGE_CURVE('',#14555,#14549,#11925,.T.) ;
#18452=EDGE_CURVE('',#14549,#14287,#11926,.T.) ;
#18453=EDGE_CURVE('',#14555,#14287,#11927,.T.) ;
#18454=EDGE_CURVE('',#14554,#14555,#7714,.T.) ;
#18455=EDGE_CURVE('',#14286,#14552,#11928,.F.) ;
#18456=EDGE_CURVE('',#14284,#14553,#7715,.T.) ;
#18457=EDGE_CURVE('',#14551,#14284,#11929,.F.) ;
#18458=EDGE_CURVE('',#14283,#14551,#11930,.F.) ;
#18459=EDGE_CURVE('',#14552,#14285,#11931,.F.) ;
#18460=EDGE_CURVE('',#14081,#14446,#11932,.T.) ;
#18461=EDGE_CURVE('',#14556,#14557,#11933,.T.) ;
#18462=EDGE_CURVE('',#14441,#14556,#7716,.T.) ;
#18463=EDGE_CURVE('',#14558,#14441,#11934,.T.) ;
#18464=EDGE_CURVE('',#14557,#14558,#7717,.T.) ;
#18465=EDGE_CURVE('',#14559,#14081,#11935,.F.) ;
#18466=EDGE_CURVE('',#14445,#14559,#11936,.T.) ;
#18467=EDGE_CURVE('',#14560,#14444,#11937,.T.) ;
#18468=EDGE_CURVE('',#14559,#14560,#7718,.T.) ;
#18469=EDGE_CURVE('',#14080,#14561,#11938,.F.) ;
#18470=EDGE_CURVE('',#14561,#14074,#11939,.T.) ;
#18471=EDGE_CURVE('',#14562,#14563,#11940,.F.) ;
#18472=EDGE_CURVE('',#14563,#14443,#11941,.T.) ;
#18473=EDGE_CURVE('',#14442,#14562,#11942,.T.) ;
#18474=EDGE_CURVE('',#14562,#14068,#7719,.T.) ;
#18475=EDGE_CURVE('',#14440,#14558,#11943,.T.) ;
#18476=EDGE_CURVE('',#14558,#14563,#7720,.T.) ;
#18477=EDGE_CURVE('',#14564,#14072,#11944,.F.) ;
#18478=EDGE_CURVE('',#14079,#14564,#11945,.T.) ;
#18479=EDGE_CURVE('',#14557,#14078,#11946,.T.) ;
#18480=EDGE_CURVE('',#14564,#14557,#7721,.T.) ;
#18481=EDGE_CURVE('',#14563,#14564,#7722,.T.) ;
#18482=EDGE_CURVE('',#14072,#14562,#7723,.T.) ;
#18483=EDGE_CURVE('',#14075,#14565,#11947,.T.) ;
#18484=EDGE_CURVE('',#14565,#14561,#7724,.T.) ;
#18485=EDGE_CURVE('',#14561,#14559,#7725,.T.) ;
#18486=EDGE_CURVE('',#14556,#14078,#11948,.T.) ;
#18487=EDGE_CURVE('',#14565,#14448,#11949,.T.) ;
#18488=EDGE_CURVE('',#14560,#14565,#7726,.T.) ;
#18489=EDGE_CURVE('',#14447,#14560,#11950,.T.) ;
#18490=EDGE_CURVE('',#14075,#14448,#11951,.T.) ;
#18491=EDGE_CURVE('',#14566,#14567,#7727,.T.) ;
#18492=EDGE_CURVE('',#14567,#14568,#7728,.T.) ;
#18493=EDGE_CURVE('',#14568,#14569,#7729,.T.) ;
#18494=EDGE_CURVE('',#14569,#14566,#7730,.T.) ;
#18495=EDGE_CURVE('',#14570,#14567,#11952,.T.) ;
#18496=EDGE_CURVE('',#14567,#14571,#11953,.T.) ;
#18497=EDGE_CURVE('',#14570,#14571,#11954,.T.) ;
#18498=EDGE_CURVE('',#14572,#14566,#11955,.T.) ;
#18499=EDGE_CURVE('',#14566,#14266,#11956,.T.) ;
#18500=EDGE_CURVE('',#14572,#14266,#11957,.T.) ;
#18501=EDGE_CURVE('',#14571,#14572,#7731,.T.) ;
#18502=EDGE_CURVE('',#14265,#14569,#11958,.F.) ;
#18503=EDGE_CURVE('',#14263,#14570,#7732,.T.) ;
#18504=EDGE_CURVE('',#14568,#14263,#11959,.F.) ;
#18505=EDGE_CURVE('',#14262,#14568,#11960,.F.) ;
#18506=EDGE_CURVE('',#14569,#14264,#11961,.F.) ;
#18507=EDGE_CURVE('',#14062,#14423,#11962,.T.) ;
#18508=EDGE_CURVE('',#14573,#14574,#11963,.T.) ;
#18509=EDGE_CURVE('',#14418,#14573,#7733,.T.) ;
#18510=EDGE_CURVE('',#14575,#14418,#11964,.T.) ;
#18511=EDGE_CURVE('',#14574,#14575,#7734,.T.) ;
#18512=EDGE_CURVE('',#14576,#14062,#11965,.F.) ;
#18513=EDGE_CURVE('',#14422,#14576,#11966,.T.) ;
#18514=EDGE_CURVE('',#14577,#14421,#11967,.T.) ;
#18515=EDGE_CURVE('',#14576,#14577,#7735,.T.) ;
#18516=EDGE_CURVE('',#14061,#14578,#11968,.F.) ;
#18517=EDGE_CURVE('',#14578,#14055,#11969,.T.) ;
#18518=EDGE_CURVE('',#14579,#14580,#11970,.F.) ;
#18519=EDGE_CURVE('',#14580,#14420,#11971,.T.) ;
#18520=EDGE_CURVE('',#14419,#14579,#11972,.T.) ;
#18521=EDGE_CURVE('',#14579,#14049,#7736,.T.) ;
#18522=EDGE_CURVE('',#14417,#14575,#11973,.T.) ;
#18523=EDGE_CURVE('',#14575,#14580,#7737,.T.) ;
#18524=EDGE_CURVE('',#14581,#14053,#11974,.F.) ;
#18525=EDGE_CURVE('',#14060,#14581,#11975,.T.) ;
#18526=EDGE_CURVE('',#14574,#14059,#11976,.T.) ;
#18527=EDGE_CURVE('',#14581,#14574,#7738,.T.) ;
#18528=EDGE_CURVE('',#14580,#14581,#7739,.T.) ;
#18529=EDGE_CURVE('',#14053,#14579,#7740,.T.) ;
#18530=EDGE_CURVE('',#14056,#14582,#11977,.T.) ;
#18531=EDGE_CURVE('',#14582,#14578,#7741,.T.) ;
#18532=EDGE_CURVE('',#14578,#14576,#7742,.T.) ;
#18533=EDGE_CURVE('',#14573,#14059,#11978,.T.) ;
#18534=EDGE_CURVE('',#14582,#14425,#11979,.T.) ;
#18535=EDGE_CURVE('',#14577,#14582,#7743,.T.) ;
#18536=EDGE_CURVE('',#14424,#14577,#11980,.T.) ;
#18537=EDGE_CURVE('',#14056,#14425,#11981,.T.) ;
#18538=EDGE_CURVE('',#14583,#14584,#7744,.T.) ;
#18539=EDGE_CURVE('',#14584,#14585,#7745,.T.) ;
#18540=EDGE_CURVE('',#14585,#14586,#7746,.T.) ;
#18541=EDGE_CURVE('',#14586,#14583,#7747,.T.) ;
#18542=EDGE_CURVE('',#14587,#14584,#11982,.T.) ;
#18543=EDGE_CURVE('',#14584,#14588,#11983,.T.) ;
#18544=EDGE_CURVE('',#14587,#14588,#11984,.T.) ;
#18545=EDGE_CURVE('',#14589,#14583,#11985,.T.) ;
#18546=EDGE_CURVE('',#14583,#14245,#11986,.T.) ;
#18547=EDGE_CURVE('',#14589,#14245,#11987,.T.) ;
#18548=EDGE_CURVE('',#14588,#14589,#7748,.T.) ;
#18549=EDGE_CURVE('',#14244,#14586,#11988,.F.) ;
#18550=EDGE_CURVE('',#14242,#14587,#7749,.T.) ;
#18551=EDGE_CURVE('',#14585,#14242,#11989,.F.) ;
#18552=EDGE_CURVE('',#14241,#14585,#11990,.F.) ;
#18553=EDGE_CURVE('',#14586,#14243,#11991,.F.) ;
#18554=EDGE_CURVE('',#14043,#14400,#11992,.T.) ;
#18555=EDGE_CURVE('',#14590,#14591,#11993,.T.) ;
#18556=EDGE_CURVE('',#14395,#14590,#7750,.T.) ;
#18557=EDGE_CURVE('',#14592,#14395,#11994,.T.) ;
#18558=EDGE_CURVE('',#14591,#14592,#7751,.T.) ;
#18559=EDGE_CURVE('',#14593,#14043,#11995,.F.) ;
#18560=EDGE_CURVE('',#14399,#14593,#11996,.T.) ;
#18561=EDGE_CURVE('',#14594,#14398,#11997,.T.) ;
#18562=EDGE_CURVE('',#14593,#14594,#7752,.T.) ;
#18563=EDGE_CURVE('',#14042,#14595,#11998,.F.) ;
#18564=EDGE_CURVE('',#14595,#14036,#11999,.T.) ;
#18565=EDGE_CURVE('',#14596,#14597,#12000,.F.) ;
#18566=EDGE_CURVE('',#14597,#14397,#12001,.T.) ;
#18567=EDGE_CURVE('',#14396,#14596,#12002,.T.) ;
#18568=EDGE_CURVE('',#14596,#14030,#7753,.T.) ;
#18569=EDGE_CURVE('',#14394,#14592,#12003,.T.) ;
#18570=EDGE_CURVE('',#14592,#14597,#7754,.T.) ;
#18571=EDGE_CURVE('',#14598,#14034,#12004,.F.) ;
#18572=EDGE_CURVE('',#14041,#14598,#12005,.T.) ;
#18573=EDGE_CURVE('',#14591,#14040,#12006,.T.) ;
#18574=EDGE_CURVE('',#14598,#14591,#7755,.T.) ;
#18575=EDGE_CURVE('',#14597,#14598,#7756,.T.) ;
#18576=EDGE_CURVE('',#14034,#14596,#7757,.T.) ;
#18577=EDGE_CURVE('',#14037,#14599,#12007,.T.) ;
#18578=EDGE_CURVE('',#14599,#14595,#7758,.T.) ;
#18579=EDGE_CURVE('',#14595,#14593,#7759,.T.) ;
#18580=EDGE_CURVE('',#14590,#14040,#12008,.T.) ;
#18581=EDGE_CURVE('',#14599,#14402,#12009,.T.) ;
#18582=EDGE_CURVE('',#14594,#14599,#7760,.T.) ;
#18583=EDGE_CURVE('',#14401,#14594,#12010,.T.) ;
#18584=EDGE_CURVE('',#14037,#14402,#12011,.T.) ;
#18585=EDGE_CURVE('',#14600,#14601,#7761,.T.) ;
#18586=EDGE_CURVE('',#14601,#14602,#7762,.T.) ;
#18587=EDGE_CURVE('',#14602,#14603,#7763,.T.) ;
#18588=EDGE_CURVE('',#14603,#14600,#7764,.T.) ;
#18589=EDGE_CURVE('',#14604,#14601,#12012,.T.) ;
#18590=EDGE_CURVE('',#14601,#14605,#12013,.T.) ;
#18591=EDGE_CURVE('',#14604,#14605,#12014,.T.) ;
#18592=EDGE_CURVE('',#14606,#14600,#12015,.T.) ;
#18593=EDGE_CURVE('',#14600,#14224,#12016,.T.) ;
#18594=EDGE_CURVE('',#14606,#14224,#12017,.T.) ;
#18595=EDGE_CURVE('',#14605,#14606,#7765,.T.) ;
#18596=EDGE_CURVE('',#14223,#14603,#12018,.F.) ;
#18597=EDGE_CURVE('',#14221,#14604,#7766,.T.) ;
#18598=EDGE_CURVE('',#14602,#14221,#12019,.F.) ;
#18599=EDGE_CURVE('',#14220,#14602,#12020,.F.) ;
#18600=EDGE_CURVE('',#14603,#14222,#12021,.F.) ;
#18601=EDGE_CURVE('',#14024,#14377,#12022,.T.) ;
#18602=EDGE_CURVE('',#14607,#14608,#12023,.T.) ;
#18603=EDGE_CURVE('',#14372,#14607,#7767,.T.) ;
#18604=EDGE_CURVE('',#14609,#14372,#12024,.T.) ;
#18605=EDGE_CURVE('',#14608,#14609,#7768,.T.) ;
#18606=EDGE_CURVE('',#14610,#14024,#12025,.F.) ;
#18607=EDGE_CURVE('',#14376,#14610,#12026,.T.) ;
#18608=EDGE_CURVE('',#14611,#14375,#12027,.T.) ;
#18609=EDGE_CURVE('',#14610,#14611,#7769,.T.) ;
#18610=EDGE_CURVE('',#14023,#14612,#12028,.F.) ;
#18611=EDGE_CURVE('',#14612,#14017,#12029,.T.) ;
#18612=EDGE_CURVE('',#14613,#14614,#12030,.F.) ;
#18613=EDGE_CURVE('',#14614,#14374,#12031,.T.) ;
#18614=EDGE_CURVE('',#14373,#14613,#12032,.T.) ;
#18615=EDGE_CURVE('',#14613,#14011,#7770,.T.) ;
#18616=EDGE_CURVE('',#14371,#14609,#12033,.T.) ;
#18617=EDGE_CURVE('',#14609,#14614,#7771,.T.) ;
#18618=EDGE_CURVE('',#14615,#14015,#12034,.F.) ;
#18619=EDGE_CURVE('',#14022,#14615,#12035,.T.) ;
#18620=EDGE_CURVE('',#14608,#14021,#12036,.T.) ;
#18621=EDGE_CURVE('',#14615,#14608,#7772,.T.) ;
#18622=EDGE_CURVE('',#14614,#14615,#7773,.T.) ;
#18623=EDGE_CURVE('',#14015,#14613,#7774,.T.) ;
#18624=EDGE_CURVE('',#14018,#14616,#12037,.T.) ;
#18625=EDGE_CURVE('',#14616,#14612,#7775,.T.) ;
#18626=EDGE_CURVE('',#14612,#14610,#7776,.T.) ;
#18627=EDGE_CURVE('',#14607,#14021,#12038,.T.) ;
#18628=EDGE_CURVE('',#14616,#14379,#12039,.T.) ;
#18629=EDGE_CURVE('',#14611,#14616,#7777,.T.) ;
#18630=EDGE_CURVE('',#14378,#14611,#12040,.T.) ;
#18631=EDGE_CURVE('',#14018,#14379,#12041,.T.) ;
#18632=EDGE_CURVE('',#14617,#14618,#7778,.T.) ;
#18633=EDGE_CURVE('',#14618,#14619,#7779,.T.) ;
#18634=EDGE_CURVE('',#14619,#14620,#7780,.T.) ;
#18635=EDGE_CURVE('',#14620,#14617,#7781,.T.) ;
#18636=EDGE_CURVE('',#14621,#14618,#12042,.T.) ;
#18637=EDGE_CURVE('',#14618,#14622,#12043,.T.) ;
#18638=EDGE_CURVE('',#14621,#14622,#12044,.T.) ;
#18639=EDGE_CURVE('',#14623,#14617,#12045,.T.) ;
#18640=EDGE_CURVE('',#14617,#14203,#12046,.T.) ;
#18641=EDGE_CURVE('',#14623,#14203,#12047,.T.) ;
#18642=EDGE_CURVE('',#14622,#14623,#7782,.T.) ;
#18643=EDGE_CURVE('',#14202,#14620,#12048,.F.) ;
#18644=EDGE_CURVE('',#14200,#14621,#7783,.T.) ;
#18645=EDGE_CURVE('',#14619,#14200,#12049,.F.) ;
#18646=EDGE_CURVE('',#14199,#14619,#12050,.F.) ;
#18647=EDGE_CURVE('',#14620,#14201,#12051,.F.) ;
#18648=EDGE_CURVE('',#14005,#14354,#12052,.T.) ;
#18649=EDGE_CURVE('',#14624,#14625,#12053,.T.) ;
#18650=EDGE_CURVE('',#14349,#14624,#7784,.T.) ;
#18651=EDGE_CURVE('',#14626,#14349,#12054,.T.) ;
#18652=EDGE_CURVE('',#14625,#14626,#7785,.T.) ;
#18653=EDGE_CURVE('',#14627,#14005,#12055,.F.) ;
#18654=EDGE_CURVE('',#14353,#14627,#12056,.T.) ;
#18655=EDGE_CURVE('',#14628,#14352,#12057,.T.) ;
#18656=EDGE_CURVE('',#14627,#14628,#7786,.T.) ;
#18657=EDGE_CURVE('',#14004,#14629,#12058,.F.) ;
#18658=EDGE_CURVE('',#14629,#13998,#12059,.T.) ;
#18659=EDGE_CURVE('',#14630,#14631,#12060,.F.) ;
#18660=EDGE_CURVE('',#14631,#14351,#12061,.T.) ;
#18661=EDGE_CURVE('',#14350,#14630,#12062,.T.) ;
#18662=EDGE_CURVE('',#14630,#13992,#7787,.T.) ;
#18663=EDGE_CURVE('',#14348,#14626,#12063,.T.) ;
#18664=EDGE_CURVE('',#14626,#14631,#7788,.T.) ;
#18665=EDGE_CURVE('',#14632,#13996,#12064,.F.) ;
#18666=EDGE_CURVE('',#14003,#14632,#12065,.T.) ;
#18667=EDGE_CURVE('',#14625,#14002,#12066,.T.) ;
#18668=EDGE_CURVE('',#14632,#14625,#7789,.T.) ;
#18669=EDGE_CURVE('',#14631,#14632,#7790,.T.) ;
#18670=EDGE_CURVE('',#13996,#14630,#7791,.T.) ;
#18671=EDGE_CURVE('',#13999,#14633,#12067,.T.) ;
#18672=EDGE_CURVE('',#14633,#14629,#7792,.T.) ;
#18673=EDGE_CURVE('',#14629,#14627,#7793,.T.) ;
#18674=EDGE_CURVE('',#14624,#14002,#12068,.T.) ;
#18675=EDGE_CURVE('',#14633,#14356,#12069,.T.) ;
#18676=EDGE_CURVE('',#14628,#14633,#7794,.T.) ;
#18677=EDGE_CURVE('',#14355,#14628,#12070,.T.) ;
#18678=EDGE_CURVE('',#13999,#14356,#12071,.T.) ;
#18679=EDGE_CURVE('',#14634,#14635,#7795,.T.) ;
#18680=EDGE_CURVE('',#14635,#14636,#7796,.T.) ;
#18681=EDGE_CURVE('',#14636,#14637,#7797,.T.) ;
#18682=EDGE_CURVE('',#14637,#14634,#7798,.T.) ;
#18683=EDGE_CURVE('',#14638,#14635,#12072,.T.) ;
#18684=EDGE_CURVE('',#14635,#14639,#12073,.T.) ;
#18685=EDGE_CURVE('',#14638,#14639,#12074,.T.) ;
#18686=EDGE_CURVE('',#14640,#14634,#12075,.T.) ;
#18687=EDGE_CURVE('',#14634,#14182,#12076,.T.) ;
#18688=EDGE_CURVE('',#14640,#14182,#12077,.T.) ;
#18689=EDGE_CURVE('',#14639,#14640,#7799,.T.) ;
#18690=EDGE_CURVE('',#14181,#14637,#12078,.F.) ;
#18691=EDGE_CURVE('',#14179,#14638,#7800,.T.) ;
#18692=EDGE_CURVE('',#14636,#14179,#12079,.F.) ;
#18693=EDGE_CURVE('',#14178,#14636,#12080,.F.) ;
#18694=EDGE_CURVE('',#14637,#14180,#12081,.F.) ;
#18695=EDGE_CURVE('',#13986,#14331,#12082,.T.) ;
#18696=EDGE_CURVE('',#14641,#14642,#12083,.T.) ;
#18697=EDGE_CURVE('',#14326,#14641,#7801,.T.) ;
#18698=EDGE_CURVE('',#14643,#14326,#12084,.T.) ;
#18699=EDGE_CURVE('',#14642,#14643,#7802,.T.) ;
#18700=EDGE_CURVE('',#14644,#13986,#12085,.F.) ;
#18701=EDGE_CURVE('',#14330,#14644,#12086,.T.) ;
#18702=EDGE_CURVE('',#14645,#14329,#12087,.T.) ;
#18703=EDGE_CURVE('',#14644,#14645,#7803,.T.) ;
#18704=EDGE_CURVE('',#13985,#14646,#12088,.F.) ;
#18705=EDGE_CURVE('',#14646,#13979,#12089,.T.) ;
#18706=EDGE_CURVE('',#14647,#14648,#12090,.F.) ;
#18707=EDGE_CURVE('',#14648,#14328,#12091,.T.) ;
#18708=EDGE_CURVE('',#14327,#14647,#12092,.T.) ;
#18709=EDGE_CURVE('',#14647,#13973,#7804,.T.) ;
#18710=EDGE_CURVE('',#14325,#14643,#12093,.T.) ;
#18711=EDGE_CURVE('',#14643,#14648,#7805,.T.) ;
#18712=EDGE_CURVE('',#14649,#13977,#12094,.F.) ;
#18713=EDGE_CURVE('',#13984,#14649,#12095,.T.) ;
#18714=EDGE_CURVE('',#14642,#13983,#12096,.T.) ;
#18715=EDGE_CURVE('',#14649,#14642,#7806,.T.) ;
#18716=EDGE_CURVE('',#14648,#14649,#7807,.T.) ;
#18717=EDGE_CURVE('',#13977,#14647,#7808,.T.) ;
#18718=EDGE_CURVE('',#13980,#14650,#12097,.T.) ;
#18719=EDGE_CURVE('',#14650,#14646,#7809,.T.) ;
#18720=EDGE_CURVE('',#14646,#14644,#7810,.T.) ;
#18721=EDGE_CURVE('',#14641,#13983,#12098,.T.) ;
#18722=EDGE_CURVE('',#14650,#14333,#12099,.T.) ;
#18723=EDGE_CURVE('',#14645,#14650,#7811,.T.) ;
#18724=EDGE_CURVE('',#14332,#14645,#12100,.T.) ;
#18725=EDGE_CURVE('',#13980,#14333,#12101,.T.) ;
#18726=EDGE_CURVE('',#14651,#14652,#7812,.T.) ;
#18727=EDGE_CURVE('',#14652,#14653,#7813,.T.) ;
#18728=EDGE_CURVE('',#14653,#14654,#7814,.T.) ;
#18729=EDGE_CURVE('',#14654,#14651,#7815,.T.) ;
#18730=EDGE_CURVE('',#14655,#14652,#12102,.T.) ;
#18731=EDGE_CURVE('',#14652,#14656,#12103,.T.) ;
#18732=EDGE_CURVE('',#14655,#14656,#12104,.T.) ;
#18733=EDGE_CURVE('',#14657,#14651,#12105,.T.) ;
#18734=EDGE_CURVE('',#14651,#14161,#12106,.T.) ;
#18735=EDGE_CURVE('',#14657,#14161,#12107,.T.) ;
#18736=EDGE_CURVE('',#14656,#14657,#7816,.T.) ;
#18737=EDGE_CURVE('',#14160,#14654,#12108,.F.) ;
#18738=EDGE_CURVE('',#14158,#14655,#7817,.T.) ;
#18739=EDGE_CURVE('',#14653,#14158,#12109,.F.) ;
#18740=EDGE_CURVE('',#14157,#14653,#12110,.F.) ;
#18741=EDGE_CURVE('',#14654,#14159,#12111,.F.) ;
#18742=EDGE_CURVE('',#13967,#14308,#12112,.T.) ;
#18743=EDGE_CURVE('',#14658,#14659,#12113,.T.) ;
#18744=EDGE_CURVE('',#14303,#14658,#7818,.T.) ;
#18745=EDGE_CURVE('',#14660,#14303,#12114,.T.) ;
#18746=EDGE_CURVE('',#14659,#14660,#7819,.T.) ;
#18747=EDGE_CURVE('',#14661,#13967,#12115,.F.) ;
#18748=EDGE_CURVE('',#14307,#14661,#12116,.T.) ;
#18749=EDGE_CURVE('',#14662,#14306,#12117,.T.) ;
#18750=EDGE_CURVE('',#14661,#14662,#7820,.T.) ;
#18751=EDGE_CURVE('',#13966,#14663,#12118,.F.) ;
#18752=EDGE_CURVE('',#14663,#13960,#12119,.T.) ;
#18753=EDGE_CURVE('',#14664,#14665,#12120,.F.) ;
#18754=EDGE_CURVE('',#14665,#14305,#12121,.T.) ;
#18755=EDGE_CURVE('',#14304,#14664,#12122,.T.) ;
#18756=EDGE_CURVE('',#14664,#13954,#7821,.T.) ;
#18757=EDGE_CURVE('',#14302,#14660,#12123,.T.) ;
#18758=EDGE_CURVE('',#14660,#14665,#7822,.T.) ;
#18759=EDGE_CURVE('',#14666,#13958,#12124,.F.) ;
#18760=EDGE_CURVE('',#13965,#14666,#12125,.T.) ;
#18761=EDGE_CURVE('',#14659,#13964,#12126,.T.) ;
#18762=EDGE_CURVE('',#14666,#14659,#7823,.T.) ;
#18763=EDGE_CURVE('',#14665,#14666,#7824,.T.) ;
#18764=EDGE_CURVE('',#13958,#14664,#7825,.T.) ;
#18765=EDGE_CURVE('',#13961,#14667,#12127,.T.) ;
#18766=EDGE_CURVE('',#14667,#14663,#7826,.T.) ;
#18767=EDGE_CURVE('',#14663,#14661,#7827,.T.) ;
#18768=EDGE_CURVE('',#14658,#13964,#12128,.T.) ;
#18769=EDGE_CURVE('',#14667,#14310,#12129,.T.) ;
#18770=EDGE_CURVE('',#14662,#14667,#7828,.T.) ;
#18771=EDGE_CURVE('',#14309,#14662,#12130,.T.) ;
#18772=EDGE_CURVE('',#13961,#14310,#12131,.T.) ;
#18773=EDGE_CURVE('',#14668,#14669,#7829,.T.) ;
#18774=EDGE_CURVE('',#14669,#14670,#7830,.T.) ;
#18775=EDGE_CURVE('',#14670,#14671,#7831,.T.) ;
#18776=EDGE_CURVE('',#14671,#14668,#7832,.T.) ;
#18777=EDGE_CURVE('',#14672,#14669,#12132,.T.) ;
#18778=EDGE_CURVE('',#14669,#14673,#12133,.T.) ;
#18779=EDGE_CURVE('',#14672,#14673,#12134,.T.) ;
#18780=EDGE_CURVE('',#14674,#14668,#12135,.T.) ;
#18781=EDGE_CURVE('',#14668,#14140,#12136,.T.) ;
#18782=EDGE_CURVE('',#14674,#14140,#12137,.T.) ;
#18783=EDGE_CURVE('',#14673,#14674,#7833,.T.) ;
#18784=EDGE_CURVE('',#14139,#14671,#12138,.F.) ;
#18785=EDGE_CURVE('',#14137,#14672,#7834,.T.) ;
#18786=EDGE_CURVE('',#14670,#14137,#12139,.F.) ;
#18787=EDGE_CURVE('',#14136,#14670,#12140,.F.) ;
#18788=EDGE_CURVE('',#14671,#14138,#12141,.F.) ;
#18789=EDGE_CURVE('',#13769,#13812,#7835,.T.) ;
#18790=EDGE_CURVE('',#13811,#13770,#7836,.T.) ;
#18791=EDGE_CURVE('',#13826,#13774,#7837,.T.) ;
#18792=EDGE_CURVE('',#13773,#13827,#7838,.T.) ;
#18793=EDGE_CURVE('',#13841,#13778,#7839,.T.) ;
#18794=EDGE_CURVE('',#13777,#13842,#7840,.T.) ;
#18795=EDGE_CURVE('',#13856,#13782,#7841,.T.) ;
#18796=EDGE_CURVE('',#13781,#13857,#7842,.T.) ;
#18797=EDGE_CURVE('',#13870,#13786,#7843,.T.) ;
#18798=EDGE_CURVE('',#13785,#13869,#7844,.T.) ;
#18799=EDGE_CURVE('',#13885,#13790,#7845,.T.) ;
#18800=EDGE_CURVE('',#13789,#13884,#7846,.T.) ;
#18801=EDGE_CURVE('',#13900,#13794,#7847,.T.) ;
#18802=EDGE_CURVE('',#13793,#13899,#7848,.T.) ;
#18803=EDGE_CURVE('',#13915,#13798,#7849,.T.) ;
#18804=EDGE_CURVE('',#13797,#13914,#7850,.T.) ;
#18805=EDGE_CURVE('',#13929,#13802,#7851,.T.) ;
#18806=EDGE_CURVE('',#13801,#13928,#7852,.T.) ;
#18807=EDGE_CURVE('',#13779,#13839,#7853,.T.) ;
#18808=EDGE_CURVE('',#13840,#13776,#7854,.T.) ;
#18809=EDGE_CURVE('',#13901,#13792,#7855,.T.) ;
#18810=EDGE_CURVE('',#13795,#13902,#7856,.T.) ;
#18811=EDGE_CURVE('',#13916,#13796,#7857,.T.) ;
#18812=EDGE_CURVE('',#13799,#13917,#7858,.T.) ;
#18813=EDGE_CURVE('',#13783,#13854,#7859,.T.) ;
#18814=EDGE_CURVE('',#13855,#13780,#7860,.T.) ;
#18815=EDGE_CURVE('',#13775,#13824,#7861,.T.) ;
#18816=EDGE_CURVE('',#13825,#13772,#7862,.T.) ;
#18817=EDGE_CURVE('',#13886,#13788,#7863,.T.) ;
#18818=EDGE_CURVE('',#13791,#13887,#7864,.T.) ;
#18819=EDGE_CURVE('',#13930,#13800,#7865,.T.) ;
#18820=EDGE_CURVE('',#13803,#13931,#7866,.T.) ;
#18821=EDGE_CURVE('',#13871,#13784,#7867,.T.) ;
#18822=EDGE_CURVE('',#13787,#13872,#7868,.T.) ;
#18823=EDGE_CURVE('',#13771,#13809,#7869,.T.) ;
#18824=EDGE_CURVE('',#13810,#13768,#7870,.T.) ;
#18825=EDGE_CURVE('',#14675,#14676,#7871,.T.) ;
#18826=EDGE_CURVE('',#14677,#14676,#7872,.T.) ;
#18827=EDGE_CURVE('',#14677,#14678,#7873,.T.) ;
#18828=EDGE_CURVE('',#14679,#14678,#7874,.T.) ;
#18829=EDGE_CURVE('',#14679,#14680,#7875,.T.) ;
#18830=EDGE_CURVE('',#14681,#14680,#7876,.T.) ;
#18831=EDGE_CURVE('',#14681,#14682,#7877,.T.) ;
#18832=EDGE_CURVE('',#14683,#14682,#7878,.T.) ;
#18833=EDGE_CURVE('',#14683,#14684,#7879,.T.) ;
#18834=EDGE_CURVE('',#14685,#14684,#7880,.T.) ;
#18835=EDGE_CURVE('',#14685,#14686,#7881,.T.) ;
#18836=EDGE_CURVE('',#14687,#14686,#7882,.T.) ;
#18837=EDGE_CURVE('',#14687,#14688,#7883,.T.) ;
#18838=EDGE_CURVE('',#14689,#14688,#7884,.T.) ;
#18839=EDGE_CURVE('',#14689,#14690,#7885,.T.) ;
#18840=EDGE_CURVE('',#14691,#14690,#7886,.T.) ;
#18841=EDGE_CURVE('',#14691,#14692,#7887,.T.) ;
#18842=EDGE_CURVE('',#14693,#14692,#7888,.T.) ;
#18843=EDGE_CURVE('',#14694,#14693,#7889,.T.) ;
#18844=EDGE_CURVE('',#14695,#14694,#7890,.T.) ;
#18845=EDGE_CURVE('',#14695,#14696,#7891,.T.) ;
#18846=EDGE_CURVE('',#14697,#14696,#7892,.T.) ;
#18847=EDGE_CURVE('',#14698,#14697,#7893,.T.) ;
#18848=EDGE_CURVE('',#14699,#14698,#7894,.T.) ;
#18849=EDGE_CURVE('',#14699,#14700,#7895,.T.) ;
#18850=EDGE_CURVE('',#14701,#14700,#7896,.T.) ;
#18851=EDGE_CURVE('',#14702,#14701,#7897,.T.) ;
#18852=EDGE_CURVE('',#14703,#14702,#7898,.T.) ;
#18853=EDGE_CURVE('',#14703,#14704,#7899,.T.) ;
#18854=EDGE_CURVE('',#14705,#14704,#7900,.T.) ;
#18855=EDGE_CURVE('',#14706,#14705,#7901,.T.) ;
#18856=EDGE_CURVE('',#14707,#14706,#7902,.T.) ;
#18857=EDGE_CURVE('',#14707,#14708,#7903,.T.) ;
#18858=EDGE_CURVE('',#14709,#14708,#7904,.T.) ;
#18859=EDGE_CURVE('',#14709,#14710,#7905,.T.) ;
#18860=EDGE_CURVE('',#14711,#14710,#7906,.T.) ;
#18861=EDGE_CURVE('',#14712,#14711,#7907,.T.) ;
#18862=EDGE_CURVE('',#14713,#14712,#7908,.T.) ;
#18863=EDGE_CURVE('',#14714,#14713,#7909,.T.) ;
#18864=EDGE_CURVE('',#14675,#14714,#7910,.T.) ;
#18865=EDGE_CURVE('',#14676,#14715,#130,.T.) ;
#18866=EDGE_CURVE('',#14715,#14716,#7911,.T.) ;
#18867=EDGE_CURVE('',#14716,#14677,#131,.T.) ;
#18868=EDGE_CURVE('',#14494,#14675,#7912,.T.) ;
#18869=EDGE_CURVE('',#14717,#14493,#7913,.F.) ;
#18870=EDGE_CURVE('',#14715,#14717,#7914,.T.) ;
#18871=EDGE_CURVE('',#14718,#14719,#7915,.T.) ;
#18872=EDGE_CURVE('',#14719,#14681,#132,.T.) ;
#18873=EDGE_CURVE('',#14680,#14718,#133,.T.) ;
#18874=EDGE_CURVE('',#14684,#14720,#134,.T.) ;
#18875=EDGE_CURVE('',#14720,#14721,#7916,.T.) ;
#18876=EDGE_CURVE('',#14721,#14685,#135,.T.) ;
#18877=EDGE_CURVE('',#14688,#14722,#136,.T.) ;
#18878=EDGE_CURVE('',#14722,#14723,#7917,.T.) ;
#18879=EDGE_CURVE('',#14723,#14689,#137,.T.) ;
#18880=EDGE_CURVE('',#14724,#14725,#7918,.T.) ;
#18881=EDGE_CURVE('',#14725,#14693,#138,.T.) ;
#18882=EDGE_CURVE('',#14692,#14724,#139,.T.) ;
#18883=EDGE_CURVE('',#14726,#14727,#7919,.T.) ;
#18884=EDGE_CURVE('',#14727,#14697,#140,.T.) ;
#18885=EDGE_CURVE('',#14696,#14726,#141,.T.) ;
#18886=EDGE_CURVE('',#14728,#14729,#7920,.T.) ;
#18887=EDGE_CURVE('',#14729,#14701,#142,.T.) ;
#18888=EDGE_CURVE('',#14700,#14728,#143,.T.) ;
#18889=EDGE_CURVE('',#14704,#14730,#144,.T.) ;
#18890=EDGE_CURVE('',#14730,#14731,#7921,.T.) ;
#18891=EDGE_CURVE('',#14731,#14705,#145,.T.) ;
#18892=EDGE_CURVE('',#14732,#14733,#7922,.T.) ;
#18893=EDGE_CURVE('',#14733,#14709,#146,.T.) ;
#18894=EDGE_CURVE('',#14708,#14732,#147,.T.) ;
#18895=EDGE_CURVE('',#14734,#14713,#148,.T.) ;
#18896=EDGE_CURVE('',#14735,#14734,#7923,.T.) ;
#18897=EDGE_CURVE('',#14496,#14735,#7924,.F.) ;
#18898=EDGE_CURVE('',#14714,#14495,#7925,.T.) ;
#18899=EDGE_CURVE('',#14736,#14734,#7926,.T.) ;
#18900=EDGE_CURVE('',#14712,#14736,#149,.T.) ;
#18901=EDGE_CURVE('',#14735,#14717,#7927,.T.) ;
#18902=EDGE_CURVE('',#14737,#14738,#7928,.F.) ;
#18903=EDGE_CURVE('',#14738,#14739,#7929,.T.) ;
#18904=EDGE_CURVE('',#14739,#14740,#7930,.F.) ;
#18905=EDGE_CURVE('',#14740,#14737,#7931,.T.) ;
#18906=EDGE_CURVE('',#14741,#14742,#7932,.F.) ;
#18907=EDGE_CURVE('',#14742,#14743,#7933,.T.) ;
#18908=EDGE_CURVE('',#14743,#14744,#7934,.F.) ;
#18909=EDGE_CURVE('',#14744,#14741,#7935,.T.) ;
#18910=EDGE_CURVE('',#14745,#14746,#7936,.F.) ;
#18911=EDGE_CURVE('',#14746,#14747,#7937,.T.) ;
#18912=EDGE_CURVE('',#14747,#14748,#7938,.F.) ;
#18913=EDGE_CURVE('',#14748,#14745,#7939,.T.) ;
#18914=EDGE_CURVE('',#14749,#14750,#7940,.F.) ;
#18915=EDGE_CURVE('',#14750,#14751,#7941,.T.) ;
#18916=EDGE_CURVE('',#14751,#14752,#7942,.F.) ;
#18917=EDGE_CURVE('',#14752,#14749,#7943,.T.) ;
#18918=EDGE_CURVE('',#14753,#14754,#7944,.F.) ;
#18919=EDGE_CURVE('',#14754,#14755,#7945,.T.) ;
#18920=EDGE_CURVE('',#14755,#14756,#7946,.F.) ;
#18921=EDGE_CURVE('',#14756,#14753,#7947,.T.) ;
#18922=EDGE_CURVE('',#14757,#14758,#7948,.F.) ;
#18923=EDGE_CURVE('',#14758,#14759,#7949,.T.) ;
#18924=EDGE_CURVE('',#14759,#14760,#7950,.F.) ;
#18925=EDGE_CURVE('',#14760,#14757,#7951,.T.) ;
#18926=EDGE_CURVE('',#14761,#14762,#7952,.F.) ;
#18927=EDGE_CURVE('',#14762,#14763,#7953,.T.) ;
#18928=EDGE_CURVE('',#14763,#14764,#7954,.F.) ;
#18929=EDGE_CURVE('',#14764,#14761,#7955,.T.) ;
#18930=EDGE_CURVE('',#14765,#14766,#7956,.F.) ;
#18931=EDGE_CURVE('',#14766,#14767,#7957,.T.) ;
#18932=EDGE_CURVE('',#14767,#14768,#7958,.F.) ;
#18933=EDGE_CURVE('',#14768,#14765,#7959,.T.) ;
#18934=EDGE_CURVE('',#14736,#13804,#7960,.T.) ;
#18935=EDGE_CURVE('',#13805,#14711,#7961,.T.) ;
#18936=EDGE_CURVE('',#14738,#14716,#7962,.T.) ;
#18937=EDGE_CURVE('',#14769,#14737,#7963,.T.) ;
#18938=EDGE_CURVE('',#14678,#14769,#7964,.T.) ;
#18939=EDGE_CURVE('',#14770,#14679,#7965,.T.) ;
#18940=EDGE_CURVE('',#14740,#14770,#7966,.T.) ;
#18941=EDGE_CURVE('',#14718,#14739,#7967,.T.) ;
#18942=EDGE_CURVE('',#14742,#14719,#7968,.T.) ;
#18943=EDGE_CURVE('',#14771,#14741,#7969,.T.) ;
#18944=EDGE_CURVE('',#14682,#14771,#7970,.T.) ;
#18945=EDGE_CURVE('',#14772,#14683,#7971,.T.) ;
#18946=EDGE_CURVE('',#14744,#14772,#7972,.T.) ;
#18947=EDGE_CURVE('',#14720,#14743,#7973,.T.) ;
#18948=EDGE_CURVE('',#14746,#14721,#7974,.T.) ;
#18949=EDGE_CURVE('',#14773,#14745,#7975,.T.) ;
#18950=EDGE_CURVE('',#14686,#14773,#7976,.T.) ;
#18951=EDGE_CURVE('',#14774,#14687,#7977,.T.) ;
#18952=EDGE_CURVE('',#14748,#14774,#7978,.T.) ;
#18953=EDGE_CURVE('',#14722,#14747,#7979,.T.) ;
#18954=EDGE_CURVE('',#14750,#14723,#7980,.T.) ;
#18955=EDGE_CURVE('',#14775,#14749,#7981,.T.) ;
#18956=EDGE_CURVE('',#14690,#14775,#7982,.T.) ;
#18957=EDGE_CURVE('',#14776,#14691,#7983,.T.) ;
#18958=EDGE_CURVE('',#14752,#14776,#7984,.T.) ;
#18959=EDGE_CURVE('',#14724,#14751,#7985,.T.) ;
#18960=EDGE_CURVE('',#14754,#14725,#7986,.T.) ;
#18961=EDGE_CURVE('',#14777,#14753,#7987,.T.) ;
#18962=EDGE_CURVE('',#14694,#14777,#7988,.T.) ;
#18963=EDGE_CURVE('',#14778,#14695,#7989,.T.) ;
#18964=EDGE_CURVE('',#14756,#14778,#7990,.T.) ;
#18965=EDGE_CURVE('',#14726,#14755,#7991,.T.) ;
#18966=EDGE_CURVE('',#14758,#14727,#7992,.T.) ;
#18967=EDGE_CURVE('',#14779,#14757,#7993,.T.) ;
#18968=EDGE_CURVE('',#14698,#14779,#7994,.T.) ;
#18969=EDGE_CURVE('',#14780,#14699,#7995,.T.) ;
#18970=EDGE_CURVE('',#14760,#14780,#7996,.T.) ;
#18971=EDGE_CURVE('',#14728,#14759,#7997,.T.) ;
#18972=EDGE_CURVE('',#14762,#14729,#7998,.T.) ;
#18973=EDGE_CURVE('',#14781,#14761,#7999,.T.) ;
#18974=EDGE_CURVE('',#14702,#14781,#8000,.T.) ;
#18975=EDGE_CURVE('',#14782,#14703,#8001,.T.) ;
#18976=EDGE_CURVE('',#14764,#14782,#8002,.T.) ;
#18977=EDGE_CURVE('',#14730,#14763,#8003,.T.) ;
#18978=EDGE_CURVE('',#14766,#14731,#8004,.T.) ;
#18979=EDGE_CURVE('',#14783,#14765,#8005,.T.) ;
#18980=EDGE_CURVE('',#14706,#14783,#8006,.T.) ;
#18981=EDGE_CURVE('',#14784,#14707,#8007,.T.) ;
#18982=EDGE_CURVE('',#14768,#14784,#8008,.T.) ;
#18983=EDGE_CURVE('',#14732,#14767,#8009,.T.) ;
#18984=EDGE_CURVE('',#14710,#13766,#8010,.T.) ;
#18985=EDGE_CURVE('',#14769,#14770,#8011,.T.) ;
#18986=EDGE_CURVE('',#14771,#14772,#8012,.T.) ;
#18987=EDGE_CURVE('',#14773,#14774,#8013,.T.) ;
#18988=EDGE_CURVE('',#14775,#14776,#8014,.T.) ;
#18989=EDGE_CURVE('',#14777,#14778,#8015,.T.) ;
#18990=EDGE_CURVE('',#14779,#14780,#8016,.T.) ;
#18991=EDGE_CURVE('',#14781,#14782,#8017,.T.) ;
#18992=EDGE_CURVE('',#14783,#14784,#8018,.T.) ;
#18993=EDGE_CURVE('',#14785,#14785,#12142,.T.) ;
#18994=EDGE_CURVE('',#14786,#14787,#12143,.T.) ;
#18995=EDGE_CURVE('',#14787,#14786,#12144,.T.) ;
#18996=EDGE_CURVE('',#14787,#14785,#12145,.T.) ;
#18997=EDGE_CURVE('',#14788,#14788,#12146,.T.) ;
#18998=EDGE_CURVE('',#14788,#14786,#8019,.T.) ;
#18999=EDGE_CURVE('',#14788,#13941,#12147,.T.) ;
#19000=EDGE_CURVE('',#14658,#14298,#8020,.T.) ;
#19001=EDGE_CURVE('',#14789,#14789,#12148,.T.) ;
#19002=EDGE_CURVE('',#14790,#14791,#12149,.T.) ;
#19003=EDGE_CURVE('',#14791,#14790,#12150,.T.) ;
#19004=EDGE_CURVE('',#14791,#14789,#12151,.T.) ;
#19005=EDGE_CURVE('',#14792,#14792,#12152,.T.) ;
#19006=EDGE_CURVE('',#14792,#14790,#8021,.T.) ;
#19007=EDGE_CURVE('',#14792,#13942,#12153,.T.) ;
#19008=EDGE_CURVE('',#14641,#14321,#8022,.T.) ;
#19009=EDGE_CURVE('',#14793,#14793,#12154,.T.) ;
#19010=EDGE_CURVE('',#14794,#14795,#12155,.T.) ;
#19011=EDGE_CURVE('',#14795,#14794,#12156,.T.) ;
#19012=EDGE_CURVE('',#14795,#14793,#12157,.T.) ;
#19013=EDGE_CURVE('',#14796,#14796,#12158,.T.) ;
#19014=EDGE_CURVE('',#14796,#14794,#8023,.T.) ;
#19015=EDGE_CURVE('',#14796,#13943,#12159,.T.) ;
#19016=EDGE_CURVE('',#14624,#14344,#8024,.T.) ;
#19017=EDGE_CURVE('',#14797,#14797,#12160,.T.) ;
#19018=EDGE_CURVE('',#14798,#14799,#12161,.T.) ;
#19019=EDGE_CURVE('',#14799,#14798,#12162,.T.) ;
#19020=EDGE_CURVE('',#14799,#14797,#12163,.T.) ;
#19021=EDGE_CURVE('',#14800,#14800,#12164,.T.) ;
#19022=EDGE_CURVE('',#14800,#14798,#8025,.T.) ;
#19023=EDGE_CURVE('',#14800,#13944,#12165,.T.) ;
#19024=EDGE_CURVE('',#14607,#14367,#8026,.T.) ;
#19025=EDGE_CURVE('',#14801,#14801,#12166,.T.) ;
#19026=EDGE_CURVE('',#14802,#14803,#12167,.T.) ;
#19027=EDGE_CURVE('',#14803,#14802,#12168,.T.) ;
#19028=EDGE_CURVE('',#14803,#14801,#12169,.T.) ;
#19029=EDGE_CURVE('',#14804,#14804,#12170,.T.) ;
#19030=EDGE_CURVE('',#14804,#14802,#8027,.T.) ;
#19031=EDGE_CURVE('',#14804,#13945,#12171,.T.) ;
#19032=EDGE_CURVE('',#14590,#14390,#8028,.T.) ;
#19033=EDGE_CURVE('',#14805,#14805,#12172,.T.) ;
#19034=EDGE_CURVE('',#14806,#14807,#12173,.T.) ;
#19035=EDGE_CURVE('',#14807,#14806,#12174,.T.) ;
#19036=EDGE_CURVE('',#14807,#14805,#12175,.T.) ;
#19037=EDGE_CURVE('',#14808,#14808,#12176,.T.) ;
#19038=EDGE_CURVE('',#14808,#14806,#8029,.T.) ;
#19039=EDGE_CURVE('',#14808,#13946,#12177,.T.) ;
#19040=EDGE_CURVE('',#14573,#14413,#8030,.T.) ;
#19041=EDGE_CURVE('',#14809,#14809,#12178,.T.) ;
#19042=EDGE_CURVE('',#14810,#14811,#12179,.T.) ;
#19043=EDGE_CURVE('',#14811,#14810,#12180,.T.) ;
#19044=EDGE_CURVE('',#14811,#14809,#12181,.T.) ;
#19045=EDGE_CURVE('',#14812,#14812,#12182,.T.) ;
#19046=EDGE_CURVE('',#14812,#14810,#8031,.T.) ;
#19047=EDGE_CURVE('',#14812,#13947,#12183,.T.) ;
#19048=EDGE_CURVE('',#14556,#14436,#8032,.T.) ;
#19049=EDGE_CURVE('',#14813,#14813,#12184,.T.) ;
#19050=EDGE_CURVE('',#14814,#14815,#12185,.T.) ;
#19051=EDGE_CURVE('',#14815,#14814,#12186,.T.) ;
#19052=EDGE_CURVE('',#14815,#14813,#12187,.T.) ;
#19053=EDGE_CURVE('',#14816,#14816,#12188,.T.) ;
#19054=EDGE_CURVE('',#14816,#14814,#8033,.T.) ;
#19055=EDGE_CURVE('',#14816,#13948,#12189,.T.) ;
#19056=EDGE_CURVE('',#14539,#14459,#8034,.T.) ;
#19057=EDGE_CURVE('',#14817,#14818,#12190,.T.) ;
#19058=EDGE_CURVE('',#14818,#14817,#12191,.T.) ;
#19059=EDGE_CURVE('',#14818,#14505,#12192,.T.) ;
#19060=EDGE_CURVE('',#14819,#14819,#12193,.T.) ;
#19061=EDGE_CURVE('',#14819,#14817,#8035,.T.) ;
#19062=EDGE_CURVE('',#14819,#14525,#12194,.T.) ;
#19063=EDGE_CURVE('',#13767,#14733,#8036,.T.) ;
#19064=EDGE_CURVE('',#14674,#14134,#8037,.T.) ;
#19065=EDGE_CURVE('',#14132,#14673,#8038,.T.) ;
#19066=EDGE_CURVE('',#14672,#14130,#8039,.T.) ;
#19067=EDGE_CURVE('',#14657,#14155,#8040,.T.) ;
#19068=EDGE_CURVE('',#14153,#14656,#8041,.T.) ;
#19069=EDGE_CURVE('',#14655,#14151,#8042,.T.) ;
#19070=EDGE_CURVE('',#14640,#14176,#8043,.T.) ;
#19071=EDGE_CURVE('',#14174,#14639,#8044,.T.) ;
#19072=EDGE_CURVE('',#14638,#14172,#8045,.T.) ;
#19073=EDGE_CURVE('',#14623,#14197,#8046,.T.) ;
#19074=EDGE_CURVE('',#14195,#14622,#8047,.T.) ;
#19075=EDGE_CURVE('',#14621,#14193,#8048,.T.) ;
#19076=EDGE_CURVE('',#14606,#14218,#8049,.T.) ;
#19077=EDGE_CURVE('',#14216,#14605,#8050,.T.) ;
#19078=EDGE_CURVE('',#14604,#14214,#8051,.T.) ;
#19079=EDGE_CURVE('',#14589,#14239,#8052,.T.) ;
#19080=EDGE_CURVE('',#14237,#14588,#8053,.T.) ;
#19081=EDGE_CURVE('',#14587,#14235,#8054,.T.) ;
#19082=EDGE_CURVE('',#14572,#14260,#8055,.T.) ;
#19083=EDGE_CURVE('',#14258,#14571,#8056,.T.) ;
#19084=EDGE_CURVE('',#14570,#14256,#8057,.T.) ;
#19085=EDGE_CURVE('',#14555,#14281,#8058,.T.) ;
#19086=EDGE_CURVE('',#14279,#14554,#8059,.T.) ;
#19087=EDGE_CURVE('',#14553,#14277,#8060,.T.) ;
#23464=ORIENTED_EDGE('',*,*,#17138,.F.) ;
#23465=ORIENTED_EDGE('',*,*,#17139,.T.) ;
#23466=ORIENTED_EDGE('',*,*,#17140,.T.) ;
#23467=ORIENTED_EDGE('',*,*,#17141,.F.) ;
#23468=ORIENTED_EDGE('',*,*,#17142,.F.) ;
#23469=ORIENTED_EDGE('',*,*,#17143,.F.) ;
#23470=ORIENTED_EDGE('',*,*,#17144,.T.) ;
#23471=ORIENTED_EDGE('',*,*,#17139,.F.) ;
#23472=ORIENTED_EDGE('',*,*,#17145,.F.) ;
#23473=ORIENTED_EDGE('',*,*,#17141,.T.) ;
#23474=ORIENTED_EDGE('',*,*,#17146,.T.) ;
#23475=ORIENTED_EDGE('',*,*,#17147,.F.) ;
#23476=ORIENTED_EDGE('',*,*,#17146,.F.) ;
#23477=ORIENTED_EDGE('',*,*,#17140,.F.) ;
#23478=ORIENTED_EDGE('',*,*,#17144,.F.) ;
#23479=ORIENTED_EDGE('',*,*,#17148,.F.) ;
#23480=ORIENTED_EDGE('',*,*,#17149,.F.) ;
#23481=ORIENTED_EDGE('',*,*,#17150,.T.) ;
#23482=ORIENTED_EDGE('',*,*,#17151,.T.) ;
#23483=ORIENTED_EDGE('',*,*,#17152,.F.) ;
#23484=ORIENTED_EDGE('',*,*,#17153,.F.) ;
#23485=ORIENTED_EDGE('',*,*,#17154,.F.) ;
#23486=ORIENTED_EDGE('',*,*,#17155,.T.) ;
#23487=ORIENTED_EDGE('',*,*,#17150,.F.) ;
#23488=ORIENTED_EDGE('',*,*,#17156,.F.) ;
#23489=ORIENTED_EDGE('',*,*,#17152,.T.) ;
#23490=ORIENTED_EDGE('',*,*,#17157,.T.) ;
#23491=ORIENTED_EDGE('',*,*,#17158,.F.) ;
#23492=ORIENTED_EDGE('',*,*,#17157,.F.) ;
#23493=ORIENTED_EDGE('',*,*,#17151,.F.) ;
#23494=ORIENTED_EDGE('',*,*,#17155,.F.) ;
#23495=ORIENTED_EDGE('',*,*,#17159,.F.) ;
#23496=ORIENTED_EDGE('',*,*,#17160,.F.) ;
#23497=ORIENTED_EDGE('',*,*,#17161,.T.) ;
#23498=ORIENTED_EDGE('',*,*,#17162,.T.) ;
#23499=ORIENTED_EDGE('',*,*,#17163,.F.) ;
#23500=ORIENTED_EDGE('',*,*,#17164,.F.) ;
#23501=ORIENTED_EDGE('',*,*,#17165,.T.) ;
#23502=ORIENTED_EDGE('',*,*,#17166,.T.) ;
#23503=ORIENTED_EDGE('',*,*,#17161,.F.) ;
#23504=ORIENTED_EDGE('',*,*,#17167,.F.) ;
#23505=ORIENTED_EDGE('',*,*,#17168,.F.) ;
#23506=ORIENTED_EDGE('',*,*,#17169,.T.) ;
#23507=ORIENTED_EDGE('',*,*,#17165,.F.) ;
#23508=ORIENTED_EDGE('',*,*,#17169,.F.) ;
#23509=ORIENTED_EDGE('',*,*,#17170,.F.) ;
#23510=ORIENTED_EDGE('',*,*,#17162,.F.) ;
#23511=ORIENTED_EDGE('',*,*,#17166,.F.) ;
#23512=ORIENTED_EDGE('',*,*,#17171,.F.) ;
#23513=ORIENTED_EDGE('',*,*,#17172,.T.) ;
#23514=ORIENTED_EDGE('',*,*,#17173,.T.) ;
#23515=ORIENTED_EDGE('',*,*,#17174,.F.) ;
#23516=ORIENTED_EDGE('',*,*,#17175,.F.) ;
#23517=ORIENTED_EDGE('',*,*,#17176,.F.) ;
#23518=ORIENTED_EDGE('',*,*,#17177,.T.) ;
#23519=ORIENTED_EDGE('',*,*,#17172,.F.) ;
#23520=ORIENTED_EDGE('',*,*,#17178,.F.) ;
#23521=ORIENTED_EDGE('',*,*,#17174,.T.) ;
#23522=ORIENTED_EDGE('',*,*,#17179,.T.) ;
#23523=ORIENTED_EDGE('',*,*,#17180,.F.) ;
#23524=ORIENTED_EDGE('',*,*,#17179,.F.) ;
#23525=ORIENTED_EDGE('',*,*,#17173,.F.) ;
#23526=ORIENTED_EDGE('',*,*,#17177,.F.) ;
#23527=ORIENTED_EDGE('',*,*,#17181,.F.) ;
#23528=ORIENTED_EDGE('',*,*,#17182,.F.) ;
#23529=ORIENTED_EDGE('',*,*,#17183,.T.) ;
#23530=ORIENTED_EDGE('',*,*,#17184,.T.) ;
#23531=ORIENTED_EDGE('',*,*,#17185,.F.) ;
#23532=ORIENTED_EDGE('',*,*,#17186,.F.) ;
#23533=ORIENTED_EDGE('',*,*,#17187,.F.) ;
#23534=ORIENTED_EDGE('',*,*,#17188,.T.) ;
#23535=ORIENTED_EDGE('',*,*,#17183,.F.) ;
#23536=ORIENTED_EDGE('',*,*,#17189,.F.) ;
#23537=ORIENTED_EDGE('',*,*,#17185,.T.) ;
#23538=ORIENTED_EDGE('',*,*,#17190,.T.) ;
#23539=ORIENTED_EDGE('',*,*,#17191,.F.) ;
#23540=ORIENTED_EDGE('',*,*,#17190,.F.) ;
#23541=ORIENTED_EDGE('',*,*,#17184,.F.) ;
#23542=ORIENTED_EDGE('',*,*,#17188,.F.) ;
#23543=ORIENTED_EDGE('',*,*,#17192,.F.) ;
#23544=ORIENTED_EDGE('',*,*,#17193,.F.) ;
#23545=ORIENTED_EDGE('',*,*,#17194,.T.) ;
#23546=ORIENTED_EDGE('',*,*,#17195,.T.) ;
#23547=ORIENTED_EDGE('',*,*,#17196,.F.) ;
#23548=ORIENTED_EDGE('',*,*,#17197,.F.) ;
#23549=ORIENTED_EDGE('',*,*,#17198,.F.) ;
#23550=ORIENTED_EDGE('',*,*,#17199,.T.) ;
#23551=ORIENTED_EDGE('',*,*,#17194,.F.) ;
#23552=ORIENTED_EDGE('',*,*,#17200,.F.) ;
#23553=ORIENTED_EDGE('',*,*,#17196,.T.) ;
#23554=ORIENTED_EDGE('',*,*,#17201,.T.) ;
#23555=ORIENTED_EDGE('',*,*,#17202,.F.) ;
#23556=ORIENTED_EDGE('',*,*,#17201,.F.) ;
#23557=ORIENTED_EDGE('',*,*,#17195,.F.) ;
#23558=ORIENTED_EDGE('',*,*,#17199,.F.) ;
#23559=ORIENTED_EDGE('',*,*,#17203,.F.) ;
#23560=ORIENTED_EDGE('',*,*,#17204,.F.) ;
#23561=ORIENTED_EDGE('',*,*,#17205,.T.) ;
#23562=ORIENTED_EDGE('',*,*,#17206,.T.) ;
#23563=ORIENTED_EDGE('',*,*,#17207,.F.) ;
#23564=ORIENTED_EDGE('',*,*,#17208,.F.) ;
#23565=ORIENTED_EDGE('',*,*,#17209,.T.) ;
#23566=ORIENTED_EDGE('',*,*,#17210,.T.) ;
#23567=ORIENTED_EDGE('',*,*,#17205,.F.) ;
#23568=ORIENTED_EDGE('',*,*,#17211,.F.) ;
#23569=ORIENTED_EDGE('',*,*,#17212,.F.) ;
#23570=ORIENTED_EDGE('',*,*,#17213,.T.) ;
#23571=ORIENTED_EDGE('',*,*,#17209,.F.) ;
#23572=ORIENTED_EDGE('',*,*,#17213,.F.) ;
#23573=ORIENTED_EDGE('',*,*,#17214,.F.) ;
#23574=ORIENTED_EDGE('',*,*,#17206,.F.) ;
#23575=ORIENTED_EDGE('',*,*,#17210,.F.) ;
#23576=ORIENTED_EDGE('',*,*,#17215,.F.) ;
#23577=ORIENTED_EDGE('',*,*,#17216,.T.) ;
#23578=ORIENTED_EDGE('',*,*,#17217,.T.) ;
#23579=ORIENTED_EDGE('',*,*,#17218,.F.) ;
#23580=ORIENTED_EDGE('',*,*,#17219,.F.) ;
#23581=ORIENTED_EDGE('',*,*,#17220,.F.) ;
#23582=ORIENTED_EDGE('',*,*,#17221,.T.) ;
#23583=ORIENTED_EDGE('',*,*,#17216,.F.) ;
#23584=ORIENTED_EDGE('',*,*,#17222,.F.) ;
#23585=ORIENTED_EDGE('',*,*,#17218,.T.) ;
#23586=ORIENTED_EDGE('',*,*,#17223,.T.) ;
#23587=ORIENTED_EDGE('',*,*,#17224,.F.) ;
#23588=ORIENTED_EDGE('',*,*,#17223,.F.) ;
#23589=ORIENTED_EDGE('',*,*,#17217,.F.) ;
#23590=ORIENTED_EDGE('',*,*,#17221,.F.) ;
#23591=ORIENTED_EDGE('',*,*,#17225,.F.) ;
#23592=ORIENTED_EDGE('',*,*,#17226,.F.) ;
#23593=ORIENTED_EDGE('',*,*,#17227,.T.) ;
#23594=ORIENTED_EDGE('',*,*,#17228,.T.) ;
#23595=ORIENTED_EDGE('',*,*,#17229,.F.) ;
#23596=ORIENTED_EDGE('',*,*,#17230,.F.) ;
#23597=ORIENTED_EDGE('',*,*,#17231,.F.) ;
#23598=ORIENTED_EDGE('',*,*,#17232,.T.) ;
#23599=ORIENTED_EDGE('',*,*,#17227,.F.) ;
#23600=ORIENTED_EDGE('',*,*,#17233,.F.) ;
#23601=ORIENTED_EDGE('',*,*,#17229,.T.) ;
#23602=ORIENTED_EDGE('',*,*,#17234,.T.) ;
#23603=ORIENTED_EDGE('',*,*,#17235,.F.) ;
#23604=ORIENTED_EDGE('',*,*,#17234,.F.) ;
#23605=ORIENTED_EDGE('',*,*,#17228,.F.) ;
#23606=ORIENTED_EDGE('',*,*,#17232,.F.) ;
#23607=ORIENTED_EDGE('',*,*,#17236,.F.) ;
#23608=ORIENTED_EDGE('',*,*,#17147,.T.) ;
#23609=ORIENTED_EDGE('',*,*,#17148,.T.) ;
#23610=ORIENTED_EDGE('',*,*,#17143,.T.) ;
#23611=ORIENTED_EDGE('',*,*,#17237,.F.) ;
#23612=ORIENTED_EDGE('',*,*,#17180,.T.) ;
#23613=ORIENTED_EDGE('',*,*,#17181,.T.) ;
#23614=ORIENTED_EDGE('',*,*,#17176,.T.) ;
#23615=ORIENTED_EDGE('',*,*,#17238,.F.) ;
#23616=ORIENTED_EDGE('',*,*,#17224,.T.) ;
#23617=ORIENTED_EDGE('',*,*,#17225,.T.) ;
#23618=ORIENTED_EDGE('',*,*,#17220,.T.) ;
#23619=ORIENTED_EDGE('',*,*,#17239,.F.) ;
#23620=ORIENTED_EDGE('',*,*,#17202,.T.) ;
#23621=ORIENTED_EDGE('',*,*,#17203,.T.) ;
#23622=ORIENTED_EDGE('',*,*,#17198,.T.) ;
#23623=ORIENTED_EDGE('',*,*,#17240,.F.) ;
#23624=ORIENTED_EDGE('',*,*,#17158,.T.) ;
#23625=ORIENTED_EDGE('',*,*,#17159,.T.) ;
#23626=ORIENTED_EDGE('',*,*,#17154,.T.) ;
#23627=ORIENTED_EDGE('',*,*,#17241,.F.) ;
#23628=ORIENTED_EDGE('',*,*,#17163,.T.) ;
#23629=ORIENTED_EDGE('',*,*,#17170,.T.) ;
#23630=ORIENTED_EDGE('',*,*,#17168,.T.) ;
#23631=ORIENTED_EDGE('',*,*,#17242,.F.) ;
#23632=ORIENTED_EDGE('',*,*,#17207,.T.) ;
#23633=ORIENTED_EDGE('',*,*,#17214,.T.) ;
#23634=ORIENTED_EDGE('',*,*,#17212,.T.) ;
#23635=ORIENTED_EDGE('',*,*,#17243,.F.) ;
#23636=ORIENTED_EDGE('',*,*,#17244,.F.) ;
#23637=ORIENTED_EDGE('',*,*,#17245,.T.) ;
#23638=ORIENTED_EDGE('',*,*,#17246,.T.) ;
#23639=ORIENTED_EDGE('',*,*,#17247,.T.) ;
#23640=ORIENTED_EDGE('',*,*,#17248,.T.) ;
#23641=ORIENTED_EDGE('',*,*,#17249,.T.) ;
#23642=ORIENTED_EDGE('',*,*,#17250,.T.) ;
#23643=ORIENTED_EDGE('',*,*,#17251,.T.) ;
#23644=ORIENTED_EDGE('',*,*,#17252,.T.) ;
#23645=ORIENTED_EDGE('',*,*,#17253,.T.) ;
#23646=ORIENTED_EDGE('',*,*,#17254,.T.) ;
#23647=ORIENTED_EDGE('',*,*,#17255,.T.) ;
#23648=ORIENTED_EDGE('',*,*,#17256,.T.) ;
#23649=ORIENTED_EDGE('',*,*,#17257,.T.) ;
#23650=ORIENTED_EDGE('',*,*,#17258,.T.) ;
#23651=ORIENTED_EDGE('',*,*,#17259,.T.) ;
#23652=ORIENTED_EDGE('',*,*,#17260,.T.) ;
#23653=ORIENTED_EDGE('',*,*,#17261,.T.) ;
#23654=ORIENTED_EDGE('',*,*,#17262,.T.) ;
#23655=ORIENTED_EDGE('',*,*,#17263,.T.) ;
#23656=ORIENTED_EDGE('',*,*,#17264,.T.) ;
#23657=ORIENTED_EDGE('',*,*,#17265,.T.) ;
#23658=ORIENTED_EDGE('',*,*,#17266,.T.) ;
#23659=ORIENTED_EDGE('',*,*,#17267,.T.) ;
#23660=ORIENTED_EDGE('',*,*,#17268,.T.) ;
#23661=ORIENTED_EDGE('',*,*,#17269,.T.) ;
#23662=ORIENTED_EDGE('',*,*,#17270,.T.) ;
#23663=ORIENTED_EDGE('',*,*,#17271,.T.) ;
#23664=ORIENTED_EDGE('',*,*,#17272,.T.) ;
#23665=ORIENTED_EDGE('',*,*,#17273,.T.) ;
#23666=ORIENTED_EDGE('',*,*,#17274,.T.) ;
#23667=ORIENTED_EDGE('',*,*,#17275,.T.) ;
#23668=ORIENTED_EDGE('',*,*,#17276,.T.) ;
#23669=ORIENTED_EDGE('',*,*,#17277,.T.) ;
#23670=ORIENTED_EDGE('',*,*,#17278,.T.) ;
#23671=ORIENTED_EDGE('',*,*,#17279,.T.) ;
#23672=ORIENTED_EDGE('',*,*,#17280,.T.) ;
#23673=ORIENTED_EDGE('',*,*,#17281,.T.) ;
#23674=ORIENTED_EDGE('',*,*,#17282,.T.) ;
#23675=ORIENTED_EDGE('',*,*,#17283,.F.) ;
#23676=ORIENTED_EDGE('',*,*,#17235,.T.) ;
#23677=ORIENTED_EDGE('',*,*,#17236,.T.) ;
#23678=ORIENTED_EDGE('',*,*,#17231,.T.) ;
#23679=ORIENTED_EDGE('',*,*,#17284,.F.) ;
#23680=ORIENTED_EDGE('',*,*,#17191,.T.) ;
#23681=ORIENTED_EDGE('',*,*,#17192,.T.) ;
#23682=ORIENTED_EDGE('',*,*,#17187,.T.) ;
#23683=ORIENTED_EDGE('',*,*,#17285,.F.) ;
#23684=ORIENTED_EDGE('',*,*,#17286,.T.) ;
#23685=ORIENTED_EDGE('',*,*,#17287,.T.) ;
#23686=ORIENTED_EDGE('',*,*,#17288,.T.) ;
#23687=ORIENTED_EDGE('',*,*,#17287,.F.) ;
#23688=ORIENTED_EDGE('',*,*,#17289,.T.) ;
#23689=ORIENTED_EDGE('',*,*,#17290,.T.) ;
#23690=ORIENTED_EDGE('',*,*,#17286,.F.) ;
#23691=ORIENTED_EDGE('',*,*,#17290,.F.) ;
#23692=ORIENTED_EDGE('',*,*,#17291,.F.) ;
#23693=ORIENTED_EDGE('',*,*,#17292,.F.) ;
#23694=ORIENTED_EDGE('',*,*,#17293,.F.) ;
#23695=ORIENTED_EDGE('',*,*,#17294,.F.) ;
#23696=ORIENTED_EDGE('',*,*,#17295,.T.) ;
#23697=ORIENTED_EDGE('',*,*,#17296,.F.) ;
#23698=ORIENTED_EDGE('',*,*,#17297,.T.) ;
#23699=ORIENTED_EDGE('',*,*,#17298,.F.) ;
#23700=ORIENTED_EDGE('',*,*,#17299,.T.) ;
#23701=ORIENTED_EDGE('',*,*,#17300,.F.) ;
#23702=ORIENTED_EDGE('',*,*,#17301,.T.) ;
#23703=ORIENTED_EDGE('',*,*,#17302,.F.) ;
#23704=ORIENTED_EDGE('',*,*,#17288,.F.) ;
#23705=ORIENTED_EDGE('',*,*,#17303,.T.) ;
#23706=ORIENTED_EDGE('',*,*,#17304,.T.) ;
#23707=ORIENTED_EDGE('',*,*,#17305,.T.) ;
#23708=ORIENTED_EDGE('',*,*,#17304,.F.) ;
#23709=ORIENTED_EDGE('',*,*,#17306,.T.) ;
#23710=ORIENTED_EDGE('',*,*,#17307,.T.) ;
#23711=ORIENTED_EDGE('',*,*,#17303,.F.) ;
#23712=ORIENTED_EDGE('',*,*,#17307,.F.) ;
#23713=ORIENTED_EDGE('',*,*,#17308,.F.) ;
#23714=ORIENTED_EDGE('',*,*,#17309,.F.) ;
#23715=ORIENTED_EDGE('',*,*,#17310,.F.) ;
#23716=ORIENTED_EDGE('',*,*,#17311,.F.) ;
#23717=ORIENTED_EDGE('',*,*,#17312,.T.) ;
#23718=ORIENTED_EDGE('',*,*,#17313,.F.) ;
#23719=ORIENTED_EDGE('',*,*,#17314,.T.) ;
#23720=ORIENTED_EDGE('',*,*,#17315,.F.) ;
#23721=ORIENTED_EDGE('',*,*,#17316,.T.) ;
#23722=ORIENTED_EDGE('',*,*,#17317,.F.) ;
#23723=ORIENTED_EDGE('',*,*,#17318,.T.) ;
#23724=ORIENTED_EDGE('',*,*,#17319,.F.) ;
#23725=ORIENTED_EDGE('',*,*,#17305,.F.) ;
#23726=ORIENTED_EDGE('',*,*,#17320,.T.) ;
#23727=ORIENTED_EDGE('',*,*,#17321,.T.) ;
#23728=ORIENTED_EDGE('',*,*,#17322,.T.) ;
#23729=ORIENTED_EDGE('',*,*,#17321,.F.) ;
#23730=ORIENTED_EDGE('',*,*,#17323,.T.) ;
#23731=ORIENTED_EDGE('',*,*,#17324,.T.) ;
#23732=ORIENTED_EDGE('',*,*,#17320,.F.) ;
#23733=ORIENTED_EDGE('',*,*,#17324,.F.) ;
#23734=ORIENTED_EDGE('',*,*,#17325,.F.) ;
#23735=ORIENTED_EDGE('',*,*,#17326,.F.) ;
#23736=ORIENTED_EDGE('',*,*,#17327,.F.) ;
#23737=ORIENTED_EDGE('',*,*,#17328,.F.) ;
#23738=ORIENTED_EDGE('',*,*,#17329,.T.) ;
#23739=ORIENTED_EDGE('',*,*,#17330,.F.) ;
#23740=ORIENTED_EDGE('',*,*,#17331,.T.) ;
#23741=ORIENTED_EDGE('',*,*,#17332,.F.) ;
#23742=ORIENTED_EDGE('',*,*,#17333,.T.) ;
#23743=ORIENTED_EDGE('',*,*,#17334,.F.) ;
#23744=ORIENTED_EDGE('',*,*,#17335,.T.) ;
#23745=ORIENTED_EDGE('',*,*,#17336,.F.) ;
#23746=ORIENTED_EDGE('',*,*,#17322,.F.) ;
#23747=ORIENTED_EDGE('',*,*,#17337,.T.) ;
#23748=ORIENTED_EDGE('',*,*,#17338,.T.) ;
#23749=ORIENTED_EDGE('',*,*,#17339,.T.) ;
#23750=ORIENTED_EDGE('',*,*,#17338,.F.) ;
#23751=ORIENTED_EDGE('',*,*,#17340,.T.) ;
#23752=ORIENTED_EDGE('',*,*,#17341,.T.) ;
#23753=ORIENTED_EDGE('',*,*,#17337,.F.) ;
#23754=ORIENTED_EDGE('',*,*,#17341,.F.) ;
#23755=ORIENTED_EDGE('',*,*,#17342,.F.) ;
#23756=ORIENTED_EDGE('',*,*,#17343,.F.) ;
#23757=ORIENTED_EDGE('',*,*,#17344,.F.) ;
#23758=ORIENTED_EDGE('',*,*,#17345,.F.) ;
#23759=ORIENTED_EDGE('',*,*,#17346,.T.) ;
#23760=ORIENTED_EDGE('',*,*,#17347,.F.) ;
#23761=ORIENTED_EDGE('',*,*,#17348,.T.) ;
#23762=ORIENTED_EDGE('',*,*,#17349,.F.) ;
#23763=ORIENTED_EDGE('',*,*,#17350,.T.) ;
#23764=ORIENTED_EDGE('',*,*,#17351,.F.) ;
#23765=ORIENTED_EDGE('',*,*,#17352,.T.) ;
#23766=ORIENTED_EDGE('',*,*,#17353,.F.) ;
#23767=ORIENTED_EDGE('',*,*,#17339,.F.) ;
#23768=ORIENTED_EDGE('',*,*,#17354,.T.) ;
#23769=ORIENTED_EDGE('',*,*,#17355,.T.) ;
#23770=ORIENTED_EDGE('',*,*,#17356,.T.) ;
#23771=ORIENTED_EDGE('',*,*,#17355,.F.) ;
#23772=ORIENTED_EDGE('',*,*,#17357,.T.) ;
#23773=ORIENTED_EDGE('',*,*,#17358,.T.) ;
#23774=ORIENTED_EDGE('',*,*,#17354,.F.) ;
#23775=ORIENTED_EDGE('',*,*,#17358,.F.) ;
#23776=ORIENTED_EDGE('',*,*,#17359,.F.) ;
#23777=ORIENTED_EDGE('',*,*,#17360,.F.) ;
#23778=ORIENTED_EDGE('',*,*,#17361,.F.) ;
#23779=ORIENTED_EDGE('',*,*,#17362,.F.) ;
#23780=ORIENTED_EDGE('',*,*,#17363,.T.) ;
#23781=ORIENTED_EDGE('',*,*,#17364,.F.) ;
#23782=ORIENTED_EDGE('',*,*,#17365,.T.) ;
#23783=ORIENTED_EDGE('',*,*,#17366,.F.) ;
#23784=ORIENTED_EDGE('',*,*,#17367,.T.) ;
#23785=ORIENTED_EDGE('',*,*,#17368,.F.) ;
#23786=ORIENTED_EDGE('',*,*,#17369,.T.) ;
#23787=ORIENTED_EDGE('',*,*,#17370,.F.) ;
#23788=ORIENTED_EDGE('',*,*,#17356,.F.) ;
#23789=ORIENTED_EDGE('',*,*,#17371,.T.) ;
#23790=ORIENTED_EDGE('',*,*,#17372,.T.) ;
#23791=ORIENTED_EDGE('',*,*,#17373,.T.) ;
#23792=ORIENTED_EDGE('',*,*,#17372,.F.) ;
#23793=ORIENTED_EDGE('',*,*,#17374,.T.) ;
#23794=ORIENTED_EDGE('',*,*,#17375,.T.) ;
#23795=ORIENTED_EDGE('',*,*,#17371,.F.) ;
#23796=ORIENTED_EDGE('',*,*,#17375,.F.) ;
#23797=ORIENTED_EDGE('',*,*,#17376,.F.) ;
#23798=ORIENTED_EDGE('',*,*,#17377,.F.) ;
#23799=ORIENTED_EDGE('',*,*,#17378,.F.) ;
#23800=ORIENTED_EDGE('',*,*,#17379,.F.) ;
#23801=ORIENTED_EDGE('',*,*,#17380,.T.) ;
#23802=ORIENTED_EDGE('',*,*,#17381,.F.) ;
#23803=ORIENTED_EDGE('',*,*,#17382,.T.) ;
#23804=ORIENTED_EDGE('',*,*,#17383,.F.) ;
#23805=ORIENTED_EDGE('',*,*,#17384,.T.) ;
#23806=ORIENTED_EDGE('',*,*,#17385,.F.) ;
#23807=ORIENTED_EDGE('',*,*,#17386,.T.) ;
#23808=ORIENTED_EDGE('',*,*,#17387,.F.) ;
#23809=ORIENTED_EDGE('',*,*,#17373,.F.) ;
#23810=ORIENTED_EDGE('',*,*,#17388,.T.) ;
#23811=ORIENTED_EDGE('',*,*,#17389,.T.) ;
#23812=ORIENTED_EDGE('',*,*,#17390,.T.) ;
#23813=ORIENTED_EDGE('',*,*,#17389,.F.) ;
#23814=ORIENTED_EDGE('',*,*,#17391,.T.) ;
#23815=ORIENTED_EDGE('',*,*,#17392,.T.) ;
#23816=ORIENTED_EDGE('',*,*,#17388,.F.) ;
#23817=ORIENTED_EDGE('',*,*,#17392,.F.) ;
#23818=ORIENTED_EDGE('',*,*,#17393,.F.) ;
#23819=ORIENTED_EDGE('',*,*,#17394,.F.) ;
#23820=ORIENTED_EDGE('',*,*,#17395,.F.) ;
#23821=ORIENTED_EDGE('',*,*,#17396,.F.) ;
#23822=ORIENTED_EDGE('',*,*,#17397,.T.) ;
#23823=ORIENTED_EDGE('',*,*,#17398,.F.) ;
#23824=ORIENTED_EDGE('',*,*,#17399,.T.) ;
#23825=ORIENTED_EDGE('',*,*,#17400,.F.) ;
#23826=ORIENTED_EDGE('',*,*,#17401,.T.) ;
#23827=ORIENTED_EDGE('',*,*,#17402,.F.) ;
#23828=ORIENTED_EDGE('',*,*,#17403,.T.) ;
#23829=ORIENTED_EDGE('',*,*,#17404,.F.) ;
#23830=ORIENTED_EDGE('',*,*,#17390,.F.) ;
#23831=ORIENTED_EDGE('',*,*,#17405,.T.) ;
#23832=ORIENTED_EDGE('',*,*,#17406,.T.) ;
#23833=ORIENTED_EDGE('',*,*,#17407,.T.) ;
#23834=ORIENTED_EDGE('',*,*,#17406,.F.) ;
#23835=ORIENTED_EDGE('',*,*,#17408,.T.) ;
#23836=ORIENTED_EDGE('',*,*,#17409,.T.) ;
#23837=ORIENTED_EDGE('',*,*,#17405,.F.) ;
#23838=ORIENTED_EDGE('',*,*,#17409,.F.) ;
#23839=ORIENTED_EDGE('',*,*,#17410,.F.) ;
#23840=ORIENTED_EDGE('',*,*,#17411,.F.) ;
#23841=ORIENTED_EDGE('',*,*,#17412,.F.) ;
#23842=ORIENTED_EDGE('',*,*,#17413,.F.) ;
#23843=ORIENTED_EDGE('',*,*,#17414,.T.) ;
#23844=ORIENTED_EDGE('',*,*,#17415,.F.) ;
#23845=ORIENTED_EDGE('',*,*,#17416,.T.) ;
#23846=ORIENTED_EDGE('',*,*,#17417,.F.) ;
#23847=ORIENTED_EDGE('',*,*,#17418,.T.) ;
#23848=ORIENTED_EDGE('',*,*,#17419,.F.) ;
#23849=ORIENTED_EDGE('',*,*,#17420,.T.) ;
#23850=ORIENTED_EDGE('',*,*,#17421,.F.) ;
#23851=ORIENTED_EDGE('',*,*,#17407,.F.) ;
#23852=ORIENTED_EDGE('',*,*,#17422,.T.) ;
#23853=ORIENTED_EDGE('',*,*,#17423,.T.) ;
#23854=ORIENTED_EDGE('',*,*,#17424,.T.) ;
#23855=ORIENTED_EDGE('',*,*,#17423,.F.) ;
#23856=ORIENTED_EDGE('',*,*,#17425,.F.) ;
#23857=ORIENTED_EDGE('',*,*,#17426,.F.) ;
#23858=ORIENTED_EDGE('',*,*,#17427,.F.) ;
#23859=ORIENTED_EDGE('',*,*,#17428,.F.) ;
#23860=ORIENTED_EDGE('',*,*,#17429,.F.) ;
#23861=ORIENTED_EDGE('',*,*,#17430,.F.) ;
#23862=ORIENTED_EDGE('',*,*,#17431,.F.) ;
#23863=ORIENTED_EDGE('',*,*,#17432,.F.) ;
#23864=ORIENTED_EDGE('',*,*,#17433,.F.) ;
#23865=ORIENTED_EDGE('',*,*,#17434,.F.) ;
#23866=ORIENTED_EDGE('',*,*,#17435,.F.) ;
#23867=ORIENTED_EDGE('',*,*,#17436,.F.) ;
#23868=ORIENTED_EDGE('',*,*,#17424,.F.) ;
#23869=ORIENTED_EDGE('',*,*,#17437,.F.) ;
#23870=ORIENTED_EDGE('',*,*,#17438,.T.) ;
#23871=ORIENTED_EDGE('',*,*,#17422,.F.) ;
#23872=ORIENTED_EDGE('',*,*,#17438,.F.) ;
#23873=ORIENTED_EDGE('',*,*,#17439,.T.) ;
#23874=ORIENTED_EDGE('',*,*,#17289,.F.) ;
#23875=ORIENTED_EDGE('',*,*,#17440,.T.) ;
#23876=ORIENTED_EDGE('',*,*,#17306,.F.) ;
#23877=ORIENTED_EDGE('',*,*,#17441,.T.) ;
#23878=ORIENTED_EDGE('',*,*,#17323,.F.) ;
#23879=ORIENTED_EDGE('',*,*,#17442,.T.) ;
#23880=ORIENTED_EDGE('',*,*,#17340,.F.) ;
#23881=ORIENTED_EDGE('',*,*,#17443,.T.) ;
#23882=ORIENTED_EDGE('',*,*,#17357,.F.) ;
#23883=ORIENTED_EDGE('',*,*,#17444,.T.) ;
#23884=ORIENTED_EDGE('',*,*,#17374,.F.) ;
#23885=ORIENTED_EDGE('',*,*,#17445,.T.) ;
#23886=ORIENTED_EDGE('',*,*,#17391,.F.) ;
#23887=ORIENTED_EDGE('',*,*,#17446,.T.) ;
#23888=ORIENTED_EDGE('',*,*,#17408,.F.) ;
#23889=ORIENTED_EDGE('',*,*,#17447,.T.) ;
#23890=ORIENTED_EDGE('',*,*,#17448,.T.) ;
#23891=ORIENTED_EDGE('',*,*,#17449,.T.) ;
#23892=ORIENTED_EDGE('',*,*,#17295,.F.) ;
#23893=ORIENTED_EDGE('',*,*,#17450,.T.) ;
#23894=ORIENTED_EDGE('',*,*,#17296,.T.) ;
#23895=ORIENTED_EDGE('',*,*,#17449,.F.) ;
#23896=ORIENTED_EDGE('',*,*,#17451,.F.) ;
#23897=ORIENTED_EDGE('',*,*,#17452,.T.) ;
#23898=ORIENTED_EDGE('',*,*,#17297,.F.) ;
#23899=ORIENTED_EDGE('',*,*,#17450,.F.) ;
#23900=ORIENTED_EDGE('',*,*,#17453,.T.) ;
#23901=ORIENTED_EDGE('',*,*,#17454,.T.) ;
#23902=ORIENTED_EDGE('',*,*,#17298,.T.) ;
#23903=ORIENTED_EDGE('',*,*,#17452,.F.) ;
#23904=ORIENTED_EDGE('',*,*,#17455,.T.) ;
#23905=ORIENTED_EDGE('',*,*,#17456,.T.) ;
#23906=ORIENTED_EDGE('',*,*,#17299,.F.) ;
#23907=ORIENTED_EDGE('',*,*,#17454,.F.) ;
#23908=ORIENTED_EDGE('',*,*,#17457,.T.) ;
#23909=ORIENTED_EDGE('',*,*,#17458,.T.) ;
#23910=ORIENTED_EDGE('',*,*,#17300,.T.) ;
#23911=ORIENTED_EDGE('',*,*,#17456,.F.) ;
#23912=ORIENTED_EDGE('',*,*,#17459,.F.) ;
#23913=ORIENTED_EDGE('',*,*,#17460,.T.) ;
#23914=ORIENTED_EDGE('',*,*,#17301,.F.) ;
#23915=ORIENTED_EDGE('',*,*,#17458,.F.) ;
#23916=ORIENTED_EDGE('',*,*,#17461,.T.) ;
#23917=ORIENTED_EDGE('',*,*,#17447,.F.) ;
#23918=ORIENTED_EDGE('',*,*,#17302,.T.) ;
#23919=ORIENTED_EDGE('',*,*,#17460,.F.) ;
#23920=ORIENTED_EDGE('',*,*,#17462,.T.) ;
#23921=ORIENTED_EDGE('',*,*,#17455,.F.) ;
#23922=ORIENTED_EDGE('',*,*,#17463,.F.) ;
#23923=ORIENTED_EDGE('',*,*,#17464,.F.) ;
#23924=ORIENTED_EDGE('',*,*,#17465,.F.) ;
#23925=ORIENTED_EDGE('',*,*,#17453,.F.) ;
#23926=ORIENTED_EDGE('',*,*,#17466,.T.) ;
#23927=ORIENTED_EDGE('',*,*,#17467,.T.) ;
#23928=ORIENTED_EDGE('',*,*,#17468,.T.) ;
#23929=ORIENTED_EDGE('',*,*,#17469,.T.) ;
#23930=ORIENTED_EDGE('',*,*,#17470,.F.) ;
#23931=ORIENTED_EDGE('',*,*,#17471,.T.) ;
#23932=ORIENTED_EDGE('',*,*,#17472,.T.) ;
#23933=ORIENTED_EDGE('',*,*,#17473,.T.) ;
#23934=ORIENTED_EDGE('',*,*,#17463,.T.) ;
#23935=ORIENTED_EDGE('',*,*,#17451,.T.) ;
#23936=ORIENTED_EDGE('',*,*,#17474,.F.) ;
#23937=ORIENTED_EDGE('',*,*,#17475,.F.) ;
#23938=ORIENTED_EDGE('',*,*,#17466,.F.) ;
#23939=ORIENTED_EDGE('',*,*,#17448,.F.) ;
#23940=ORIENTED_EDGE('',*,*,#17476,.T.) ;
#23941=ORIENTED_EDGE('',*,*,#17477,.T.) ;
#23942=ORIENTED_EDGE('',*,*,#17474,.T.) ;
#23943=ORIENTED_EDGE('',*,*,#17478,.T.) ;
#23944=ORIENTED_EDGE('',*,*,#17479,.T.) ;
#23945=ORIENTED_EDGE('',*,*,#17480,.T.) ;
#23946=ORIENTED_EDGE('',*,*,#17312,.F.) ;
#23947=ORIENTED_EDGE('',*,*,#17481,.T.) ;
#23948=ORIENTED_EDGE('',*,*,#17313,.T.) ;
#23949=ORIENTED_EDGE('',*,*,#17480,.F.) ;
#23950=ORIENTED_EDGE('',*,*,#17482,.F.) ;
#23951=ORIENTED_EDGE('',*,*,#17483,.T.) ;
#23952=ORIENTED_EDGE('',*,*,#17314,.F.) ;
#23953=ORIENTED_EDGE('',*,*,#17481,.F.) ;
#23954=ORIENTED_EDGE('',*,*,#17484,.T.) ;
#23955=ORIENTED_EDGE('',*,*,#17485,.T.) ;
#23956=ORIENTED_EDGE('',*,*,#17315,.T.) ;
#23957=ORIENTED_EDGE('',*,*,#17483,.F.) ;
#23958=ORIENTED_EDGE('',*,*,#17486,.T.) ;
#23959=ORIENTED_EDGE('',*,*,#17487,.T.) ;
#23960=ORIENTED_EDGE('',*,*,#17316,.F.) ;
#23961=ORIENTED_EDGE('',*,*,#17485,.F.) ;
#23962=ORIENTED_EDGE('',*,*,#17488,.T.) ;
#23963=ORIENTED_EDGE('',*,*,#17489,.T.) ;
#23964=ORIENTED_EDGE('',*,*,#17317,.T.) ;
#23965=ORIENTED_EDGE('',*,*,#17487,.F.) ;
#23966=ORIENTED_EDGE('',*,*,#17490,.F.) ;
#23967=ORIENTED_EDGE('',*,*,#17491,.T.) ;
#23968=ORIENTED_EDGE('',*,*,#17318,.F.) ;
#23969=ORIENTED_EDGE('',*,*,#17489,.F.) ;
#23970=ORIENTED_EDGE('',*,*,#17492,.T.) ;
#23971=ORIENTED_EDGE('',*,*,#17478,.F.) ;
#23972=ORIENTED_EDGE('',*,*,#17319,.T.) ;
#23973=ORIENTED_EDGE('',*,*,#17491,.F.) ;
#23974=ORIENTED_EDGE('',*,*,#17493,.T.) ;
#23975=ORIENTED_EDGE('',*,*,#17486,.F.) ;
#23976=ORIENTED_EDGE('',*,*,#17494,.F.) ;
#23977=ORIENTED_EDGE('',*,*,#17495,.F.) ;
#23978=ORIENTED_EDGE('',*,*,#17496,.F.) ;
#23979=ORIENTED_EDGE('',*,*,#17484,.F.) ;
#23980=ORIENTED_EDGE('',*,*,#17497,.T.) ;
#23981=ORIENTED_EDGE('',*,*,#17498,.T.) ;
#23982=ORIENTED_EDGE('',*,*,#17499,.T.) ;
#23983=ORIENTED_EDGE('',*,*,#17500,.T.) ;
#23984=ORIENTED_EDGE('',*,*,#17501,.F.) ;
#23985=ORIENTED_EDGE('',*,*,#17502,.T.) ;
#23986=ORIENTED_EDGE('',*,*,#17503,.T.) ;
#23987=ORIENTED_EDGE('',*,*,#17504,.T.) ;
#23988=ORIENTED_EDGE('',*,*,#17494,.T.) ;
#23989=ORIENTED_EDGE('',*,*,#17482,.T.) ;
#23990=ORIENTED_EDGE('',*,*,#17505,.F.) ;
#23991=ORIENTED_EDGE('',*,*,#17506,.F.) ;
#23992=ORIENTED_EDGE('',*,*,#17497,.F.) ;
#23993=ORIENTED_EDGE('',*,*,#17479,.F.) ;
#23994=ORIENTED_EDGE('',*,*,#17507,.T.) ;
#23995=ORIENTED_EDGE('',*,*,#17508,.T.) ;
#23996=ORIENTED_EDGE('',*,*,#17505,.T.) ;
#23997=ORIENTED_EDGE('',*,*,#17509,.T.) ;
#23998=ORIENTED_EDGE('',*,*,#17510,.T.) ;
#23999=ORIENTED_EDGE('',*,*,#17511,.T.) ;
#24000=ORIENTED_EDGE('',*,*,#17329,.F.) ;
#24001=ORIENTED_EDGE('',*,*,#17512,.T.) ;
#24002=ORIENTED_EDGE('',*,*,#17330,.T.) ;
#24003=ORIENTED_EDGE('',*,*,#17511,.F.) ;
#24004=ORIENTED_EDGE('',*,*,#17513,.F.) ;
#24005=ORIENTED_EDGE('',*,*,#17514,.T.) ;
#24006=ORIENTED_EDGE('',*,*,#17331,.F.) ;
#24007=ORIENTED_EDGE('',*,*,#17512,.F.) ;
#24008=ORIENTED_EDGE('',*,*,#17515,.T.) ;
#24009=ORIENTED_EDGE('',*,*,#17516,.T.) ;
#24010=ORIENTED_EDGE('',*,*,#17332,.T.) ;
#24011=ORIENTED_EDGE('',*,*,#17514,.F.) ;
#24012=ORIENTED_EDGE('',*,*,#17517,.T.) ;
#24013=ORIENTED_EDGE('',*,*,#17518,.T.) ;
#24014=ORIENTED_EDGE('',*,*,#17333,.F.) ;
#24015=ORIENTED_EDGE('',*,*,#17516,.F.) ;
#24016=ORIENTED_EDGE('',*,*,#17519,.T.) ;
#24017=ORIENTED_EDGE('',*,*,#17520,.T.) ;
#24018=ORIENTED_EDGE('',*,*,#17334,.T.) ;
#24019=ORIENTED_EDGE('',*,*,#17518,.F.) ;
#24020=ORIENTED_EDGE('',*,*,#17521,.F.) ;
#24021=ORIENTED_EDGE('',*,*,#17522,.T.) ;
#24022=ORIENTED_EDGE('',*,*,#17335,.F.) ;
#24023=ORIENTED_EDGE('',*,*,#17520,.F.) ;
#24024=ORIENTED_EDGE('',*,*,#17523,.T.) ;
#24025=ORIENTED_EDGE('',*,*,#17509,.F.) ;
#24026=ORIENTED_EDGE('',*,*,#17336,.T.) ;
#24027=ORIENTED_EDGE('',*,*,#17522,.F.) ;
#24028=ORIENTED_EDGE('',*,*,#17524,.T.) ;
#24029=ORIENTED_EDGE('',*,*,#17517,.F.) ;
#24030=ORIENTED_EDGE('',*,*,#17525,.F.) ;
#24031=ORIENTED_EDGE('',*,*,#17526,.F.) ;
#24032=ORIENTED_EDGE('',*,*,#17527,.F.) ;
#24033=ORIENTED_EDGE('',*,*,#17515,.F.) ;
#24034=ORIENTED_EDGE('',*,*,#17528,.T.) ;
#24035=ORIENTED_EDGE('',*,*,#17529,.T.) ;
#24036=ORIENTED_EDGE('',*,*,#17530,.T.) ;
#24037=ORIENTED_EDGE('',*,*,#17531,.T.) ;
#24038=ORIENTED_EDGE('',*,*,#17532,.F.) ;
#24039=ORIENTED_EDGE('',*,*,#17533,.T.) ;
#24040=ORIENTED_EDGE('',*,*,#17534,.T.) ;
#24041=ORIENTED_EDGE('',*,*,#17535,.T.) ;
#24042=ORIENTED_EDGE('',*,*,#17525,.T.) ;
#24043=ORIENTED_EDGE('',*,*,#17513,.T.) ;
#24044=ORIENTED_EDGE('',*,*,#17536,.F.) ;
#24045=ORIENTED_EDGE('',*,*,#17537,.F.) ;
#24046=ORIENTED_EDGE('',*,*,#17528,.F.) ;
#24047=ORIENTED_EDGE('',*,*,#17510,.F.) ;
#24048=ORIENTED_EDGE('',*,*,#17538,.T.) ;
#24049=ORIENTED_EDGE('',*,*,#17539,.T.) ;
#24050=ORIENTED_EDGE('',*,*,#17536,.T.) ;
#24051=ORIENTED_EDGE('',*,*,#17540,.T.) ;
#24052=ORIENTED_EDGE('',*,*,#17541,.T.) ;
#24053=ORIENTED_EDGE('',*,*,#17542,.T.) ;
#24054=ORIENTED_EDGE('',*,*,#17346,.F.) ;
#24055=ORIENTED_EDGE('',*,*,#17543,.T.) ;
#24056=ORIENTED_EDGE('',*,*,#17347,.T.) ;
#24057=ORIENTED_EDGE('',*,*,#17542,.F.) ;
#24058=ORIENTED_EDGE('',*,*,#17544,.F.) ;
#24059=ORIENTED_EDGE('',*,*,#17545,.T.) ;
#24060=ORIENTED_EDGE('',*,*,#17348,.F.) ;
#24061=ORIENTED_EDGE('',*,*,#17543,.F.) ;
#24062=ORIENTED_EDGE('',*,*,#17546,.T.) ;
#24063=ORIENTED_EDGE('',*,*,#17547,.T.) ;
#24064=ORIENTED_EDGE('',*,*,#17349,.T.) ;
#24065=ORIENTED_EDGE('',*,*,#17545,.F.) ;
#24066=ORIENTED_EDGE('',*,*,#17548,.T.) ;
#24067=ORIENTED_EDGE('',*,*,#17549,.T.) ;
#24068=ORIENTED_EDGE('',*,*,#17350,.F.) ;
#24069=ORIENTED_EDGE('',*,*,#17547,.F.) ;
#24070=ORIENTED_EDGE('',*,*,#17550,.T.) ;
#24071=ORIENTED_EDGE('',*,*,#17551,.T.) ;
#24072=ORIENTED_EDGE('',*,*,#17351,.T.) ;
#24073=ORIENTED_EDGE('',*,*,#17549,.F.) ;
#24074=ORIENTED_EDGE('',*,*,#17552,.F.) ;
#24075=ORIENTED_EDGE('',*,*,#17553,.T.) ;
#24076=ORIENTED_EDGE('',*,*,#17352,.F.) ;
#24077=ORIENTED_EDGE('',*,*,#17551,.F.) ;
#24078=ORIENTED_EDGE('',*,*,#17554,.T.) ;
#24079=ORIENTED_EDGE('',*,*,#17540,.F.) ;
#24080=ORIENTED_EDGE('',*,*,#17353,.T.) ;
#24081=ORIENTED_EDGE('',*,*,#17553,.F.) ;
#24082=ORIENTED_EDGE('',*,*,#17555,.T.) ;
#24083=ORIENTED_EDGE('',*,*,#17548,.F.) ;
#24084=ORIENTED_EDGE('',*,*,#17556,.F.) ;
#24085=ORIENTED_EDGE('',*,*,#17557,.F.) ;
#24086=ORIENTED_EDGE('',*,*,#17558,.F.) ;
#24087=ORIENTED_EDGE('',*,*,#17546,.F.) ;
#24088=ORIENTED_EDGE('',*,*,#17559,.T.) ;
#24089=ORIENTED_EDGE('',*,*,#17560,.T.) ;
#24090=ORIENTED_EDGE('',*,*,#17561,.T.) ;
#24091=ORIENTED_EDGE('',*,*,#17562,.T.) ;
#24092=ORIENTED_EDGE('',*,*,#17563,.F.) ;
#24093=ORIENTED_EDGE('',*,*,#17564,.T.) ;
#24094=ORIENTED_EDGE('',*,*,#17565,.T.) ;
#24095=ORIENTED_EDGE('',*,*,#17566,.T.) ;
#24096=ORIENTED_EDGE('',*,*,#17556,.T.) ;
#24097=ORIENTED_EDGE('',*,*,#17544,.T.) ;
#24098=ORIENTED_EDGE('',*,*,#17567,.F.) ;
#24099=ORIENTED_EDGE('',*,*,#17568,.F.) ;
#24100=ORIENTED_EDGE('',*,*,#17559,.F.) ;
#24101=ORIENTED_EDGE('',*,*,#17541,.F.) ;
#24102=ORIENTED_EDGE('',*,*,#17569,.T.) ;
#24103=ORIENTED_EDGE('',*,*,#17570,.T.) ;
#24104=ORIENTED_EDGE('',*,*,#17567,.T.) ;
#24105=ORIENTED_EDGE('',*,*,#17571,.T.) ;
#24106=ORIENTED_EDGE('',*,*,#17572,.T.) ;
#24107=ORIENTED_EDGE('',*,*,#17573,.T.) ;
#24108=ORIENTED_EDGE('',*,*,#17363,.F.) ;
#24109=ORIENTED_EDGE('',*,*,#17574,.T.) ;
#24110=ORIENTED_EDGE('',*,*,#17364,.T.) ;
#24111=ORIENTED_EDGE('',*,*,#17573,.F.) ;
#24112=ORIENTED_EDGE('',*,*,#17575,.F.) ;
#24113=ORIENTED_EDGE('',*,*,#17576,.T.) ;
#24114=ORIENTED_EDGE('',*,*,#17365,.F.) ;
#24115=ORIENTED_EDGE('',*,*,#17574,.F.) ;
#24116=ORIENTED_EDGE('',*,*,#17577,.T.) ;
#24117=ORIENTED_EDGE('',*,*,#17578,.T.) ;
#24118=ORIENTED_EDGE('',*,*,#17366,.T.) ;
#24119=ORIENTED_EDGE('',*,*,#17576,.F.) ;
#24120=ORIENTED_EDGE('',*,*,#17579,.T.) ;
#24121=ORIENTED_EDGE('',*,*,#17580,.T.) ;
#24122=ORIENTED_EDGE('',*,*,#17367,.F.) ;
#24123=ORIENTED_EDGE('',*,*,#17578,.F.) ;
#24124=ORIENTED_EDGE('',*,*,#17581,.T.) ;
#24125=ORIENTED_EDGE('',*,*,#17582,.T.) ;
#24126=ORIENTED_EDGE('',*,*,#17368,.T.) ;
#24127=ORIENTED_EDGE('',*,*,#17580,.F.) ;
#24128=ORIENTED_EDGE('',*,*,#17583,.F.) ;
#24129=ORIENTED_EDGE('',*,*,#17584,.T.) ;
#24130=ORIENTED_EDGE('',*,*,#17369,.F.) ;
#24131=ORIENTED_EDGE('',*,*,#17582,.F.) ;
#24132=ORIENTED_EDGE('',*,*,#17585,.T.) ;
#24133=ORIENTED_EDGE('',*,*,#17571,.F.) ;
#24134=ORIENTED_EDGE('',*,*,#17370,.T.) ;
#24135=ORIENTED_EDGE('',*,*,#17584,.F.) ;
#24136=ORIENTED_EDGE('',*,*,#17586,.T.) ;
#24137=ORIENTED_EDGE('',*,*,#17579,.F.) ;
#24138=ORIENTED_EDGE('',*,*,#17587,.F.) ;
#24139=ORIENTED_EDGE('',*,*,#17588,.F.) ;
#24140=ORIENTED_EDGE('',*,*,#17589,.F.) ;
#24141=ORIENTED_EDGE('',*,*,#17577,.F.) ;
#24142=ORIENTED_EDGE('',*,*,#17590,.T.) ;
#24143=ORIENTED_EDGE('',*,*,#17591,.T.) ;
#24144=ORIENTED_EDGE('',*,*,#17592,.T.) ;
#24145=ORIENTED_EDGE('',*,*,#17593,.T.) ;
#24146=ORIENTED_EDGE('',*,*,#17594,.F.) ;
#24147=ORIENTED_EDGE('',*,*,#17595,.T.) ;
#24148=ORIENTED_EDGE('',*,*,#17596,.T.) ;
#24149=ORIENTED_EDGE('',*,*,#17597,.T.) ;
#24150=ORIENTED_EDGE('',*,*,#17587,.T.) ;
#24151=ORIENTED_EDGE('',*,*,#17575,.T.) ;
#24152=ORIENTED_EDGE('',*,*,#17598,.F.) ;
#24153=ORIENTED_EDGE('',*,*,#17599,.F.) ;
#24154=ORIENTED_EDGE('',*,*,#17590,.F.) ;
#24155=ORIENTED_EDGE('',*,*,#17572,.F.) ;
#24156=ORIENTED_EDGE('',*,*,#17600,.T.) ;
#24157=ORIENTED_EDGE('',*,*,#17601,.T.) ;
#24158=ORIENTED_EDGE('',*,*,#17598,.T.) ;
#24159=ORIENTED_EDGE('',*,*,#17602,.T.) ;
#24160=ORIENTED_EDGE('',*,*,#17603,.T.) ;
#24161=ORIENTED_EDGE('',*,*,#17604,.T.) ;
#24162=ORIENTED_EDGE('',*,*,#17380,.F.) ;
#24163=ORIENTED_EDGE('',*,*,#17605,.T.) ;
#24164=ORIENTED_EDGE('',*,*,#17381,.T.) ;
#24165=ORIENTED_EDGE('',*,*,#17604,.F.) ;
#24166=ORIENTED_EDGE('',*,*,#17606,.F.) ;
#24167=ORIENTED_EDGE('',*,*,#17607,.T.) ;
#24168=ORIENTED_EDGE('',*,*,#17382,.F.) ;
#24169=ORIENTED_EDGE('',*,*,#17605,.F.) ;
#24170=ORIENTED_EDGE('',*,*,#17608,.T.) ;
#24171=ORIENTED_EDGE('',*,*,#17609,.T.) ;
#24172=ORIENTED_EDGE('',*,*,#17383,.T.) ;
#24173=ORIENTED_EDGE('',*,*,#17607,.F.) ;
#24174=ORIENTED_EDGE('',*,*,#17610,.T.) ;
#24175=ORIENTED_EDGE('',*,*,#17611,.T.) ;
#24176=ORIENTED_EDGE('',*,*,#17384,.F.) ;
#24177=ORIENTED_EDGE('',*,*,#17609,.F.) ;
#24178=ORIENTED_EDGE('',*,*,#17612,.T.) ;
#24179=ORIENTED_EDGE('',*,*,#17613,.T.) ;
#24180=ORIENTED_EDGE('',*,*,#17385,.T.) ;
#24181=ORIENTED_EDGE('',*,*,#17611,.F.) ;
#24182=ORIENTED_EDGE('',*,*,#17614,.F.) ;
#24183=ORIENTED_EDGE('',*,*,#17615,.T.) ;
#24184=ORIENTED_EDGE('',*,*,#17386,.F.) ;
#24185=ORIENTED_EDGE('',*,*,#17613,.F.) ;
#24186=ORIENTED_EDGE('',*,*,#17616,.T.) ;
#24187=ORIENTED_EDGE('',*,*,#17602,.F.) ;
#24188=ORIENTED_EDGE('',*,*,#17387,.T.) ;
#24189=ORIENTED_EDGE('',*,*,#17615,.F.) ;
#24190=ORIENTED_EDGE('',*,*,#17617,.T.) ;
#24191=ORIENTED_EDGE('',*,*,#17610,.F.) ;
#24192=ORIENTED_EDGE('',*,*,#17618,.F.) ;
#24193=ORIENTED_EDGE('',*,*,#17619,.F.) ;
#24194=ORIENTED_EDGE('',*,*,#17620,.F.) ;
#24195=ORIENTED_EDGE('',*,*,#17608,.F.) ;
#24196=ORIENTED_EDGE('',*,*,#17621,.T.) ;
#24197=ORIENTED_EDGE('',*,*,#17622,.T.) ;
#24198=ORIENTED_EDGE('',*,*,#17623,.T.) ;
#24199=ORIENTED_EDGE('',*,*,#17624,.T.) ;
#24200=ORIENTED_EDGE('',*,*,#17625,.F.) ;
#24201=ORIENTED_EDGE('',*,*,#17626,.T.) ;
#24202=ORIENTED_EDGE('',*,*,#17627,.T.) ;
#24203=ORIENTED_EDGE('',*,*,#17628,.T.) ;
#24204=ORIENTED_EDGE('',*,*,#17618,.T.) ;
#24205=ORIENTED_EDGE('',*,*,#17606,.T.) ;
#24206=ORIENTED_EDGE('',*,*,#17629,.F.) ;
#24207=ORIENTED_EDGE('',*,*,#17630,.F.) ;
#24208=ORIENTED_EDGE('',*,*,#17621,.F.) ;
#24209=ORIENTED_EDGE('',*,*,#17603,.F.) ;
#24210=ORIENTED_EDGE('',*,*,#17631,.T.) ;
#24211=ORIENTED_EDGE('',*,*,#17632,.T.) ;
#24212=ORIENTED_EDGE('',*,*,#17629,.T.) ;
#24213=ORIENTED_EDGE('',*,*,#17633,.T.) ;
#24214=ORIENTED_EDGE('',*,*,#17634,.T.) ;
#24215=ORIENTED_EDGE('',*,*,#17635,.T.) ;
#24216=ORIENTED_EDGE('',*,*,#17397,.F.) ;
#24217=ORIENTED_EDGE('',*,*,#17636,.T.) ;
#24218=ORIENTED_EDGE('',*,*,#17398,.T.) ;
#24219=ORIENTED_EDGE('',*,*,#17635,.F.) ;
#24220=ORIENTED_EDGE('',*,*,#17637,.F.) ;
#24221=ORIENTED_EDGE('',*,*,#17638,.T.) ;
#24222=ORIENTED_EDGE('',*,*,#17399,.F.) ;
#24223=ORIENTED_EDGE('',*,*,#17636,.F.) ;
#24224=ORIENTED_EDGE('',*,*,#17639,.T.) ;
#24225=ORIENTED_EDGE('',*,*,#17640,.T.) ;
#24226=ORIENTED_EDGE('',*,*,#17400,.T.) ;
#24227=ORIENTED_EDGE('',*,*,#17638,.F.) ;
#24228=ORIENTED_EDGE('',*,*,#17641,.T.) ;
#24229=ORIENTED_EDGE('',*,*,#17642,.T.) ;
#24230=ORIENTED_EDGE('',*,*,#17401,.F.) ;
#24231=ORIENTED_EDGE('',*,*,#17640,.F.) ;
#24232=ORIENTED_EDGE('',*,*,#17643,.T.) ;
#24233=ORIENTED_EDGE('',*,*,#17644,.T.) ;
#24234=ORIENTED_EDGE('',*,*,#17402,.T.) ;
#24235=ORIENTED_EDGE('',*,*,#17642,.F.) ;
#24236=ORIENTED_EDGE('',*,*,#17645,.F.) ;
#24237=ORIENTED_EDGE('',*,*,#17646,.T.) ;
#24238=ORIENTED_EDGE('',*,*,#17403,.F.) ;
#24239=ORIENTED_EDGE('',*,*,#17644,.F.) ;
#24240=ORIENTED_EDGE('',*,*,#17647,.T.) ;
#24241=ORIENTED_EDGE('',*,*,#17633,.F.) ;
#24242=ORIENTED_EDGE('',*,*,#17404,.T.) ;
#24243=ORIENTED_EDGE('',*,*,#17646,.F.) ;
#24244=ORIENTED_EDGE('',*,*,#17648,.T.) ;
#24245=ORIENTED_EDGE('',*,*,#17641,.F.) ;
#24246=ORIENTED_EDGE('',*,*,#17649,.F.) ;
#24247=ORIENTED_EDGE('',*,*,#17650,.F.) ;
#24248=ORIENTED_EDGE('',*,*,#17651,.F.) ;
#24249=ORIENTED_EDGE('',*,*,#17639,.F.) ;
#24250=ORIENTED_EDGE('',*,*,#17652,.T.) ;
#24251=ORIENTED_EDGE('',*,*,#17653,.T.) ;
#24252=ORIENTED_EDGE('',*,*,#17654,.T.) ;
#24253=ORIENTED_EDGE('',*,*,#17655,.T.) ;
#24254=ORIENTED_EDGE('',*,*,#17656,.F.) ;
#24255=ORIENTED_EDGE('',*,*,#17657,.T.) ;
#24256=ORIENTED_EDGE('',*,*,#17658,.T.) ;
#24257=ORIENTED_EDGE('',*,*,#17659,.T.) ;
#24258=ORIENTED_EDGE('',*,*,#17649,.T.) ;
#24259=ORIENTED_EDGE('',*,*,#17637,.T.) ;
#24260=ORIENTED_EDGE('',*,*,#17660,.F.) ;
#24261=ORIENTED_EDGE('',*,*,#17661,.F.) ;
#24262=ORIENTED_EDGE('',*,*,#17652,.F.) ;
#24263=ORIENTED_EDGE('',*,*,#17634,.F.) ;
#24264=ORIENTED_EDGE('',*,*,#17662,.T.) ;
#24265=ORIENTED_EDGE('',*,*,#17663,.T.) ;
#24266=ORIENTED_EDGE('',*,*,#17660,.T.) ;
#24267=ORIENTED_EDGE('',*,*,#17664,.T.) ;
#24268=ORIENTED_EDGE('',*,*,#17665,.T.) ;
#24269=ORIENTED_EDGE('',*,*,#17666,.T.) ;
#24270=ORIENTED_EDGE('',*,*,#17414,.F.) ;
#24271=ORIENTED_EDGE('',*,*,#17667,.T.) ;
#24272=ORIENTED_EDGE('',*,*,#17415,.T.) ;
#24273=ORIENTED_EDGE('',*,*,#17666,.F.) ;
#24274=ORIENTED_EDGE('',*,*,#17668,.F.) ;
#24275=ORIENTED_EDGE('',*,*,#17669,.T.) ;
#24276=ORIENTED_EDGE('',*,*,#17416,.F.) ;
#24277=ORIENTED_EDGE('',*,*,#17667,.F.) ;
#24278=ORIENTED_EDGE('',*,*,#17670,.T.) ;
#24279=ORIENTED_EDGE('',*,*,#17671,.T.) ;
#24280=ORIENTED_EDGE('',*,*,#17417,.T.) ;
#24281=ORIENTED_EDGE('',*,*,#17669,.F.) ;
#24282=ORIENTED_EDGE('',*,*,#17672,.T.) ;
#24283=ORIENTED_EDGE('',*,*,#17673,.T.) ;
#24284=ORIENTED_EDGE('',*,*,#17418,.F.) ;
#24285=ORIENTED_EDGE('',*,*,#17671,.F.) ;
#24286=ORIENTED_EDGE('',*,*,#17674,.T.) ;
#24287=ORIENTED_EDGE('',*,*,#17675,.T.) ;
#24288=ORIENTED_EDGE('',*,*,#17419,.T.) ;
#24289=ORIENTED_EDGE('',*,*,#17673,.F.) ;
#24290=ORIENTED_EDGE('',*,*,#17676,.F.) ;
#24291=ORIENTED_EDGE('',*,*,#17677,.T.) ;
#24292=ORIENTED_EDGE('',*,*,#17420,.F.) ;
#24293=ORIENTED_EDGE('',*,*,#17675,.F.) ;
#24294=ORIENTED_EDGE('',*,*,#17678,.T.) ;
#24295=ORIENTED_EDGE('',*,*,#17664,.F.) ;
#24296=ORIENTED_EDGE('',*,*,#17421,.T.) ;
#24297=ORIENTED_EDGE('',*,*,#17677,.F.) ;
#24298=ORIENTED_EDGE('',*,*,#17679,.T.) ;
#24299=ORIENTED_EDGE('',*,*,#17672,.F.) ;
#24300=ORIENTED_EDGE('',*,*,#17680,.F.) ;
#24301=ORIENTED_EDGE('',*,*,#17681,.F.) ;
#24302=ORIENTED_EDGE('',*,*,#17682,.F.) ;
#24303=ORIENTED_EDGE('',*,*,#17670,.F.) ;
#24304=ORIENTED_EDGE('',*,*,#17683,.T.) ;
#24305=ORIENTED_EDGE('',*,*,#17684,.T.) ;
#24306=ORIENTED_EDGE('',*,*,#17685,.T.) ;
#24307=ORIENTED_EDGE('',*,*,#17686,.T.) ;
#24308=ORIENTED_EDGE('',*,*,#17687,.F.) ;
#24309=ORIENTED_EDGE('',*,*,#17688,.T.) ;
#24310=ORIENTED_EDGE('',*,*,#17689,.T.) ;
#24311=ORIENTED_EDGE('',*,*,#17690,.T.) ;
#24312=ORIENTED_EDGE('',*,*,#17680,.T.) ;
#24313=ORIENTED_EDGE('',*,*,#17668,.T.) ;
#24314=ORIENTED_EDGE('',*,*,#17691,.F.) ;
#24315=ORIENTED_EDGE('',*,*,#17692,.F.) ;
#24316=ORIENTED_EDGE('',*,*,#17683,.F.) ;
#24317=ORIENTED_EDGE('',*,*,#17665,.F.) ;
#24318=ORIENTED_EDGE('',*,*,#17693,.T.) ;
#24319=ORIENTED_EDGE('',*,*,#17694,.T.) ;
#24320=ORIENTED_EDGE('',*,*,#17691,.T.) ;
#24321=ORIENTED_EDGE('',*,*,#17695,.T.) ;
#24322=ORIENTED_EDGE('',*,*,#17696,.T.) ;
#24323=ORIENTED_EDGE('',*,*,#17697,.T.) ;
#24324=ORIENTED_EDGE('',*,*,#17429,.T.) ;
#24325=ORIENTED_EDGE('',*,*,#17698,.T.) ;
#24326=ORIENTED_EDGE('',*,*,#17430,.T.) ;
#24327=ORIENTED_EDGE('',*,*,#17697,.F.) ;
#24328=ORIENTED_EDGE('',*,*,#17699,.T.) ;
#24329=ORIENTED_EDGE('',*,*,#17700,.T.) ;
#24330=ORIENTED_EDGE('',*,*,#17431,.T.) ;
#24331=ORIENTED_EDGE('',*,*,#17698,.F.) ;
#24332=ORIENTED_EDGE('',*,*,#17701,.T.) ;
#24333=ORIENTED_EDGE('',*,*,#17702,.T.) ;
#24334=ORIENTED_EDGE('',*,*,#17432,.T.) ;
#24335=ORIENTED_EDGE('',*,*,#17700,.F.) ;
#24336=ORIENTED_EDGE('',*,*,#17703,.T.) ;
#24337=ORIENTED_EDGE('',*,*,#17704,.T.) ;
#24338=ORIENTED_EDGE('',*,*,#17433,.T.) ;
#24339=ORIENTED_EDGE('',*,*,#17702,.F.) ;
#24340=ORIENTED_EDGE('',*,*,#17705,.T.) ;
#24341=ORIENTED_EDGE('',*,*,#17706,.T.) ;
#24342=ORIENTED_EDGE('',*,*,#17434,.T.) ;
#24343=ORIENTED_EDGE('',*,*,#17704,.F.) ;
#24344=ORIENTED_EDGE('',*,*,#17707,.T.) ;
#24345=ORIENTED_EDGE('',*,*,#17708,.T.) ;
#24346=ORIENTED_EDGE('',*,*,#17435,.T.) ;
#24347=ORIENTED_EDGE('',*,*,#17706,.F.) ;
#24348=ORIENTED_EDGE('',*,*,#17709,.T.) ;
#24349=ORIENTED_EDGE('',*,*,#17695,.F.) ;
#24350=ORIENTED_EDGE('',*,*,#17436,.T.) ;
#24351=ORIENTED_EDGE('',*,*,#17708,.F.) ;
#24352=ORIENTED_EDGE('',*,*,#17710,.T.) ;
#24353=ORIENTED_EDGE('',*,*,#17703,.F.) ;
#24354=ORIENTED_EDGE('',*,*,#17711,.F.) ;
#24355=ORIENTED_EDGE('',*,*,#17712,.F.) ;
#24356=ORIENTED_EDGE('',*,*,#17713,.F.) ;
#24357=ORIENTED_EDGE('',*,*,#17714,.F.) ;
#24358=ORIENTED_EDGE('',*,*,#17715,.T.) ;
#24359=ORIENTED_EDGE('',*,*,#17716,.T.) ;
#24360=ORIENTED_EDGE('',*,*,#17717,.T.) ;
#24361=ORIENTED_EDGE('',*,*,#17711,.T.) ;
#24362=ORIENTED_EDGE('',*,*,#17701,.F.) ;
#24363=ORIENTED_EDGE('',*,*,#17718,.T.) ;
#24364=ORIENTED_EDGE('',*,*,#17719,.T.) ;
#24365=ORIENTED_EDGE('',*,*,#17720,.T.) ;
#24366=ORIENTED_EDGE('',*,*,#17721,.T.) ;
#24367=ORIENTED_EDGE('',*,*,#17699,.F.) ;
#24368=ORIENTED_EDGE('',*,*,#17722,.F.) ;
#24369=ORIENTED_EDGE('',*,*,#17723,.F.) ;
#24370=ORIENTED_EDGE('',*,*,#17718,.F.) ;
#24371=ORIENTED_EDGE('',*,*,#17696,.F.) ;
#24372=ORIENTED_EDGE('',*,*,#17724,.T.) ;
#24373=ORIENTED_EDGE('',*,*,#17725,.T.) ;
#24374=ORIENTED_EDGE('',*,*,#17722,.T.) ;
#24375=ORIENTED_EDGE('',*,*,#17726,.T.) ;
#24376=ORIENTED_EDGE('',*,*,#17727,.T.) ;
#24377=ORIENTED_EDGE('',*,*,#17728,.T.) ;
#24378=ORIENTED_EDGE('',*,*,#17729,.F.) ;
#24379=ORIENTED_EDGE('',*,*,#17730,.T.) ;
#24380=ORIENTED_EDGE('',*,*,#17731,.T.) ;
#24381=ORIENTED_EDGE('',*,*,#17728,.F.) ;
#24382=ORIENTED_EDGE('',*,*,#17732,.T.) ;
#24383=ORIENTED_EDGE('',*,*,#17733,.T.) ;
#24384=ORIENTED_EDGE('',*,*,#17734,.F.) ;
#24385=ORIENTED_EDGE('',*,*,#17730,.F.) ;
#24386=ORIENTED_EDGE('',*,*,#17735,.T.) ;
#24387=ORIENTED_EDGE('',*,*,#17736,.T.) ;
#24388=ORIENTED_EDGE('',*,*,#17737,.T.) ;
#24389=ORIENTED_EDGE('',*,*,#17733,.F.) ;
#24390=ORIENTED_EDGE('',*,*,#17738,.F.) ;
#24391=ORIENTED_EDGE('',*,*,#17739,.T.) ;
#24392=ORIENTED_EDGE('',*,*,#17740,.F.) ;
#24393=ORIENTED_EDGE('',*,*,#17736,.F.) ;
#24394=ORIENTED_EDGE('',*,*,#17741,.T.) ;
#24395=ORIENTED_EDGE('',*,*,#17742,.T.) ;
#24396=ORIENTED_EDGE('',*,*,#17743,.T.) ;
#24397=ORIENTED_EDGE('',*,*,#17739,.F.) ;
#24398=ORIENTED_EDGE('',*,*,#17744,.T.) ;
#24399=ORIENTED_EDGE('',*,*,#17745,.T.) ;
#24400=ORIENTED_EDGE('',*,*,#17746,.F.) ;
#24401=ORIENTED_EDGE('',*,*,#17742,.F.) ;
#24402=ORIENTED_EDGE('',*,*,#17747,.T.) ;
#24403=ORIENTED_EDGE('',*,*,#17726,.F.) ;
#24404=ORIENTED_EDGE('',*,*,#17748,.T.) ;
#24405=ORIENTED_EDGE('',*,*,#17745,.F.) ;
#24406=ORIENTED_EDGE('',*,*,#17749,.F.) ;
#24407=ORIENTED_EDGE('',*,*,#17738,.T.) ;
#24408=ORIENTED_EDGE('',*,*,#17750,.F.) ;
#24409=ORIENTED_EDGE('',*,*,#17751,.F.) ;
#24410=ORIENTED_EDGE('',*,*,#17752,.F.) ;
#24411=ORIENTED_EDGE('',*,*,#17735,.F.) ;
#24412=ORIENTED_EDGE('',*,*,#17753,.T.) ;
#24413=ORIENTED_EDGE('',*,*,#17754,.T.) ;
#24414=ORIENTED_EDGE('',*,*,#17750,.T.) ;
#24415=ORIENTED_EDGE('',*,*,#17732,.F.) ;
#24416=ORIENTED_EDGE('',*,*,#17755,.F.) ;
#24417=ORIENTED_EDGE('',*,*,#17756,.F.) ;
#24418=ORIENTED_EDGE('',*,*,#17753,.F.) ;
#24419=ORIENTED_EDGE('',*,*,#17727,.F.) ;
#24420=ORIENTED_EDGE('',*,*,#17757,.T.) ;
#24421=ORIENTED_EDGE('',*,*,#17758,.T.) ;
#24422=ORIENTED_EDGE('',*,*,#17755,.T.) ;
#24423=ORIENTED_EDGE('',*,*,#17759,.T.) ;
#24424=ORIENTED_EDGE('',*,*,#17760,.T.) ;
#24425=ORIENTED_EDGE('',*,*,#17761,.T.) ;
#24426=ORIENTED_EDGE('',*,*,#17762,.F.) ;
#24427=ORIENTED_EDGE('',*,*,#17763,.T.) ;
#24428=ORIENTED_EDGE('',*,*,#17764,.T.) ;
#24429=ORIENTED_EDGE('',*,*,#17761,.F.) ;
#24430=ORIENTED_EDGE('',*,*,#17765,.T.) ;
#24431=ORIENTED_EDGE('',*,*,#17766,.T.) ;
#24432=ORIENTED_EDGE('',*,*,#17767,.F.) ;
#24433=ORIENTED_EDGE('',*,*,#17763,.F.) ;
#24434=ORIENTED_EDGE('',*,*,#17768,.T.) ;
#24435=ORIENTED_EDGE('',*,*,#17769,.T.) ;
#24436=ORIENTED_EDGE('',*,*,#17770,.T.) ;
#24437=ORIENTED_EDGE('',*,*,#17766,.F.) ;
#24438=ORIENTED_EDGE('',*,*,#17771,.F.) ;
#24439=ORIENTED_EDGE('',*,*,#17772,.T.) ;
#24440=ORIENTED_EDGE('',*,*,#17773,.F.) ;
#24441=ORIENTED_EDGE('',*,*,#17769,.F.) ;
#24442=ORIENTED_EDGE('',*,*,#17774,.T.) ;
#24443=ORIENTED_EDGE('',*,*,#17775,.T.) ;
#24444=ORIENTED_EDGE('',*,*,#17776,.T.) ;
#24445=ORIENTED_EDGE('',*,*,#17772,.F.) ;
#24446=ORIENTED_EDGE('',*,*,#17777,.T.) ;
#24447=ORIENTED_EDGE('',*,*,#17778,.T.) ;
#24448=ORIENTED_EDGE('',*,*,#17779,.F.) ;
#24449=ORIENTED_EDGE('',*,*,#17775,.F.) ;
#24450=ORIENTED_EDGE('',*,*,#17780,.T.) ;
#24451=ORIENTED_EDGE('',*,*,#17759,.F.) ;
#24452=ORIENTED_EDGE('',*,*,#17781,.T.) ;
#24453=ORIENTED_EDGE('',*,*,#17778,.F.) ;
#24454=ORIENTED_EDGE('',*,*,#17782,.F.) ;
#24455=ORIENTED_EDGE('',*,*,#17771,.T.) ;
#24456=ORIENTED_EDGE('',*,*,#17783,.F.) ;
#24457=ORIENTED_EDGE('',*,*,#17784,.F.) ;
#24458=ORIENTED_EDGE('',*,*,#17785,.F.) ;
#24459=ORIENTED_EDGE('',*,*,#17768,.F.) ;
#24460=ORIENTED_EDGE('',*,*,#17786,.T.) ;
#24461=ORIENTED_EDGE('',*,*,#17787,.T.) ;
#24462=ORIENTED_EDGE('',*,*,#17783,.T.) ;
#24463=ORIENTED_EDGE('',*,*,#17765,.F.) ;
#24464=ORIENTED_EDGE('',*,*,#17788,.F.) ;
#24465=ORIENTED_EDGE('',*,*,#17789,.F.) ;
#24466=ORIENTED_EDGE('',*,*,#17786,.F.) ;
#24467=ORIENTED_EDGE('',*,*,#17760,.F.) ;
#24468=ORIENTED_EDGE('',*,*,#17790,.T.) ;
#24469=ORIENTED_EDGE('',*,*,#17791,.T.) ;
#24470=ORIENTED_EDGE('',*,*,#17788,.T.) ;
#24471=ORIENTED_EDGE('',*,*,#17792,.T.) ;
#24472=ORIENTED_EDGE('',*,*,#17793,.T.) ;
#24473=ORIENTED_EDGE('',*,*,#17794,.T.) ;
#24474=ORIENTED_EDGE('',*,*,#17795,.F.) ;
#24475=ORIENTED_EDGE('',*,*,#17796,.T.) ;
#24476=ORIENTED_EDGE('',*,*,#17797,.T.) ;
#24477=ORIENTED_EDGE('',*,*,#17794,.F.) ;
#24478=ORIENTED_EDGE('',*,*,#17798,.T.) ;
#24479=ORIENTED_EDGE('',*,*,#17799,.T.) ;
#24480=ORIENTED_EDGE('',*,*,#17800,.F.) ;
#24481=ORIENTED_EDGE('',*,*,#17796,.F.) ;
#24482=ORIENTED_EDGE('',*,*,#17801,.T.) ;
#24483=ORIENTED_EDGE('',*,*,#17802,.T.) ;
#24484=ORIENTED_EDGE('',*,*,#17803,.T.) ;
#24485=ORIENTED_EDGE('',*,*,#17799,.F.) ;
#24486=ORIENTED_EDGE('',*,*,#17804,.F.) ;
#24487=ORIENTED_EDGE('',*,*,#17805,.T.) ;
#24488=ORIENTED_EDGE('',*,*,#17806,.F.) ;
#24489=ORIENTED_EDGE('',*,*,#17802,.F.) ;
#24490=ORIENTED_EDGE('',*,*,#17807,.T.) ;
#24491=ORIENTED_EDGE('',*,*,#17808,.T.) ;
#24492=ORIENTED_EDGE('',*,*,#17809,.T.) ;
#24493=ORIENTED_EDGE('',*,*,#17805,.F.) ;
#24494=ORIENTED_EDGE('',*,*,#17810,.T.) ;
#24495=ORIENTED_EDGE('',*,*,#17811,.T.) ;
#24496=ORIENTED_EDGE('',*,*,#17812,.F.) ;
#24497=ORIENTED_EDGE('',*,*,#17808,.F.) ;
#24498=ORIENTED_EDGE('',*,*,#17813,.T.) ;
#24499=ORIENTED_EDGE('',*,*,#17792,.F.) ;
#24500=ORIENTED_EDGE('',*,*,#17814,.T.) ;
#24501=ORIENTED_EDGE('',*,*,#17811,.F.) ;
#24502=ORIENTED_EDGE('',*,*,#17815,.F.) ;
#24503=ORIENTED_EDGE('',*,*,#17804,.T.) ;
#24504=ORIENTED_EDGE('',*,*,#17816,.F.) ;
#24505=ORIENTED_EDGE('',*,*,#17817,.F.) ;
#24506=ORIENTED_EDGE('',*,*,#17818,.F.) ;
#24507=ORIENTED_EDGE('',*,*,#17801,.F.) ;
#24508=ORIENTED_EDGE('',*,*,#17819,.T.) ;
#24509=ORIENTED_EDGE('',*,*,#17820,.T.) ;
#24510=ORIENTED_EDGE('',*,*,#17816,.T.) ;
#24511=ORIENTED_EDGE('',*,*,#17798,.F.) ;
#24512=ORIENTED_EDGE('',*,*,#17821,.F.) ;
#24513=ORIENTED_EDGE('',*,*,#17822,.F.) ;
#24514=ORIENTED_EDGE('',*,*,#17819,.F.) ;
#24515=ORIENTED_EDGE('',*,*,#17793,.F.) ;
#24516=ORIENTED_EDGE('',*,*,#17823,.T.) ;
#24517=ORIENTED_EDGE('',*,*,#17824,.T.) ;
#24518=ORIENTED_EDGE('',*,*,#17821,.T.) ;
#24519=ORIENTED_EDGE('',*,*,#17825,.T.) ;
#24520=ORIENTED_EDGE('',*,*,#17826,.T.) ;
#24521=ORIENTED_EDGE('',*,*,#17827,.T.) ;
#24522=ORIENTED_EDGE('',*,*,#17828,.F.) ;
#24523=ORIENTED_EDGE('',*,*,#17829,.T.) ;
#24524=ORIENTED_EDGE('',*,*,#17830,.T.) ;
#24525=ORIENTED_EDGE('',*,*,#17827,.F.) ;
#24526=ORIENTED_EDGE('',*,*,#17831,.T.) ;
#24527=ORIENTED_EDGE('',*,*,#17832,.T.) ;
#24528=ORIENTED_EDGE('',*,*,#17833,.F.) ;
#24529=ORIENTED_EDGE('',*,*,#17829,.F.) ;
#24530=ORIENTED_EDGE('',*,*,#17834,.T.) ;
#24531=ORIENTED_EDGE('',*,*,#17835,.T.) ;
#24532=ORIENTED_EDGE('',*,*,#17836,.T.) ;
#24533=ORIENTED_EDGE('',*,*,#17832,.F.) ;
#24534=ORIENTED_EDGE('',*,*,#17837,.F.) ;
#24535=ORIENTED_EDGE('',*,*,#17838,.T.) ;
#24536=ORIENTED_EDGE('',*,*,#17839,.F.) ;
#24537=ORIENTED_EDGE('',*,*,#17835,.F.) ;
#24538=ORIENTED_EDGE('',*,*,#17840,.T.) ;
#24539=ORIENTED_EDGE('',*,*,#17841,.T.) ;
#24540=ORIENTED_EDGE('',*,*,#17842,.T.) ;
#24541=ORIENTED_EDGE('',*,*,#17838,.F.) ;
#24542=ORIENTED_EDGE('',*,*,#17843,.T.) ;
#24543=ORIENTED_EDGE('',*,*,#17844,.T.) ;
#24544=ORIENTED_EDGE('',*,*,#17845,.F.) ;
#24545=ORIENTED_EDGE('',*,*,#17841,.F.) ;
#24546=ORIENTED_EDGE('',*,*,#17846,.T.) ;
#24547=ORIENTED_EDGE('',*,*,#17825,.F.) ;
#24548=ORIENTED_EDGE('',*,*,#17847,.T.) ;
#24549=ORIENTED_EDGE('',*,*,#17844,.F.) ;
#24550=ORIENTED_EDGE('',*,*,#17848,.F.) ;
#24551=ORIENTED_EDGE('',*,*,#17837,.T.) ;
#24552=ORIENTED_EDGE('',*,*,#17849,.F.) ;
#24553=ORIENTED_EDGE('',*,*,#17850,.F.) ;
#24554=ORIENTED_EDGE('',*,*,#17851,.F.) ;
#24555=ORIENTED_EDGE('',*,*,#17834,.F.) ;
#24556=ORIENTED_EDGE('',*,*,#17852,.T.) ;
#24557=ORIENTED_EDGE('',*,*,#17853,.T.) ;
#24558=ORIENTED_EDGE('',*,*,#17849,.T.) ;
#24559=ORIENTED_EDGE('',*,*,#17831,.F.) ;
#24560=ORIENTED_EDGE('',*,*,#17854,.F.) ;
#24561=ORIENTED_EDGE('',*,*,#17855,.F.) ;
#24562=ORIENTED_EDGE('',*,*,#17852,.F.) ;
#24563=ORIENTED_EDGE('',*,*,#17826,.F.) ;
#24564=ORIENTED_EDGE('',*,*,#17856,.T.) ;
#24565=ORIENTED_EDGE('',*,*,#17857,.T.) ;
#24566=ORIENTED_EDGE('',*,*,#17854,.T.) ;
#24567=ORIENTED_EDGE('',*,*,#17858,.T.) ;
#24568=ORIENTED_EDGE('',*,*,#17859,.T.) ;
#24569=ORIENTED_EDGE('',*,*,#17860,.T.) ;
#24570=ORIENTED_EDGE('',*,*,#17861,.F.) ;
#24571=ORIENTED_EDGE('',*,*,#17862,.T.) ;
#24572=ORIENTED_EDGE('',*,*,#17863,.T.) ;
#24573=ORIENTED_EDGE('',*,*,#17860,.F.) ;
#24574=ORIENTED_EDGE('',*,*,#17864,.T.) ;
#24575=ORIENTED_EDGE('',*,*,#17865,.T.) ;
#24576=ORIENTED_EDGE('',*,*,#17866,.F.) ;
#24577=ORIENTED_EDGE('',*,*,#17862,.F.) ;
#24578=ORIENTED_EDGE('',*,*,#17867,.T.) ;
#24579=ORIENTED_EDGE('',*,*,#17868,.T.) ;
#24580=ORIENTED_EDGE('',*,*,#17869,.T.) ;
#24581=ORIENTED_EDGE('',*,*,#17865,.F.) ;
#24582=ORIENTED_EDGE('',*,*,#17870,.F.) ;
#24583=ORIENTED_EDGE('',*,*,#17871,.T.) ;
#24584=ORIENTED_EDGE('',*,*,#17872,.F.) ;
#24585=ORIENTED_EDGE('',*,*,#17868,.F.) ;
#24586=ORIENTED_EDGE('',*,*,#17873,.T.) ;
#24587=ORIENTED_EDGE('',*,*,#17874,.T.) ;
#24588=ORIENTED_EDGE('',*,*,#17875,.T.) ;
#24589=ORIENTED_EDGE('',*,*,#17871,.F.) ;
#24590=ORIENTED_EDGE('',*,*,#17876,.T.) ;
#24591=ORIENTED_EDGE('',*,*,#17877,.T.) ;
#24592=ORIENTED_EDGE('',*,*,#17878,.F.) ;
#24593=ORIENTED_EDGE('',*,*,#17874,.F.) ;
#24594=ORIENTED_EDGE('',*,*,#17879,.T.) ;
#24595=ORIENTED_EDGE('',*,*,#17858,.F.) ;
#24596=ORIENTED_EDGE('',*,*,#17880,.T.) ;
#24597=ORIENTED_EDGE('',*,*,#17877,.F.) ;
#24598=ORIENTED_EDGE('',*,*,#17881,.F.) ;
#24599=ORIENTED_EDGE('',*,*,#17870,.T.) ;
#24600=ORIENTED_EDGE('',*,*,#17882,.F.) ;
#24601=ORIENTED_EDGE('',*,*,#17883,.F.) ;
#24602=ORIENTED_EDGE('',*,*,#17884,.F.) ;
#24603=ORIENTED_EDGE('',*,*,#17867,.F.) ;
#24604=ORIENTED_EDGE('',*,*,#17885,.T.) ;
#24605=ORIENTED_EDGE('',*,*,#17886,.T.) ;
#24606=ORIENTED_EDGE('',*,*,#17882,.T.) ;
#24607=ORIENTED_EDGE('',*,*,#17864,.F.) ;
#24608=ORIENTED_EDGE('',*,*,#17887,.F.) ;
#24609=ORIENTED_EDGE('',*,*,#17888,.F.) ;
#24610=ORIENTED_EDGE('',*,*,#17885,.F.) ;
#24611=ORIENTED_EDGE('',*,*,#17859,.F.) ;
#24612=ORIENTED_EDGE('',*,*,#17889,.T.) ;
#24613=ORIENTED_EDGE('',*,*,#17890,.T.) ;
#24614=ORIENTED_EDGE('',*,*,#17887,.T.) ;
#24615=ORIENTED_EDGE('',*,*,#17891,.T.) ;
#24616=ORIENTED_EDGE('',*,*,#17892,.T.) ;
#24617=ORIENTED_EDGE('',*,*,#17893,.T.) ;
#24618=ORIENTED_EDGE('',*,*,#17894,.F.) ;
#24619=ORIENTED_EDGE('',*,*,#17895,.T.) ;
#24620=ORIENTED_EDGE('',*,*,#17896,.T.) ;
#24621=ORIENTED_EDGE('',*,*,#17893,.F.) ;
#24622=ORIENTED_EDGE('',*,*,#17897,.T.) ;
#24623=ORIENTED_EDGE('',*,*,#17898,.T.) ;
#24624=ORIENTED_EDGE('',*,*,#17899,.F.) ;
#24625=ORIENTED_EDGE('',*,*,#17895,.F.) ;
#24626=ORIENTED_EDGE('',*,*,#17900,.T.) ;
#24627=ORIENTED_EDGE('',*,*,#17901,.T.) ;
#24628=ORIENTED_EDGE('',*,*,#17902,.T.) ;
#24629=ORIENTED_EDGE('',*,*,#17898,.F.) ;
#24630=ORIENTED_EDGE('',*,*,#17903,.F.) ;
#24631=ORIENTED_EDGE('',*,*,#17904,.T.) ;
#24632=ORIENTED_EDGE('',*,*,#17905,.F.) ;
#24633=ORIENTED_EDGE('',*,*,#17901,.F.) ;
#24634=ORIENTED_EDGE('',*,*,#17906,.T.) ;
#24635=ORIENTED_EDGE('',*,*,#17907,.T.) ;
#24636=ORIENTED_EDGE('',*,*,#17908,.T.) ;
#24637=ORIENTED_EDGE('',*,*,#17904,.F.) ;
#24638=ORIENTED_EDGE('',*,*,#17909,.T.) ;
#24639=ORIENTED_EDGE('',*,*,#17910,.T.) ;
#24640=ORIENTED_EDGE('',*,*,#17911,.F.) ;
#24641=ORIENTED_EDGE('',*,*,#17907,.F.) ;
#24642=ORIENTED_EDGE('',*,*,#17912,.T.) ;
#24643=ORIENTED_EDGE('',*,*,#17891,.F.) ;
#24644=ORIENTED_EDGE('',*,*,#17913,.T.) ;
#24645=ORIENTED_EDGE('',*,*,#17910,.F.) ;
#24646=ORIENTED_EDGE('',*,*,#17914,.F.) ;
#24647=ORIENTED_EDGE('',*,*,#17903,.T.) ;
#24648=ORIENTED_EDGE('',*,*,#17915,.F.) ;
#24649=ORIENTED_EDGE('',*,*,#17916,.F.) ;
#24650=ORIENTED_EDGE('',*,*,#17917,.F.) ;
#24651=ORIENTED_EDGE('',*,*,#17900,.F.) ;
#24652=ORIENTED_EDGE('',*,*,#17918,.T.) ;
#24653=ORIENTED_EDGE('',*,*,#17919,.T.) ;
#24654=ORIENTED_EDGE('',*,*,#17915,.T.) ;
#24655=ORIENTED_EDGE('',*,*,#17897,.F.) ;
#24656=ORIENTED_EDGE('',*,*,#17920,.F.) ;
#24657=ORIENTED_EDGE('',*,*,#17921,.F.) ;
#24658=ORIENTED_EDGE('',*,*,#17918,.F.) ;
#24659=ORIENTED_EDGE('',*,*,#17892,.F.) ;
#24660=ORIENTED_EDGE('',*,*,#17922,.T.) ;
#24661=ORIENTED_EDGE('',*,*,#17923,.T.) ;
#24662=ORIENTED_EDGE('',*,*,#17920,.T.) ;
#24663=ORIENTED_EDGE('',*,*,#17924,.T.) ;
#24664=ORIENTED_EDGE('',*,*,#17925,.T.) ;
#24665=ORIENTED_EDGE('',*,*,#17926,.T.) ;
#24666=ORIENTED_EDGE('',*,*,#17927,.F.) ;
#24667=ORIENTED_EDGE('',*,*,#17928,.T.) ;
#24668=ORIENTED_EDGE('',*,*,#17929,.T.) ;
#24669=ORIENTED_EDGE('',*,*,#17926,.F.) ;
#24670=ORIENTED_EDGE('',*,*,#17930,.T.) ;
#24671=ORIENTED_EDGE('',*,*,#17931,.T.) ;
#24672=ORIENTED_EDGE('',*,*,#17932,.F.) ;
#24673=ORIENTED_EDGE('',*,*,#17928,.F.) ;
#24674=ORIENTED_EDGE('',*,*,#17933,.T.) ;
#24675=ORIENTED_EDGE('',*,*,#17934,.T.) ;
#24676=ORIENTED_EDGE('',*,*,#17935,.T.) ;
#24677=ORIENTED_EDGE('',*,*,#17931,.F.) ;
#24678=ORIENTED_EDGE('',*,*,#17936,.F.) ;
#24679=ORIENTED_EDGE('',*,*,#17937,.T.) ;
#24680=ORIENTED_EDGE('',*,*,#17938,.F.) ;
#24681=ORIENTED_EDGE('',*,*,#17934,.F.) ;
#24682=ORIENTED_EDGE('',*,*,#17939,.T.) ;
#24683=ORIENTED_EDGE('',*,*,#17940,.T.) ;
#24684=ORIENTED_EDGE('',*,*,#17941,.T.) ;
#24685=ORIENTED_EDGE('',*,*,#17937,.F.) ;
#24686=ORIENTED_EDGE('',*,*,#17942,.T.) ;
#24687=ORIENTED_EDGE('',*,*,#17943,.T.) ;
#24688=ORIENTED_EDGE('',*,*,#17944,.F.) ;
#24689=ORIENTED_EDGE('',*,*,#17940,.F.) ;
#24690=ORIENTED_EDGE('',*,*,#17945,.T.) ;
#24691=ORIENTED_EDGE('',*,*,#17924,.F.) ;
#24692=ORIENTED_EDGE('',*,*,#17946,.T.) ;
#24693=ORIENTED_EDGE('',*,*,#17943,.F.) ;
#24694=ORIENTED_EDGE('',*,*,#17947,.F.) ;
#24695=ORIENTED_EDGE('',*,*,#17936,.T.) ;
#24696=ORIENTED_EDGE('',*,*,#17948,.F.) ;
#24697=ORIENTED_EDGE('',*,*,#17949,.F.) ;
#24698=ORIENTED_EDGE('',*,*,#17950,.F.) ;
#24699=ORIENTED_EDGE('',*,*,#17933,.F.) ;
#24700=ORIENTED_EDGE('',*,*,#17951,.T.) ;
#24701=ORIENTED_EDGE('',*,*,#17952,.T.) ;
#24702=ORIENTED_EDGE('',*,*,#17948,.T.) ;
#24703=ORIENTED_EDGE('',*,*,#17930,.F.) ;
#24704=ORIENTED_EDGE('',*,*,#17953,.F.) ;
#24705=ORIENTED_EDGE('',*,*,#17954,.F.) ;
#24706=ORIENTED_EDGE('',*,*,#17951,.F.) ;
#24707=ORIENTED_EDGE('',*,*,#17925,.F.) ;
#24708=ORIENTED_EDGE('',*,*,#17955,.T.) ;
#24709=ORIENTED_EDGE('',*,*,#17956,.T.) ;
#24710=ORIENTED_EDGE('',*,*,#17953,.T.) ;
#24711=ORIENTED_EDGE('',*,*,#17957,.T.) ;
#24712=ORIENTED_EDGE('',*,*,#17958,.T.) ;
#24713=ORIENTED_EDGE('',*,*,#17959,.T.) ;
#24714=ORIENTED_EDGE('',*,*,#17960,.F.) ;
#24715=ORIENTED_EDGE('',*,*,#17961,.T.) ;
#24716=ORIENTED_EDGE('',*,*,#17962,.T.) ;
#24717=ORIENTED_EDGE('',*,*,#17959,.F.) ;
#24718=ORIENTED_EDGE('',*,*,#17963,.T.) ;
#24719=ORIENTED_EDGE('',*,*,#17964,.T.) ;
#24720=ORIENTED_EDGE('',*,*,#17965,.F.) ;
#24721=ORIENTED_EDGE('',*,*,#17961,.F.) ;
#24722=ORIENTED_EDGE('',*,*,#17966,.T.) ;
#24723=ORIENTED_EDGE('',*,*,#17967,.T.) ;
#24724=ORIENTED_EDGE('',*,*,#17968,.T.) ;
#24725=ORIENTED_EDGE('',*,*,#17964,.F.) ;
#24726=ORIENTED_EDGE('',*,*,#17969,.F.) ;
#24727=ORIENTED_EDGE('',*,*,#17970,.T.) ;
#24728=ORIENTED_EDGE('',*,*,#17971,.F.) ;
#24729=ORIENTED_EDGE('',*,*,#17967,.F.) ;
#24730=ORIENTED_EDGE('',*,*,#17972,.T.) ;
#24731=ORIENTED_EDGE('',*,*,#17973,.T.) ;
#24732=ORIENTED_EDGE('',*,*,#17974,.T.) ;
#24733=ORIENTED_EDGE('',*,*,#17970,.F.) ;
#24734=ORIENTED_EDGE('',*,*,#17975,.T.) ;
#24735=ORIENTED_EDGE('',*,*,#17976,.T.) ;
#24736=ORIENTED_EDGE('',*,*,#17977,.F.) ;
#24737=ORIENTED_EDGE('',*,*,#17973,.F.) ;
#24738=ORIENTED_EDGE('',*,*,#17978,.T.) ;
#24739=ORIENTED_EDGE('',*,*,#17957,.F.) ;
#24740=ORIENTED_EDGE('',*,*,#17979,.T.) ;
#24741=ORIENTED_EDGE('',*,*,#17976,.F.) ;
#24742=ORIENTED_EDGE('',*,*,#17980,.F.) ;
#24743=ORIENTED_EDGE('',*,*,#17969,.T.) ;
#24744=ORIENTED_EDGE('',*,*,#17981,.F.) ;
#24745=ORIENTED_EDGE('',*,*,#17982,.F.) ;
#24746=ORIENTED_EDGE('',*,*,#17983,.F.) ;
#24747=ORIENTED_EDGE('',*,*,#17966,.F.) ;
#24748=ORIENTED_EDGE('',*,*,#17984,.T.) ;
#24749=ORIENTED_EDGE('',*,*,#17985,.T.) ;
#24750=ORIENTED_EDGE('',*,*,#17981,.T.) ;
#24751=ORIENTED_EDGE('',*,*,#17963,.F.) ;
#24752=ORIENTED_EDGE('',*,*,#17986,.F.) ;
#24753=ORIENTED_EDGE('',*,*,#17987,.F.) ;
#24754=ORIENTED_EDGE('',*,*,#17984,.F.) ;
#24755=ORIENTED_EDGE('',*,*,#17958,.F.) ;
#24756=ORIENTED_EDGE('',*,*,#17988,.T.) ;
#24757=ORIENTED_EDGE('',*,*,#17989,.T.) ;
#24758=ORIENTED_EDGE('',*,*,#17986,.T.) ;
#24759=ORIENTED_EDGE('',*,*,#17990,.T.) ;
#24760=ORIENTED_EDGE('',*,*,#17991,.T.) ;
#24761=ORIENTED_EDGE('',*,*,#17992,.T.) ;
#24762=ORIENTED_EDGE('',*,*,#17993,.F.) ;
#24763=ORIENTED_EDGE('',*,*,#17994,.T.) ;
#24764=ORIENTED_EDGE('',*,*,#17995,.T.) ;
#24765=ORIENTED_EDGE('',*,*,#17992,.F.) ;
#24766=ORIENTED_EDGE('',*,*,#17996,.T.) ;
#24767=ORIENTED_EDGE('',*,*,#17997,.T.) ;
#24768=ORIENTED_EDGE('',*,*,#17998,.F.) ;
#24769=ORIENTED_EDGE('',*,*,#17994,.F.) ;
#24770=ORIENTED_EDGE('',*,*,#17999,.T.) ;
#24771=ORIENTED_EDGE('',*,*,#18000,.T.) ;
#24772=ORIENTED_EDGE('',*,*,#18001,.T.) ;
#24773=ORIENTED_EDGE('',*,*,#17997,.F.) ;
#24774=ORIENTED_EDGE('',*,*,#18002,.F.) ;
#24775=ORIENTED_EDGE('',*,*,#18003,.T.) ;
#24776=ORIENTED_EDGE('',*,*,#18004,.F.) ;
#24777=ORIENTED_EDGE('',*,*,#18000,.F.) ;
#24778=ORIENTED_EDGE('',*,*,#18005,.T.) ;
#24779=ORIENTED_EDGE('',*,*,#18006,.T.) ;
#24780=ORIENTED_EDGE('',*,*,#18007,.T.) ;
#24781=ORIENTED_EDGE('',*,*,#18003,.F.) ;
#24782=ORIENTED_EDGE('',*,*,#18008,.T.) ;
#24783=ORIENTED_EDGE('',*,*,#18009,.T.) ;
#24784=ORIENTED_EDGE('',*,*,#18010,.F.) ;
#24785=ORIENTED_EDGE('',*,*,#18006,.F.) ;
#24786=ORIENTED_EDGE('',*,*,#17470,.T.) ;
#24787=ORIENTED_EDGE('',*,*,#17990,.F.) ;
#24788=ORIENTED_EDGE('',*,*,#18011,.T.) ;
#24789=ORIENTED_EDGE('',*,*,#18009,.F.) ;
#24790=ORIENTED_EDGE('',*,*,#18012,.F.) ;
#24791=ORIENTED_EDGE('',*,*,#18002,.T.) ;
#24792=ORIENTED_EDGE('',*,*,#18013,.F.) ;
#24793=ORIENTED_EDGE('',*,*,#18014,.T.) ;
#24794=ORIENTED_EDGE('',*,*,#18015,.T.) ;
#24795=ORIENTED_EDGE('',*,*,#17461,.F.) ;
#24796=ORIENTED_EDGE('',*,*,#18016,.T.) ;
#24797=ORIENTED_EDGE('',*,*,#18017,.T.) ;
#24798=ORIENTED_EDGE('',*,*,#18018,.T.) ;
#24799=ORIENTED_EDGE('',*,*,#18013,.T.) ;
#24800=ORIENTED_EDGE('',*,*,#17999,.F.) ;
#24801=ORIENTED_EDGE('',*,*,#18019,.T.) ;
#24802=ORIENTED_EDGE('',*,*,#18020,.T.) ;
#24803=ORIENTED_EDGE('',*,*,#18021,.T.) ;
#24804=ORIENTED_EDGE('',*,*,#18022,.T.) ;
#24805=ORIENTED_EDGE('',*,*,#17996,.F.) ;
#24806=ORIENTED_EDGE('',*,*,#18023,.F.) ;
#24807=ORIENTED_EDGE('',*,*,#18024,.T.) ;
#24808=ORIENTED_EDGE('',*,*,#18019,.F.) ;
#24809=ORIENTED_EDGE('',*,*,#17991,.F.) ;
#24810=ORIENTED_EDGE('',*,*,#18025,.T.) ;
#24811=ORIENTED_EDGE('',*,*,#18026,.T.) ;
#24812=ORIENTED_EDGE('',*,*,#18023,.T.) ;
#24813=ORIENTED_EDGE('',*,*,#18027,.T.) ;
#24814=ORIENTED_EDGE('',*,*,#18028,.T.) ;
#24815=ORIENTED_EDGE('',*,*,#18029,.T.) ;
#24816=ORIENTED_EDGE('',*,*,#18030,.F.) ;
#24817=ORIENTED_EDGE('',*,*,#18031,.T.) ;
#24818=ORIENTED_EDGE('',*,*,#18032,.T.) ;
#24819=ORIENTED_EDGE('',*,*,#18029,.F.) ;
#24820=ORIENTED_EDGE('',*,*,#18033,.T.) ;
#24821=ORIENTED_EDGE('',*,*,#18034,.T.) ;
#24822=ORIENTED_EDGE('',*,*,#18035,.F.) ;
#24823=ORIENTED_EDGE('',*,*,#18031,.F.) ;
#24824=ORIENTED_EDGE('',*,*,#18036,.T.) ;
#24825=ORIENTED_EDGE('',*,*,#18037,.T.) ;
#24826=ORIENTED_EDGE('',*,*,#18038,.T.) ;
#24827=ORIENTED_EDGE('',*,*,#18034,.F.) ;
#24828=ORIENTED_EDGE('',*,*,#18039,.F.) ;
#24829=ORIENTED_EDGE('',*,*,#18040,.T.) ;
#24830=ORIENTED_EDGE('',*,*,#18041,.F.) ;
#24831=ORIENTED_EDGE('',*,*,#18037,.F.) ;
#24832=ORIENTED_EDGE('',*,*,#18042,.T.) ;
#24833=ORIENTED_EDGE('',*,*,#18043,.T.) ;
#24834=ORIENTED_EDGE('',*,*,#18044,.T.) ;
#24835=ORIENTED_EDGE('',*,*,#18040,.F.) ;
#24836=ORIENTED_EDGE('',*,*,#18045,.T.) ;
#24837=ORIENTED_EDGE('',*,*,#18046,.T.) ;
#24838=ORIENTED_EDGE('',*,*,#18047,.F.) ;
#24839=ORIENTED_EDGE('',*,*,#18043,.F.) ;
#24840=ORIENTED_EDGE('',*,*,#17501,.T.) ;
#24841=ORIENTED_EDGE('',*,*,#18027,.F.) ;
#24842=ORIENTED_EDGE('',*,*,#18048,.T.) ;
#24843=ORIENTED_EDGE('',*,*,#18046,.F.) ;
#24844=ORIENTED_EDGE('',*,*,#18049,.F.) ;
#24845=ORIENTED_EDGE('',*,*,#18039,.T.) ;
#24846=ORIENTED_EDGE('',*,*,#18050,.F.) ;
#24847=ORIENTED_EDGE('',*,*,#18051,.T.) ;
#24848=ORIENTED_EDGE('',*,*,#18052,.T.) ;
#24849=ORIENTED_EDGE('',*,*,#17492,.F.) ;
#24850=ORIENTED_EDGE('',*,*,#18053,.T.) ;
#24851=ORIENTED_EDGE('',*,*,#18054,.T.) ;
#24852=ORIENTED_EDGE('',*,*,#18055,.T.) ;
#24853=ORIENTED_EDGE('',*,*,#18050,.T.) ;
#24854=ORIENTED_EDGE('',*,*,#18036,.F.) ;
#24855=ORIENTED_EDGE('',*,*,#18056,.T.) ;
#24856=ORIENTED_EDGE('',*,*,#18057,.T.) ;
#24857=ORIENTED_EDGE('',*,*,#18058,.T.) ;
#24858=ORIENTED_EDGE('',*,*,#18059,.T.) ;
#24859=ORIENTED_EDGE('',*,*,#18033,.F.) ;
#24860=ORIENTED_EDGE('',*,*,#18060,.F.) ;
#24861=ORIENTED_EDGE('',*,*,#18061,.T.) ;
#24862=ORIENTED_EDGE('',*,*,#18056,.F.) ;
#24863=ORIENTED_EDGE('',*,*,#18028,.F.) ;
#24864=ORIENTED_EDGE('',*,*,#18062,.T.) ;
#24865=ORIENTED_EDGE('',*,*,#18063,.T.) ;
#24866=ORIENTED_EDGE('',*,*,#18060,.T.) ;
#24867=ORIENTED_EDGE('',*,*,#18064,.T.) ;
#24868=ORIENTED_EDGE('',*,*,#18065,.T.) ;
#24869=ORIENTED_EDGE('',*,*,#18066,.T.) ;
#24870=ORIENTED_EDGE('',*,*,#18067,.F.) ;
#24871=ORIENTED_EDGE('',*,*,#18068,.T.) ;
#24872=ORIENTED_EDGE('',*,*,#18069,.T.) ;
#24873=ORIENTED_EDGE('',*,*,#18066,.F.) ;
#24874=ORIENTED_EDGE('',*,*,#18070,.T.) ;
#24875=ORIENTED_EDGE('',*,*,#18071,.T.) ;
#24876=ORIENTED_EDGE('',*,*,#18072,.F.) ;
#24877=ORIENTED_EDGE('',*,*,#18068,.F.) ;
#24878=ORIENTED_EDGE('',*,*,#18073,.T.) ;
#24879=ORIENTED_EDGE('',*,*,#18074,.T.) ;
#24880=ORIENTED_EDGE('',*,*,#18075,.T.) ;
#24881=ORIENTED_EDGE('',*,*,#18071,.F.) ;
#24882=ORIENTED_EDGE('',*,*,#18076,.F.) ;
#24883=ORIENTED_EDGE('',*,*,#18077,.T.) ;
#24884=ORIENTED_EDGE('',*,*,#18078,.F.) ;
#24885=ORIENTED_EDGE('',*,*,#18074,.F.) ;
#24886=ORIENTED_EDGE('',*,*,#18079,.T.) ;
#24887=ORIENTED_EDGE('',*,*,#18080,.T.) ;
#24888=ORIENTED_EDGE('',*,*,#18081,.T.) ;
#24889=ORIENTED_EDGE('',*,*,#18077,.F.) ;
#24890=ORIENTED_EDGE('',*,*,#18082,.T.) ;
#24891=ORIENTED_EDGE('',*,*,#18083,.T.) ;
#24892=ORIENTED_EDGE('',*,*,#18084,.F.) ;
#24893=ORIENTED_EDGE('',*,*,#18080,.F.) ;
#24894=ORIENTED_EDGE('',*,*,#17532,.T.) ;
#24895=ORIENTED_EDGE('',*,*,#18064,.F.) ;
#24896=ORIENTED_EDGE('',*,*,#18085,.T.) ;
#24897=ORIENTED_EDGE('',*,*,#18083,.F.) ;
#24898=ORIENTED_EDGE('',*,*,#18086,.F.) ;
#24899=ORIENTED_EDGE('',*,*,#18076,.T.) ;
#24900=ORIENTED_EDGE('',*,*,#18087,.F.) ;
#24901=ORIENTED_EDGE('',*,*,#18088,.T.) ;
#24902=ORIENTED_EDGE('',*,*,#18089,.T.) ;
#24903=ORIENTED_EDGE('',*,*,#17523,.F.) ;
#24904=ORIENTED_EDGE('',*,*,#18090,.T.) ;
#24905=ORIENTED_EDGE('',*,*,#18091,.T.) ;
#24906=ORIENTED_EDGE('',*,*,#18092,.T.) ;
#24907=ORIENTED_EDGE('',*,*,#18087,.T.) ;
#24908=ORIENTED_EDGE('',*,*,#18073,.F.) ;
#24909=ORIENTED_EDGE('',*,*,#18093,.T.) ;
#24910=ORIENTED_EDGE('',*,*,#18094,.T.) ;
#24911=ORIENTED_EDGE('',*,*,#18095,.T.) ;
#24912=ORIENTED_EDGE('',*,*,#18096,.T.) ;
#24913=ORIENTED_EDGE('',*,*,#18070,.F.) ;
#24914=ORIENTED_EDGE('',*,*,#18097,.F.) ;
#24915=ORIENTED_EDGE('',*,*,#18098,.T.) ;
#24916=ORIENTED_EDGE('',*,*,#18093,.F.) ;
#24917=ORIENTED_EDGE('',*,*,#18065,.F.) ;
#24918=ORIENTED_EDGE('',*,*,#18099,.T.) ;
#24919=ORIENTED_EDGE('',*,*,#18100,.T.) ;
#24920=ORIENTED_EDGE('',*,*,#18097,.T.) ;
#24921=ORIENTED_EDGE('',*,*,#18101,.T.) ;
#24922=ORIENTED_EDGE('',*,*,#18102,.T.) ;
#24923=ORIENTED_EDGE('',*,*,#18103,.T.) ;
#24924=ORIENTED_EDGE('',*,*,#18104,.F.) ;
#24925=ORIENTED_EDGE('',*,*,#18105,.T.) ;
#24926=ORIENTED_EDGE('',*,*,#18106,.T.) ;
#24927=ORIENTED_EDGE('',*,*,#18103,.F.) ;
#24928=ORIENTED_EDGE('',*,*,#18107,.T.) ;
#24929=ORIENTED_EDGE('',*,*,#18108,.T.) ;
#24930=ORIENTED_EDGE('',*,*,#18109,.F.) ;
#24931=ORIENTED_EDGE('',*,*,#18105,.F.) ;
#24932=ORIENTED_EDGE('',*,*,#18110,.T.) ;
#24933=ORIENTED_EDGE('',*,*,#18111,.T.) ;
#24934=ORIENTED_EDGE('',*,*,#18112,.T.) ;
#24935=ORIENTED_EDGE('',*,*,#18108,.F.) ;
#24936=ORIENTED_EDGE('',*,*,#18113,.F.) ;
#24937=ORIENTED_EDGE('',*,*,#18114,.T.) ;
#24938=ORIENTED_EDGE('',*,*,#18115,.F.) ;
#24939=ORIENTED_EDGE('',*,*,#18111,.F.) ;
#24940=ORIENTED_EDGE('',*,*,#18116,.T.) ;
#24941=ORIENTED_EDGE('',*,*,#18117,.T.) ;
#24942=ORIENTED_EDGE('',*,*,#18118,.T.) ;
#24943=ORIENTED_EDGE('',*,*,#18114,.F.) ;
#24944=ORIENTED_EDGE('',*,*,#18119,.T.) ;
#24945=ORIENTED_EDGE('',*,*,#18120,.T.) ;
#24946=ORIENTED_EDGE('',*,*,#18121,.F.) ;
#24947=ORIENTED_EDGE('',*,*,#18117,.F.) ;
#24948=ORIENTED_EDGE('',*,*,#17563,.T.) ;
#24949=ORIENTED_EDGE('',*,*,#18101,.F.) ;
#24950=ORIENTED_EDGE('',*,*,#18122,.T.) ;
#24951=ORIENTED_EDGE('',*,*,#18120,.F.) ;
#24952=ORIENTED_EDGE('',*,*,#18123,.F.) ;
#24953=ORIENTED_EDGE('',*,*,#18113,.T.) ;
#24954=ORIENTED_EDGE('',*,*,#18124,.F.) ;
#24955=ORIENTED_EDGE('',*,*,#18125,.T.) ;
#24956=ORIENTED_EDGE('',*,*,#18126,.T.) ;
#24957=ORIENTED_EDGE('',*,*,#17554,.F.) ;
#24958=ORIENTED_EDGE('',*,*,#18127,.T.) ;
#24959=ORIENTED_EDGE('',*,*,#18128,.T.) ;
#24960=ORIENTED_EDGE('',*,*,#18129,.T.) ;
#24961=ORIENTED_EDGE('',*,*,#18124,.T.) ;
#24962=ORIENTED_EDGE('',*,*,#18110,.F.) ;
#24963=ORIENTED_EDGE('',*,*,#18130,.T.) ;
#24964=ORIENTED_EDGE('',*,*,#18131,.T.) ;
#24965=ORIENTED_EDGE('',*,*,#18132,.T.) ;
#24966=ORIENTED_EDGE('',*,*,#18133,.T.) ;
#24967=ORIENTED_EDGE('',*,*,#18107,.F.) ;
#24968=ORIENTED_EDGE('',*,*,#18134,.F.) ;
#24969=ORIENTED_EDGE('',*,*,#18135,.T.) ;
#24970=ORIENTED_EDGE('',*,*,#18130,.F.) ;
#24971=ORIENTED_EDGE('',*,*,#18102,.F.) ;
#24972=ORIENTED_EDGE('',*,*,#18136,.T.) ;
#24973=ORIENTED_EDGE('',*,*,#18137,.T.) ;
#24974=ORIENTED_EDGE('',*,*,#18134,.T.) ;
#24975=ORIENTED_EDGE('',*,*,#18138,.T.) ;
#24976=ORIENTED_EDGE('',*,*,#18139,.T.) ;
#24977=ORIENTED_EDGE('',*,*,#18140,.T.) ;
#24978=ORIENTED_EDGE('',*,*,#18141,.F.) ;
#24979=ORIENTED_EDGE('',*,*,#18142,.T.) ;
#24980=ORIENTED_EDGE('',*,*,#18143,.T.) ;
#24981=ORIENTED_EDGE('',*,*,#18140,.F.) ;
#24982=ORIENTED_EDGE('',*,*,#18144,.T.) ;
#24983=ORIENTED_EDGE('',*,*,#18145,.T.) ;
#24984=ORIENTED_EDGE('',*,*,#18146,.F.) ;
#24985=ORIENTED_EDGE('',*,*,#18142,.F.) ;
#24986=ORIENTED_EDGE('',*,*,#18147,.T.) ;
#24987=ORIENTED_EDGE('',*,*,#18148,.T.) ;
#24988=ORIENTED_EDGE('',*,*,#18149,.T.) ;
#24989=ORIENTED_EDGE('',*,*,#18145,.F.) ;
#24990=ORIENTED_EDGE('',*,*,#18150,.F.) ;
#24991=ORIENTED_EDGE('',*,*,#18151,.T.) ;
#24992=ORIENTED_EDGE('',*,*,#18152,.F.) ;
#24993=ORIENTED_EDGE('',*,*,#18148,.F.) ;
#24994=ORIENTED_EDGE('',*,*,#18153,.T.) ;
#24995=ORIENTED_EDGE('',*,*,#18154,.T.) ;
#24996=ORIENTED_EDGE('',*,*,#18155,.T.) ;
#24997=ORIENTED_EDGE('',*,*,#18151,.F.) ;
#24998=ORIENTED_EDGE('',*,*,#18156,.T.) ;
#24999=ORIENTED_EDGE('',*,*,#18157,.T.) ;
#25000=ORIENTED_EDGE('',*,*,#18158,.F.) ;
#25001=ORIENTED_EDGE('',*,*,#18154,.F.) ;
#25002=ORIENTED_EDGE('',*,*,#17594,.T.) ;
#25003=ORIENTED_EDGE('',*,*,#18138,.F.) ;
#25004=ORIENTED_EDGE('',*,*,#18159,.T.) ;
#25005=ORIENTED_EDGE('',*,*,#18157,.F.) ;
#25006=ORIENTED_EDGE('',*,*,#18160,.F.) ;
#25007=ORIENTED_EDGE('',*,*,#18150,.T.) ;
#25008=ORIENTED_EDGE('',*,*,#18161,.F.) ;
#25009=ORIENTED_EDGE('',*,*,#18162,.T.) ;
#25010=ORIENTED_EDGE('',*,*,#18163,.T.) ;
#25011=ORIENTED_EDGE('',*,*,#17585,.F.) ;
#25012=ORIENTED_EDGE('',*,*,#18164,.T.) ;
#25013=ORIENTED_EDGE('',*,*,#18165,.T.) ;
#25014=ORIENTED_EDGE('',*,*,#18166,.T.) ;
#25015=ORIENTED_EDGE('',*,*,#18161,.T.) ;
#25016=ORIENTED_EDGE('',*,*,#18147,.F.) ;
#25017=ORIENTED_EDGE('',*,*,#18167,.T.) ;
#25018=ORIENTED_EDGE('',*,*,#18168,.T.) ;
#25019=ORIENTED_EDGE('',*,*,#18169,.T.) ;
#25020=ORIENTED_EDGE('',*,*,#18170,.T.) ;
#25021=ORIENTED_EDGE('',*,*,#18144,.F.) ;
#25022=ORIENTED_EDGE('',*,*,#18171,.F.) ;
#25023=ORIENTED_EDGE('',*,*,#18172,.T.) ;
#25024=ORIENTED_EDGE('',*,*,#18167,.F.) ;
#25025=ORIENTED_EDGE('',*,*,#18139,.F.) ;
#25026=ORIENTED_EDGE('',*,*,#18173,.T.) ;
#25027=ORIENTED_EDGE('',*,*,#18174,.T.) ;
#25028=ORIENTED_EDGE('',*,*,#18171,.T.) ;
#25029=ORIENTED_EDGE('',*,*,#18175,.T.) ;
#25030=ORIENTED_EDGE('',*,*,#18176,.T.) ;
#25031=ORIENTED_EDGE('',*,*,#18177,.T.) ;
#25032=ORIENTED_EDGE('',*,*,#18178,.F.) ;
#25033=ORIENTED_EDGE('',*,*,#18179,.T.) ;
#25034=ORIENTED_EDGE('',*,*,#18180,.T.) ;
#25035=ORIENTED_EDGE('',*,*,#18177,.F.) ;
#25036=ORIENTED_EDGE('',*,*,#18181,.T.) ;
#25037=ORIENTED_EDGE('',*,*,#18182,.T.) ;
#25038=ORIENTED_EDGE('',*,*,#18183,.F.) ;
#25039=ORIENTED_EDGE('',*,*,#18179,.F.) ;
#25040=ORIENTED_EDGE('',*,*,#18184,.T.) ;
#25041=ORIENTED_EDGE('',*,*,#18185,.T.) ;
#25042=ORIENTED_EDGE('',*,*,#18186,.T.) ;
#25043=ORIENTED_EDGE('',*,*,#18182,.F.) ;
#25044=ORIENTED_EDGE('',*,*,#18187,.F.) ;
#25045=ORIENTED_EDGE('',*,*,#18188,.T.) ;
#25046=ORIENTED_EDGE('',*,*,#18189,.F.) ;
#25047=ORIENTED_EDGE('',*,*,#18185,.F.) ;
#25048=ORIENTED_EDGE('',*,*,#18190,.T.) ;
#25049=ORIENTED_EDGE('',*,*,#18191,.T.) ;
#25050=ORIENTED_EDGE('',*,*,#18192,.T.) ;
#25051=ORIENTED_EDGE('',*,*,#18188,.F.) ;
#25052=ORIENTED_EDGE('',*,*,#18193,.T.) ;
#25053=ORIENTED_EDGE('',*,*,#18194,.T.) ;
#25054=ORIENTED_EDGE('',*,*,#18195,.F.) ;
#25055=ORIENTED_EDGE('',*,*,#18191,.F.) ;
#25056=ORIENTED_EDGE('',*,*,#17625,.T.) ;
#25057=ORIENTED_EDGE('',*,*,#18175,.F.) ;
#25058=ORIENTED_EDGE('',*,*,#18196,.T.) ;
#25059=ORIENTED_EDGE('',*,*,#18194,.F.) ;
#25060=ORIENTED_EDGE('',*,*,#18197,.F.) ;
#25061=ORIENTED_EDGE('',*,*,#18187,.T.) ;
#25062=ORIENTED_EDGE('',*,*,#18198,.F.) ;
#25063=ORIENTED_EDGE('',*,*,#18199,.T.) ;
#25064=ORIENTED_EDGE('',*,*,#18200,.T.) ;
#25065=ORIENTED_EDGE('',*,*,#17616,.F.) ;
#25066=ORIENTED_EDGE('',*,*,#18201,.T.) ;
#25067=ORIENTED_EDGE('',*,*,#18202,.T.) ;
#25068=ORIENTED_EDGE('',*,*,#18203,.T.) ;
#25069=ORIENTED_EDGE('',*,*,#18198,.T.) ;
#25070=ORIENTED_EDGE('',*,*,#18184,.F.) ;
#25071=ORIENTED_EDGE('',*,*,#18204,.T.) ;
#25072=ORIENTED_EDGE('',*,*,#18205,.T.) ;
#25073=ORIENTED_EDGE('',*,*,#18206,.T.) ;
#25074=ORIENTED_EDGE('',*,*,#18207,.T.) ;
#25075=ORIENTED_EDGE('',*,*,#18181,.F.) ;
#25076=ORIENTED_EDGE('',*,*,#18208,.F.) ;
#25077=ORIENTED_EDGE('',*,*,#18209,.T.) ;
#25078=ORIENTED_EDGE('',*,*,#18204,.F.) ;
#25079=ORIENTED_EDGE('',*,*,#18176,.F.) ;
#25080=ORIENTED_EDGE('',*,*,#18210,.T.) ;
#25081=ORIENTED_EDGE('',*,*,#18211,.T.) ;
#25082=ORIENTED_EDGE('',*,*,#18208,.T.) ;
#25083=ORIENTED_EDGE('',*,*,#18212,.T.) ;
#25084=ORIENTED_EDGE('',*,*,#18213,.T.) ;
#25085=ORIENTED_EDGE('',*,*,#18214,.T.) ;
#25086=ORIENTED_EDGE('',*,*,#18215,.F.) ;
#25087=ORIENTED_EDGE('',*,*,#18216,.T.) ;
#25088=ORIENTED_EDGE('',*,*,#18217,.T.) ;
#25089=ORIENTED_EDGE('',*,*,#18214,.F.) ;
#25090=ORIENTED_EDGE('',*,*,#18218,.T.) ;
#25091=ORIENTED_EDGE('',*,*,#18219,.T.) ;
#25092=ORIENTED_EDGE('',*,*,#18220,.F.) ;
#25093=ORIENTED_EDGE('',*,*,#18216,.F.) ;
#25094=ORIENTED_EDGE('',*,*,#18221,.T.) ;
#25095=ORIENTED_EDGE('',*,*,#18222,.T.) ;
#25096=ORIENTED_EDGE('',*,*,#18223,.T.) ;
#25097=ORIENTED_EDGE('',*,*,#18219,.F.) ;
#25098=ORIENTED_EDGE('',*,*,#18224,.F.) ;
#25099=ORIENTED_EDGE('',*,*,#18225,.T.) ;
#25100=ORIENTED_EDGE('',*,*,#18226,.F.) ;
#25101=ORIENTED_EDGE('',*,*,#18222,.F.) ;
#25102=ORIENTED_EDGE('',*,*,#18227,.T.) ;
#25103=ORIENTED_EDGE('',*,*,#18228,.T.) ;
#25104=ORIENTED_EDGE('',*,*,#18229,.T.) ;
#25105=ORIENTED_EDGE('',*,*,#18225,.F.) ;
#25106=ORIENTED_EDGE('',*,*,#18230,.T.) ;
#25107=ORIENTED_EDGE('',*,*,#18231,.T.) ;
#25108=ORIENTED_EDGE('',*,*,#18232,.F.) ;
#25109=ORIENTED_EDGE('',*,*,#18228,.F.) ;
#25110=ORIENTED_EDGE('',*,*,#17656,.T.) ;
#25111=ORIENTED_EDGE('',*,*,#18212,.F.) ;
#25112=ORIENTED_EDGE('',*,*,#18233,.T.) ;
#25113=ORIENTED_EDGE('',*,*,#18231,.F.) ;
#25114=ORIENTED_EDGE('',*,*,#18234,.F.) ;
#25115=ORIENTED_EDGE('',*,*,#18224,.T.) ;
#25116=ORIENTED_EDGE('',*,*,#18235,.F.) ;
#25117=ORIENTED_EDGE('',*,*,#18236,.T.) ;
#25118=ORIENTED_EDGE('',*,*,#18237,.T.) ;
#25119=ORIENTED_EDGE('',*,*,#17647,.F.) ;
#25120=ORIENTED_EDGE('',*,*,#18238,.T.) ;
#25121=ORIENTED_EDGE('',*,*,#18239,.T.) ;
#25122=ORIENTED_EDGE('',*,*,#18240,.T.) ;
#25123=ORIENTED_EDGE('',*,*,#18235,.T.) ;
#25124=ORIENTED_EDGE('',*,*,#18221,.F.) ;
#25125=ORIENTED_EDGE('',*,*,#18241,.T.) ;
#25126=ORIENTED_EDGE('',*,*,#18242,.T.) ;
#25127=ORIENTED_EDGE('',*,*,#18243,.T.) ;
#25128=ORIENTED_EDGE('',*,*,#18244,.T.) ;
#25129=ORIENTED_EDGE('',*,*,#18218,.F.) ;
#25130=ORIENTED_EDGE('',*,*,#18245,.F.) ;
#25131=ORIENTED_EDGE('',*,*,#18246,.T.) ;
#25132=ORIENTED_EDGE('',*,*,#18241,.F.) ;
#25133=ORIENTED_EDGE('',*,*,#18213,.F.) ;
#25134=ORIENTED_EDGE('',*,*,#18247,.T.) ;
#25135=ORIENTED_EDGE('',*,*,#18248,.T.) ;
#25136=ORIENTED_EDGE('',*,*,#18245,.T.) ;
#25137=ORIENTED_EDGE('',*,*,#18249,.T.) ;
#25138=ORIENTED_EDGE('',*,*,#18250,.T.) ;
#25139=ORIENTED_EDGE('',*,*,#18251,.T.) ;
#25140=ORIENTED_EDGE('',*,*,#18252,.F.) ;
#25141=ORIENTED_EDGE('',*,*,#18253,.T.) ;
#25142=ORIENTED_EDGE('',*,*,#18254,.T.) ;
#25143=ORIENTED_EDGE('',*,*,#18251,.F.) ;
#25144=ORIENTED_EDGE('',*,*,#18255,.T.) ;
#25145=ORIENTED_EDGE('',*,*,#18256,.T.) ;
#25146=ORIENTED_EDGE('',*,*,#18257,.F.) ;
#25147=ORIENTED_EDGE('',*,*,#18253,.F.) ;
#25148=ORIENTED_EDGE('',*,*,#18258,.T.) ;
#25149=ORIENTED_EDGE('',*,*,#18259,.T.) ;
#25150=ORIENTED_EDGE('',*,*,#18260,.T.) ;
#25151=ORIENTED_EDGE('',*,*,#18256,.F.) ;
#25152=ORIENTED_EDGE('',*,*,#18261,.F.) ;
#25153=ORIENTED_EDGE('',*,*,#18262,.T.) ;
#25154=ORIENTED_EDGE('',*,*,#18263,.F.) ;
#25155=ORIENTED_EDGE('',*,*,#18259,.F.) ;
#25156=ORIENTED_EDGE('',*,*,#18264,.T.) ;
#25157=ORIENTED_EDGE('',*,*,#18265,.T.) ;
#25158=ORIENTED_EDGE('',*,*,#18266,.T.) ;
#25159=ORIENTED_EDGE('',*,*,#18262,.F.) ;
#25160=ORIENTED_EDGE('',*,*,#18267,.T.) ;
#25161=ORIENTED_EDGE('',*,*,#18268,.T.) ;
#25162=ORIENTED_EDGE('',*,*,#18269,.F.) ;
#25163=ORIENTED_EDGE('',*,*,#18265,.F.) ;
#25164=ORIENTED_EDGE('',*,*,#17687,.T.) ;
#25165=ORIENTED_EDGE('',*,*,#18249,.F.) ;
#25166=ORIENTED_EDGE('',*,*,#18270,.T.) ;
#25167=ORIENTED_EDGE('',*,*,#18268,.F.) ;
#25168=ORIENTED_EDGE('',*,*,#18271,.F.) ;
#25169=ORIENTED_EDGE('',*,*,#18261,.T.) ;
#25170=ORIENTED_EDGE('',*,*,#18272,.F.) ;
#25171=ORIENTED_EDGE('',*,*,#18273,.T.) ;
#25172=ORIENTED_EDGE('',*,*,#18274,.T.) ;
#25173=ORIENTED_EDGE('',*,*,#17678,.F.) ;
#25174=ORIENTED_EDGE('',*,*,#18275,.T.) ;
#25175=ORIENTED_EDGE('',*,*,#18276,.T.) ;
#25176=ORIENTED_EDGE('',*,*,#18277,.T.) ;
#25177=ORIENTED_EDGE('',*,*,#18272,.T.) ;
#25178=ORIENTED_EDGE('',*,*,#18258,.F.) ;
#25179=ORIENTED_EDGE('',*,*,#18278,.T.) ;
#25180=ORIENTED_EDGE('',*,*,#18279,.T.) ;
#25181=ORIENTED_EDGE('',*,*,#18280,.T.) ;
#25182=ORIENTED_EDGE('',*,*,#18281,.T.) ;
#25183=ORIENTED_EDGE('',*,*,#18255,.F.) ;
#25184=ORIENTED_EDGE('',*,*,#18282,.F.) ;
#25185=ORIENTED_EDGE('',*,*,#18283,.T.) ;
#25186=ORIENTED_EDGE('',*,*,#18278,.F.) ;
#25187=ORIENTED_EDGE('',*,*,#18250,.F.) ;
#25188=ORIENTED_EDGE('',*,*,#18284,.T.) ;
#25189=ORIENTED_EDGE('',*,*,#18285,.T.) ;
#25190=ORIENTED_EDGE('',*,*,#18282,.T.) ;
#25191=ORIENTED_EDGE('',*,*,#18286,.T.) ;
#25192=ORIENTED_EDGE('',*,*,#18287,.T.) ;
#25193=ORIENTED_EDGE('',*,*,#18288,.T.) ;
#25194=ORIENTED_EDGE('',*,*,#18289,.T.) ;
#25195=ORIENTED_EDGE('',*,*,#18290,.T.) ;
#25196=ORIENTED_EDGE('',*,*,#18291,.T.) ;
#25197=ORIENTED_EDGE('',*,*,#18288,.F.) ;
#25198=ORIENTED_EDGE('',*,*,#18292,.T.) ;
#25199=ORIENTED_EDGE('',*,*,#18293,.T.) ;
#25200=ORIENTED_EDGE('',*,*,#18294,.T.) ;
#25201=ORIENTED_EDGE('',*,*,#18290,.F.) ;
#25202=ORIENTED_EDGE('',*,*,#18295,.T.) ;
#25203=ORIENTED_EDGE('',*,*,#18296,.T.) ;
#25204=ORIENTED_EDGE('',*,*,#18297,.T.) ;
#25205=ORIENTED_EDGE('',*,*,#18293,.F.) ;
#25206=ORIENTED_EDGE('',*,*,#18298,.T.) ;
#25207=ORIENTED_EDGE('',*,*,#18299,.T.) ;
#25208=ORIENTED_EDGE('',*,*,#18300,.T.) ;
#25209=ORIENTED_EDGE('',*,*,#18296,.F.) ;
#25210=ORIENTED_EDGE('',*,*,#18301,.T.) ;
#25211=ORIENTED_EDGE('',*,*,#18302,.T.) ;
#25212=ORIENTED_EDGE('',*,*,#18303,.T.) ;
#25213=ORIENTED_EDGE('',*,*,#18299,.F.) ;
#25214=ORIENTED_EDGE('',*,*,#18304,.T.) ;
#25215=ORIENTED_EDGE('',*,*,#18305,.T.) ;
#25216=ORIENTED_EDGE('',*,*,#18306,.T.) ;
#25217=ORIENTED_EDGE('',*,*,#18302,.F.) ;
#25218=ORIENTED_EDGE('',*,*,#18307,.T.) ;
#25219=ORIENTED_EDGE('',*,*,#18286,.F.) ;
#25220=ORIENTED_EDGE('',*,*,#18308,.T.) ;
#25221=ORIENTED_EDGE('',*,*,#18305,.F.) ;
#25222=ORIENTED_EDGE('',*,*,#18309,.T.) ;
#25223=ORIENTED_EDGE('',*,*,#18298,.F.) ;
#25224=ORIENTED_EDGE('',*,*,#18310,.F.) ;
#25225=ORIENTED_EDGE('',*,*,#18311,.F.) ;
#25226=ORIENTED_EDGE('',*,*,#18312,.F.) ;
#25227=ORIENTED_EDGE('',*,*,#18295,.F.) ;
#25228=ORIENTED_EDGE('',*,*,#18313,.T.) ;
#25229=ORIENTED_EDGE('',*,*,#18314,.T.) ;
#25230=ORIENTED_EDGE('',*,*,#18310,.T.) ;
#25231=ORIENTED_EDGE('',*,*,#18292,.F.) ;
#25232=ORIENTED_EDGE('',*,*,#18315,.F.) ;
#25233=ORIENTED_EDGE('',*,*,#18316,.F.) ;
#25234=ORIENTED_EDGE('',*,*,#18313,.F.) ;
#25235=ORIENTED_EDGE('',*,*,#18287,.F.) ;
#25236=ORIENTED_EDGE('',*,*,#18317,.T.) ;
#25237=ORIENTED_EDGE('',*,*,#18318,.T.) ;
#25238=ORIENTED_EDGE('',*,*,#18315,.T.) ;
#25239=ORIENTED_EDGE('',*,*,#18319,.T.) ;
#25240=ORIENTED_EDGE('',*,*,#18320,.F.) ;
#25241=ORIENTED_EDGE('',*,*,#18321,.T.) ;
#25242=ORIENTED_EDGE('',*,*,#18322,.F.) ;
#25243=ORIENTED_EDGE('',*,*,#18323,.F.) ;
#25244=ORIENTED_EDGE('',*,*,#18324,.F.) ;
#25245=ORIENTED_EDGE('',*,*,#18325,.F.) ;
#25246=ORIENTED_EDGE('',*,*,#18326,.F.) ;
#25247=ORIENTED_EDGE('',*,*,#18327,.F.) ;
#25248=ORIENTED_EDGE('',*,*,#18328,.F.) ;
#25249=ORIENTED_EDGE('',*,*,#18329,.F.) ;
#25250=ORIENTED_EDGE('',*,*,#18330,.F.) ;
#25251=ORIENTED_EDGE('',*,*,#18331,.T.) ;
#25252=ORIENTED_EDGE('',*,*,#18289,.F.) ;
#25253=ORIENTED_EDGE('',*,*,#18291,.F.) ;
#25254=ORIENTED_EDGE('',*,*,#18294,.F.) ;
#25255=ORIENTED_EDGE('',*,*,#18297,.F.) ;
#25256=ORIENTED_EDGE('',*,*,#18300,.F.) ;
#25257=ORIENTED_EDGE('',*,*,#18303,.F.) ;
#25258=ORIENTED_EDGE('',*,*,#18306,.F.) ;
#25259=ORIENTED_EDGE('',*,*,#18308,.F.) ;
#25260=ORIENTED_EDGE('',*,*,#18332,.T.) ;
#25261=ORIENTED_EDGE('',*,*,#18333,.T.) ;
#25262=ORIENTED_EDGE('',*,*,#18334,.T.) ;
#25263=ORIENTED_EDGE('',*,*,#18323,.T.) ;
#25264=ORIENTED_EDGE('',*,*,#18335,.T.) ;
#25265=ORIENTED_EDGE('',*,*,#18324,.T.) ;
#25266=ORIENTED_EDGE('',*,*,#18334,.F.) ;
#25267=ORIENTED_EDGE('',*,*,#18336,.T.) ;
#25268=ORIENTED_EDGE('',*,*,#18337,.T.) ;
#25269=ORIENTED_EDGE('',*,*,#18325,.T.) ;
#25270=ORIENTED_EDGE('',*,*,#18335,.F.) ;
#25271=ORIENTED_EDGE('',*,*,#18338,.T.) ;
#25272=ORIENTED_EDGE('',*,*,#18339,.T.) ;
#25273=ORIENTED_EDGE('',*,*,#18326,.T.) ;
#25274=ORIENTED_EDGE('',*,*,#18337,.F.) ;
#25275=ORIENTED_EDGE('',*,*,#18340,.T.) ;
#25276=ORIENTED_EDGE('',*,*,#18341,.T.) ;
#25277=ORIENTED_EDGE('',*,*,#18327,.T.) ;
#25278=ORIENTED_EDGE('',*,*,#18339,.F.) ;
#25279=ORIENTED_EDGE('',*,*,#18342,.T.) ;
#25280=ORIENTED_EDGE('',*,*,#18343,.T.) ;
#25281=ORIENTED_EDGE('',*,*,#18328,.T.) ;
#25282=ORIENTED_EDGE('',*,*,#18341,.F.) ;
#25283=ORIENTED_EDGE('',*,*,#18344,.T.) ;
#25284=ORIENTED_EDGE('',*,*,#18345,.T.) ;
#25285=ORIENTED_EDGE('',*,*,#18329,.T.) ;
#25286=ORIENTED_EDGE('',*,*,#18343,.F.) ;
#25287=ORIENTED_EDGE('',*,*,#17714,.T.) ;
#25288=ORIENTED_EDGE('',*,*,#18332,.F.) ;
#25289=ORIENTED_EDGE('',*,*,#18330,.T.) ;
#25290=ORIENTED_EDGE('',*,*,#18345,.F.) ;
#25291=ORIENTED_EDGE('',*,*,#18346,.T.) ;
#25292=ORIENTED_EDGE('',*,*,#18340,.F.) ;
#25293=ORIENTED_EDGE('',*,*,#18347,.F.) ;
#25294=ORIENTED_EDGE('',*,*,#18348,.T.) ;
#25295=ORIENTED_EDGE('',*,*,#18349,.T.) ;
#25296=ORIENTED_EDGE('',*,*,#18338,.F.) ;
#25297=ORIENTED_EDGE('',*,*,#18350,.T.) ;
#25298=ORIENTED_EDGE('',*,*,#18351,.T.) ;
#25299=ORIENTED_EDGE('',*,*,#18352,.T.) ;
#25300=ORIENTED_EDGE('',*,*,#18353,.T.) ;
#25301=ORIENTED_EDGE('',*,*,#17709,.F.) ;
#25302=ORIENTED_EDGE('',*,*,#18354,.T.) ;
#25303=ORIENTED_EDGE('',*,*,#18355,.T.) ;
#25304=ORIENTED_EDGE('',*,*,#18356,.T.) ;
#25305=ORIENTED_EDGE('',*,*,#18347,.T.) ;
#25306=ORIENTED_EDGE('',*,*,#18336,.F.) ;
#25307=ORIENTED_EDGE('',*,*,#18357,.T.) ;
#25308=ORIENTED_EDGE('',*,*,#18358,.T.) ;
#25309=ORIENTED_EDGE('',*,*,#18350,.F.) ;
#25310=ORIENTED_EDGE('',*,*,#18333,.F.) ;
#25311=ORIENTED_EDGE('',*,*,#18359,.T.) ;
#25312=ORIENTED_EDGE('',*,*,#18360,.T.) ;
#25313=ORIENTED_EDGE('',*,*,#18357,.F.) ;
#25314=ORIENTED_EDGE('',*,*,#18342,.F.) ;
#25315=ORIENTED_EDGE('',*,*,#18349,.F.) ;
#25316=ORIENTED_EDGE('',*,*,#18361,.T.) ;
#25317=ORIENTED_EDGE('',*,*,#18362,.T.) ;
#25318=ORIENTED_EDGE('',*,*,#18344,.F.) ;
#25319=ORIENTED_EDGE('',*,*,#18362,.F.) ;
#25320=ORIENTED_EDGE('',*,*,#18363,.T.) ;
#25321=ORIENTED_EDGE('',*,*,#17715,.F.) ;
#25322=ORIENTED_EDGE('',*,*,#18346,.F.) ;
#25323=ORIENTED_EDGE('',*,*,#17721,.F.) ;
#25324=ORIENTED_EDGE('',*,*,#18364,.T.) ;
#25325=ORIENTED_EDGE('',*,*,#18359,.F.) ;
#25326=ORIENTED_EDGE('',*,*,#18301,.F.) ;
#25327=ORIENTED_EDGE('',*,*,#18312,.T.) ;
#25328=ORIENTED_EDGE('',*,*,#18365,.T.) ;
#25329=ORIENTED_EDGE('',*,*,#18366,.T.) ;
#25330=ORIENTED_EDGE('',*,*,#18304,.F.) ;
#25331=ORIENTED_EDGE('',*,*,#18366,.F.) ;
#25332=ORIENTED_EDGE('',*,*,#18367,.T.) ;
#25333=ORIENTED_EDGE('',*,*,#18368,.F.) ;
#25334=ORIENTED_EDGE('',*,*,#18309,.F.) ;
#25335=ORIENTED_EDGE('',*,*,#18369,.F.) ;
#25336=ORIENTED_EDGE('',*,*,#18370,.T.) ;
#25337=ORIENTED_EDGE('',*,*,#18317,.F.) ;
#25338=ORIENTED_EDGE('',*,*,#18307,.F.) ;
#25339=ORIENTED_EDGE('',*,*,#18368,.T.) ;
#25340=ORIENTED_EDGE('',*,*,#18371,.T.) ;
#25341=ORIENTED_EDGE('',*,*,#18369,.T.) ;
#25342=ORIENTED_EDGE('',*,*,#18372,.T.) ;
#25343=ORIENTED_EDGE('',*,*,#17437,.T.) ;
#25344=ORIENTED_EDGE('',*,*,#17710,.F.) ;
#25345=ORIENTED_EDGE('',*,*,#18353,.F.) ;
#25346=ORIENTED_EDGE('',*,*,#18373,.F.) ;
#25347=ORIENTED_EDGE('',*,*,#17724,.F.) ;
#25348=ORIENTED_EDGE('',*,*,#18374,.F.) ;
#25349=ORIENTED_EDGE('',*,*,#18361,.F.) ;
#25350=ORIENTED_EDGE('',*,*,#18375,.F.) ;
#25351=ORIENTED_EDGE('',*,*,#18376,.F.) ;
#25352=ORIENTED_EDGE('',*,*,#18377,.T.) ;
#25353=ORIENTED_EDGE('',*,*,#18373,.T.) ;
#25354=ORIENTED_EDGE('',*,*,#18352,.F.) ;
#25355=ORIENTED_EDGE('',*,*,#18378,.T.) ;
#25356=ORIENTED_EDGE('',*,*,#18379,.F.) ;
#25357=ORIENTED_EDGE('',*,*,#18380,.F.) ;
#25358=ORIENTED_EDGE('',*,*,#18378,.F.) ;
#25359=ORIENTED_EDGE('',*,*,#18351,.F.) ;
#25360=ORIENTED_EDGE('',*,*,#18381,.T.) ;
#25361=ORIENTED_EDGE('',*,*,#18382,.T.) ;
#25362=ORIENTED_EDGE('',*,*,#17719,.F.) ;
#25363=ORIENTED_EDGE('',*,*,#17723,.T.) ;
#25364=ORIENTED_EDGE('',*,*,#18383,.T.) ;
#25365=ORIENTED_EDGE('',*,*,#18384,.T.) ;
#25366=ORIENTED_EDGE('',*,*,#18355,.F.) ;
#25367=ORIENTED_EDGE('',*,*,#18385,.T.) ;
#25368=ORIENTED_EDGE('',*,*,#17707,.F.) ;
#25369=ORIENTED_EDGE('',*,*,#18386,.F.) ;
#25370=ORIENTED_EDGE('',*,*,#18385,.F.) ;
#25371=ORIENTED_EDGE('',*,*,#18354,.F.) ;
#25372=ORIENTED_EDGE('',*,*,#18387,.F.) ;
#25373=ORIENTED_EDGE('',*,*,#18356,.F.) ;
#25374=ORIENTED_EDGE('',*,*,#18384,.F.) ;
#25375=ORIENTED_EDGE('',*,*,#18388,.F.) ;
#25376=ORIENTED_EDGE('',*,*,#18389,.T.) ;
#25377=ORIENTED_EDGE('',*,*,#17712,.T.) ;
#25378=ORIENTED_EDGE('',*,*,#17717,.F.) ;
#25379=ORIENTED_EDGE('',*,*,#18390,.T.) ;
#25380=ORIENTED_EDGE('',*,*,#18391,.F.) ;
#25381=ORIENTED_EDGE('',*,*,#18392,.F.) ;
#25382=ORIENTED_EDGE('',*,*,#18390,.F.) ;
#25383=ORIENTED_EDGE('',*,*,#17716,.F.) ;
#25384=ORIENTED_EDGE('',*,*,#18389,.F.) ;
#25385=ORIENTED_EDGE('',*,*,#18393,.F.) ;
#25386=ORIENTED_EDGE('',*,*,#18383,.F.) ;
#25387=ORIENTED_EDGE('',*,*,#18394,.F.) ;
#25388=ORIENTED_EDGE('',*,*,#18395,.F.) ;
#25389=ORIENTED_EDGE('',*,*,#17720,.F.) ;
#25390=ORIENTED_EDGE('',*,*,#18382,.F.) ;
#25391=ORIENTED_EDGE('',*,*,#18396,.F.) ;
#25392=ORIENTED_EDGE('',*,*,#18377,.F.) ;
#25393=ORIENTED_EDGE('',*,*,#18397,.F.) ;
#25394=ORIENTED_EDGE('',*,*,#18381,.F.) ;
#25395=ORIENTED_EDGE('',*,*,#17725,.F.) ;
#25396=ORIENTED_EDGE('',*,*,#18391,.T.) ;
#25397=ORIENTED_EDGE('',*,*,#18363,.F.) ;
#25398=ORIENTED_EDGE('',*,*,#18374,.T.) ;
#25399=ORIENTED_EDGE('',*,*,#18375,.T.) ;
#25400=ORIENTED_EDGE('',*,*,#18348,.F.) ;
#25401=ORIENTED_EDGE('',*,*,#18387,.T.) ;
#25402=ORIENTED_EDGE('',*,*,#18398,.F.) ;
#25403=ORIENTED_EDGE('',*,*,#18399,.F.) ;
#25404=ORIENTED_EDGE('',*,*,#18400,.F.) ;
#25405=ORIENTED_EDGE('',*,*,#18360,.F.) ;
#25406=ORIENTED_EDGE('',*,*,#18398,.T.) ;
#25407=ORIENTED_EDGE('',*,*,#18364,.F.) ;
#25408=ORIENTED_EDGE('',*,*,#18395,.T.) ;
#25409=ORIENTED_EDGE('',*,*,#18379,.T.) ;
#25410=ORIENTED_EDGE('',*,*,#18358,.F.) ;
#25411=ORIENTED_EDGE('',*,*,#18400,.T.) ;
#25412=ORIENTED_EDGE('',*,*,#17705,.F.) ;
#25413=ORIENTED_EDGE('',*,*,#17713,.T.) ;
#25414=ORIENTED_EDGE('',*,*,#18394,.T.) ;
#25415=ORIENTED_EDGE('',*,*,#18386,.T.) ;
#25416=ORIENTED_EDGE('',*,*,#18376,.T.) ;
#25417=ORIENTED_EDGE('',*,*,#18388,.T.) ;
#25418=ORIENTED_EDGE('',*,*,#18393,.T.) ;
#25419=ORIENTED_EDGE('',*,*,#18392,.T.) ;
#25420=ORIENTED_EDGE('',*,*,#18396,.T.) ;
#25421=ORIENTED_EDGE('',*,*,#18397,.T.) ;
#25422=ORIENTED_EDGE('',*,*,#18380,.T.) ;
#25423=ORIENTED_EDGE('',*,*,#18399,.T.) ;
#25424=ORIENTED_EDGE('',*,*,#18401,.T.) ;
#25425=ORIENTED_EDGE('',*,*,#18402,.T.) ;
#25426=ORIENTED_EDGE('',*,*,#18403,.T.) ;
#25427=ORIENTED_EDGE('',*,*,#18404,.T.) ;
#25428=ORIENTED_EDGE('',*,*,#18405,.T.) ;
#25429=ORIENTED_EDGE('',*,*,#18406,.T.) ;
#25430=ORIENTED_EDGE('',*,*,#18367,.F.) ;
#25431=ORIENTED_EDGE('',*,*,#18407,.T.) ;
#25432=ORIENTED_EDGE('',*,*,#18408,.T.) ;
#25433=ORIENTED_EDGE('',*,*,#18370,.F.) ;
#25434=ORIENTED_EDGE('',*,*,#18371,.F.) ;
#25435=ORIENTED_EDGE('',*,*,#18406,.F.) ;
#25436=ORIENTED_EDGE('',*,*,#18401,.F.) ;
#25437=ORIENTED_EDGE('',*,*,#18407,.F.) ;
#25438=ORIENTED_EDGE('',*,*,#18408,.F.) ;
#25439=ORIENTED_EDGE('',*,*,#18404,.F.) ;
#25440=ORIENTED_EDGE('',*,*,#18409,.F.) ;
#25441=ORIENTED_EDGE('',*,*,#18318,.F.) ;
#25442=ORIENTED_EDGE('',*,*,#18405,.F.) ;
#25443=ORIENTED_EDGE('',*,*,#18365,.F.) ;
#25444=ORIENTED_EDGE('',*,*,#18410,.F.) ;
#25445=ORIENTED_EDGE('',*,*,#18402,.F.) ;
#25446=ORIENTED_EDGE('',*,*,#18403,.F.) ;
#25447=ORIENTED_EDGE('',*,*,#18411,.F.) ;
#25448=ORIENTED_EDGE('',*,*,#18314,.F.) ;
#25449=ORIENTED_EDGE('',*,*,#18412,.F.) ;
#25450=ORIENTED_EDGE('',*,*,#18410,.T.) ;
#25451=ORIENTED_EDGE('',*,*,#18311,.T.) ;
#25452=ORIENTED_EDGE('',*,*,#18411,.T.) ;
#25453=ORIENTED_EDGE('',*,*,#18316,.T.) ;
#25454=ORIENTED_EDGE('',*,*,#18409,.T.) ;
#25455=ORIENTED_EDGE('',*,*,#18412,.T.) ;
#25456=ORIENTED_EDGE('',*,*,#17679,.F.) ;
#25457=ORIENTED_EDGE('',*,*,#18281,.F.) ;
#25458=ORIENTED_EDGE('',*,*,#18413,.F.) ;
#25459=ORIENTED_EDGE('',*,*,#17693,.F.) ;
#25460=ORIENTED_EDGE('',*,*,#18414,.F.) ;
#25461=ORIENTED_EDGE('',*,*,#18415,.F.) ;
#25462=ORIENTED_EDGE('',*,*,#18416,.F.) ;
#25463=ORIENTED_EDGE('',*,*,#18417,.F.) ;
#25464=ORIENTED_EDGE('',*,*,#18418,.T.) ;
#25465=ORIENTED_EDGE('',*,*,#18413,.T.) ;
#25466=ORIENTED_EDGE('',*,*,#18280,.F.) ;
#25467=ORIENTED_EDGE('',*,*,#18419,.T.) ;
#25468=ORIENTED_EDGE('',*,*,#18420,.F.) ;
#25469=ORIENTED_EDGE('',*,*,#18421,.F.) ;
#25470=ORIENTED_EDGE('',*,*,#18419,.F.) ;
#25471=ORIENTED_EDGE('',*,*,#18279,.F.) ;
#25472=ORIENTED_EDGE('',*,*,#18422,.T.) ;
#25473=ORIENTED_EDGE('',*,*,#18423,.T.) ;
#25474=ORIENTED_EDGE('',*,*,#17684,.F.) ;
#25475=ORIENTED_EDGE('',*,*,#17692,.T.) ;
#25476=ORIENTED_EDGE('',*,*,#18424,.T.) ;
#25477=ORIENTED_EDGE('',*,*,#18425,.T.) ;
#25478=ORIENTED_EDGE('',*,*,#18276,.F.) ;
#25479=ORIENTED_EDGE('',*,*,#18426,.T.) ;
#25480=ORIENTED_EDGE('',*,*,#17676,.T.) ;
#25481=ORIENTED_EDGE('',*,*,#18427,.F.) ;
#25482=ORIENTED_EDGE('',*,*,#18426,.F.) ;
#25483=ORIENTED_EDGE('',*,*,#18275,.F.) ;
#25484=ORIENTED_EDGE('',*,*,#18428,.F.) ;
#25485=ORIENTED_EDGE('',*,*,#18277,.F.) ;
#25486=ORIENTED_EDGE('',*,*,#18425,.F.) ;
#25487=ORIENTED_EDGE('',*,*,#18429,.F.) ;
#25488=ORIENTED_EDGE('',*,*,#18430,.T.) ;
#25489=ORIENTED_EDGE('',*,*,#17681,.T.) ;
#25490=ORIENTED_EDGE('',*,*,#17690,.F.) ;
#25491=ORIENTED_EDGE('',*,*,#18431,.T.) ;
#25492=ORIENTED_EDGE('',*,*,#18432,.F.) ;
#25493=ORIENTED_EDGE('',*,*,#18433,.F.) ;
#25494=ORIENTED_EDGE('',*,*,#18431,.F.) ;
#25495=ORIENTED_EDGE('',*,*,#17689,.F.) ;
#25496=ORIENTED_EDGE('',*,*,#18430,.F.) ;
#25497=ORIENTED_EDGE('',*,*,#18434,.F.) ;
#25498=ORIENTED_EDGE('',*,*,#18424,.F.) ;
#25499=ORIENTED_EDGE('',*,*,#18435,.F.) ;
#25500=ORIENTED_EDGE('',*,*,#18436,.F.) ;
#25501=ORIENTED_EDGE('',*,*,#17685,.F.) ;
#25502=ORIENTED_EDGE('',*,*,#18423,.F.) ;
#25503=ORIENTED_EDGE('',*,*,#18437,.F.) ;
#25504=ORIENTED_EDGE('',*,*,#18418,.F.) ;
#25505=ORIENTED_EDGE('',*,*,#18438,.F.) ;
#25506=ORIENTED_EDGE('',*,*,#18422,.F.) ;
#25507=ORIENTED_EDGE('',*,*,#17694,.F.) ;
#25508=ORIENTED_EDGE('',*,*,#18432,.T.) ;
#25509=ORIENTED_EDGE('',*,*,#18439,.F.) ;
#25510=ORIENTED_EDGE('',*,*,#18414,.T.) ;
#25511=ORIENTED_EDGE('',*,*,#18416,.T.) ;
#25512=ORIENTED_EDGE('',*,*,#18273,.F.) ;
#25513=ORIENTED_EDGE('',*,*,#18428,.T.) ;
#25514=ORIENTED_EDGE('',*,*,#18440,.F.) ;
#25515=ORIENTED_EDGE('',*,*,#18441,.F.) ;
#25516=ORIENTED_EDGE('',*,*,#18442,.F.) ;
#25517=ORIENTED_EDGE('',*,*,#18285,.F.) ;
#25518=ORIENTED_EDGE('',*,*,#18440,.T.) ;
#25519=ORIENTED_EDGE('',*,*,#18443,.F.) ;
#25520=ORIENTED_EDGE('',*,*,#18436,.T.) ;
#25521=ORIENTED_EDGE('',*,*,#18420,.T.) ;
#25522=ORIENTED_EDGE('',*,*,#18283,.F.) ;
#25523=ORIENTED_EDGE('',*,*,#18442,.T.) ;
#25524=ORIENTED_EDGE('',*,*,#17674,.F.) ;
#25525=ORIENTED_EDGE('',*,*,#17682,.T.) ;
#25526=ORIENTED_EDGE('',*,*,#18435,.T.) ;
#25527=ORIENTED_EDGE('',*,*,#18427,.T.) ;
#25528=ORIENTED_EDGE('',*,*,#18417,.T.) ;
#25529=ORIENTED_EDGE('',*,*,#18429,.T.) ;
#25530=ORIENTED_EDGE('',*,*,#18434,.T.) ;
#25531=ORIENTED_EDGE('',*,*,#18433,.T.) ;
#25532=ORIENTED_EDGE('',*,*,#18437,.T.) ;
#25533=ORIENTED_EDGE('',*,*,#18438,.T.) ;
#25534=ORIENTED_EDGE('',*,*,#18421,.T.) ;
#25535=ORIENTED_EDGE('',*,*,#18441,.T.) ;
#25536=ORIENTED_EDGE('',*,*,#18444,.T.) ;
#25537=ORIENTED_EDGE('',*,*,#18445,.T.) ;
#25538=ORIENTED_EDGE('',*,*,#18446,.T.) ;
#25539=ORIENTED_EDGE('',*,*,#18447,.T.) ;
#25540=ORIENTED_EDGE('',*,*,#18448,.T.) ;
#25541=ORIENTED_EDGE('',*,*,#18449,.T.) ;
#25542=ORIENTED_EDGE('',*,*,#18450,.F.) ;
#25543=ORIENTED_EDGE('',*,*,#18451,.T.) ;
#25544=ORIENTED_EDGE('',*,*,#18452,.T.) ;
#25545=ORIENTED_EDGE('',*,*,#18453,.F.) ;
#25546=ORIENTED_EDGE('',*,*,#18454,.F.) ;
#25547=ORIENTED_EDGE('',*,*,#18449,.F.) ;
#25548=ORIENTED_EDGE('',*,*,#18444,.F.) ;
#25549=ORIENTED_EDGE('',*,*,#18451,.F.) ;
#25550=ORIENTED_EDGE('',*,*,#18452,.F.) ;
#25551=ORIENTED_EDGE('',*,*,#18447,.F.) ;
#25552=ORIENTED_EDGE('',*,*,#18455,.F.) ;
#25553=ORIENTED_EDGE('',*,*,#17989,.F.) ;
#25554=ORIENTED_EDGE('',*,*,#18448,.F.) ;
#25555=ORIENTED_EDGE('',*,*,#18456,.F.) ;
#25556=ORIENTED_EDGE('',*,*,#18457,.F.) ;
#25557=ORIENTED_EDGE('',*,*,#18445,.F.) ;
#25558=ORIENTED_EDGE('',*,*,#18446,.F.) ;
#25559=ORIENTED_EDGE('',*,*,#18458,.F.) ;
#25560=ORIENTED_EDGE('',*,*,#17985,.F.) ;
#25561=ORIENTED_EDGE('',*,*,#18459,.F.) ;
#25562=ORIENTED_EDGE('',*,*,#18457,.T.) ;
#25563=ORIENTED_EDGE('',*,*,#17982,.T.) ;
#25564=ORIENTED_EDGE('',*,*,#18458,.T.) ;
#25565=ORIENTED_EDGE('',*,*,#17987,.T.) ;
#25566=ORIENTED_EDGE('',*,*,#18455,.T.) ;
#25567=ORIENTED_EDGE('',*,*,#18459,.T.) ;
#25568=ORIENTED_EDGE('',*,*,#17648,.F.) ;
#25569=ORIENTED_EDGE('',*,*,#18244,.F.) ;
#25570=ORIENTED_EDGE('',*,*,#18460,.F.) ;
#25571=ORIENTED_EDGE('',*,*,#17662,.F.) ;
#25572=ORIENTED_EDGE('',*,*,#18461,.F.) ;
#25573=ORIENTED_EDGE('',*,*,#18462,.F.) ;
#25574=ORIENTED_EDGE('',*,*,#18463,.F.) ;
#25575=ORIENTED_EDGE('',*,*,#18464,.F.) ;
#25576=ORIENTED_EDGE('',*,*,#18465,.T.) ;
#25577=ORIENTED_EDGE('',*,*,#18460,.T.) ;
#25578=ORIENTED_EDGE('',*,*,#18243,.F.) ;
#25579=ORIENTED_EDGE('',*,*,#18466,.T.) ;
#25580=ORIENTED_EDGE('',*,*,#18467,.F.) ;
#25581=ORIENTED_EDGE('',*,*,#18468,.F.) ;
#25582=ORIENTED_EDGE('',*,*,#18466,.F.) ;
#25583=ORIENTED_EDGE('',*,*,#18242,.F.) ;
#25584=ORIENTED_EDGE('',*,*,#18469,.T.) ;
#25585=ORIENTED_EDGE('',*,*,#18470,.T.) ;
#25586=ORIENTED_EDGE('',*,*,#17653,.F.) ;
#25587=ORIENTED_EDGE('',*,*,#17661,.T.) ;
#25588=ORIENTED_EDGE('',*,*,#18471,.T.) ;
#25589=ORIENTED_EDGE('',*,*,#18472,.T.) ;
#25590=ORIENTED_EDGE('',*,*,#18239,.F.) ;
#25591=ORIENTED_EDGE('',*,*,#18473,.T.) ;
#25592=ORIENTED_EDGE('',*,*,#17645,.T.) ;
#25593=ORIENTED_EDGE('',*,*,#18474,.F.) ;
#25594=ORIENTED_EDGE('',*,*,#18473,.F.) ;
#25595=ORIENTED_EDGE('',*,*,#18238,.F.) ;
#25596=ORIENTED_EDGE('',*,*,#18475,.F.) ;
#25597=ORIENTED_EDGE('',*,*,#18240,.F.) ;
#25598=ORIENTED_EDGE('',*,*,#18472,.F.) ;
#25599=ORIENTED_EDGE('',*,*,#18476,.F.) ;
#25600=ORIENTED_EDGE('',*,*,#18477,.T.) ;
#25601=ORIENTED_EDGE('',*,*,#17650,.T.) ;
#25602=ORIENTED_EDGE('',*,*,#17659,.F.) ;
#25603=ORIENTED_EDGE('',*,*,#18478,.T.) ;
#25604=ORIENTED_EDGE('',*,*,#18479,.F.) ;
#25605=ORIENTED_EDGE('',*,*,#18480,.F.) ;
#25606=ORIENTED_EDGE('',*,*,#18478,.F.) ;
#25607=ORIENTED_EDGE('',*,*,#17658,.F.) ;
#25608=ORIENTED_EDGE('',*,*,#18477,.F.) ;
#25609=ORIENTED_EDGE('',*,*,#18481,.F.) ;
#25610=ORIENTED_EDGE('',*,*,#18471,.F.) ;
#25611=ORIENTED_EDGE('',*,*,#18482,.F.) ;
#25612=ORIENTED_EDGE('',*,*,#18483,.F.) ;
#25613=ORIENTED_EDGE('',*,*,#17654,.F.) ;
#25614=ORIENTED_EDGE('',*,*,#18470,.F.) ;
#25615=ORIENTED_EDGE('',*,*,#18484,.F.) ;
#25616=ORIENTED_EDGE('',*,*,#18465,.F.) ;
#25617=ORIENTED_EDGE('',*,*,#18485,.F.) ;
#25618=ORIENTED_EDGE('',*,*,#18469,.F.) ;
#25619=ORIENTED_EDGE('',*,*,#17663,.F.) ;
#25620=ORIENTED_EDGE('',*,*,#18479,.T.) ;
#25621=ORIENTED_EDGE('',*,*,#18486,.F.) ;
#25622=ORIENTED_EDGE('',*,*,#18461,.T.) ;
#25623=ORIENTED_EDGE('',*,*,#18463,.T.) ;
#25624=ORIENTED_EDGE('',*,*,#18236,.F.) ;
#25625=ORIENTED_EDGE('',*,*,#18475,.T.) ;
#25626=ORIENTED_EDGE('',*,*,#18487,.F.) ;
#25627=ORIENTED_EDGE('',*,*,#18488,.F.) ;
#25628=ORIENTED_EDGE('',*,*,#18489,.F.) ;
#25629=ORIENTED_EDGE('',*,*,#18248,.F.) ;
#25630=ORIENTED_EDGE('',*,*,#18487,.T.) ;
#25631=ORIENTED_EDGE('',*,*,#18490,.F.) ;
#25632=ORIENTED_EDGE('',*,*,#18483,.T.) ;
#25633=ORIENTED_EDGE('',*,*,#18467,.T.) ;
#25634=ORIENTED_EDGE('',*,*,#18246,.F.) ;
#25635=ORIENTED_EDGE('',*,*,#18489,.T.) ;
#25636=ORIENTED_EDGE('',*,*,#17643,.F.) ;
#25637=ORIENTED_EDGE('',*,*,#17651,.T.) ;
#25638=ORIENTED_EDGE('',*,*,#18482,.T.) ;
#25639=ORIENTED_EDGE('',*,*,#18474,.T.) ;
#25640=ORIENTED_EDGE('',*,*,#18464,.T.) ;
#25641=ORIENTED_EDGE('',*,*,#18476,.T.) ;
#25642=ORIENTED_EDGE('',*,*,#18481,.T.) ;
#25643=ORIENTED_EDGE('',*,*,#18480,.T.) ;
#25644=ORIENTED_EDGE('',*,*,#18484,.T.) ;
#25645=ORIENTED_EDGE('',*,*,#18485,.T.) ;
#25646=ORIENTED_EDGE('',*,*,#18468,.T.) ;
#25647=ORIENTED_EDGE('',*,*,#18488,.T.) ;
#25648=ORIENTED_EDGE('',*,*,#18491,.T.) ;
#25649=ORIENTED_EDGE('',*,*,#18492,.T.) ;
#25650=ORIENTED_EDGE('',*,*,#18493,.T.) ;
#25651=ORIENTED_EDGE('',*,*,#18494,.T.) ;
#25652=ORIENTED_EDGE('',*,*,#18495,.T.) ;
#25653=ORIENTED_EDGE('',*,*,#18496,.T.) ;
#25654=ORIENTED_EDGE('',*,*,#18497,.F.) ;
#25655=ORIENTED_EDGE('',*,*,#18498,.T.) ;
#25656=ORIENTED_EDGE('',*,*,#18499,.T.) ;
#25657=ORIENTED_EDGE('',*,*,#18500,.F.) ;
#25658=ORIENTED_EDGE('',*,*,#18501,.F.) ;
#25659=ORIENTED_EDGE('',*,*,#18496,.F.) ;
#25660=ORIENTED_EDGE('',*,*,#18491,.F.) ;
#25661=ORIENTED_EDGE('',*,*,#18498,.F.) ;
#25662=ORIENTED_EDGE('',*,*,#18499,.F.) ;
#25663=ORIENTED_EDGE('',*,*,#18494,.F.) ;
#25664=ORIENTED_EDGE('',*,*,#18502,.F.) ;
#25665=ORIENTED_EDGE('',*,*,#17956,.F.) ;
#25666=ORIENTED_EDGE('',*,*,#18495,.F.) ;
#25667=ORIENTED_EDGE('',*,*,#18503,.F.) ;
#25668=ORIENTED_EDGE('',*,*,#18504,.F.) ;
#25669=ORIENTED_EDGE('',*,*,#18492,.F.) ;
#25670=ORIENTED_EDGE('',*,*,#18493,.F.) ;
#25671=ORIENTED_EDGE('',*,*,#18505,.F.) ;
#25672=ORIENTED_EDGE('',*,*,#17952,.F.) ;
#25673=ORIENTED_EDGE('',*,*,#18506,.F.) ;
#25674=ORIENTED_EDGE('',*,*,#18504,.T.) ;
#25675=ORIENTED_EDGE('',*,*,#17949,.T.) ;
#25676=ORIENTED_EDGE('',*,*,#18505,.T.) ;
#25677=ORIENTED_EDGE('',*,*,#17954,.T.) ;
#25678=ORIENTED_EDGE('',*,*,#18502,.T.) ;
#25679=ORIENTED_EDGE('',*,*,#18506,.T.) ;
#25680=ORIENTED_EDGE('',*,*,#17617,.F.) ;
#25681=ORIENTED_EDGE('',*,*,#18207,.F.) ;
#25682=ORIENTED_EDGE('',*,*,#18507,.F.) ;
#25683=ORIENTED_EDGE('',*,*,#17631,.F.) ;
#25684=ORIENTED_EDGE('',*,*,#18508,.F.) ;
#25685=ORIENTED_EDGE('',*,*,#18509,.F.) ;
#25686=ORIENTED_EDGE('',*,*,#18510,.F.) ;
#25687=ORIENTED_EDGE('',*,*,#18511,.F.) ;
#25688=ORIENTED_EDGE('',*,*,#18512,.T.) ;
#25689=ORIENTED_EDGE('',*,*,#18507,.T.) ;
#25690=ORIENTED_EDGE('',*,*,#18206,.F.) ;
#25691=ORIENTED_EDGE('',*,*,#18513,.T.) ;
#25692=ORIENTED_EDGE('',*,*,#18514,.F.) ;
#25693=ORIENTED_EDGE('',*,*,#18515,.F.) ;
#25694=ORIENTED_EDGE('',*,*,#18513,.F.) ;
#25695=ORIENTED_EDGE('',*,*,#18205,.F.) ;
#25696=ORIENTED_EDGE('',*,*,#18516,.T.) ;
#25697=ORIENTED_EDGE('',*,*,#18517,.T.) ;
#25698=ORIENTED_EDGE('',*,*,#17622,.F.) ;
#25699=ORIENTED_EDGE('',*,*,#17630,.T.) ;
#25700=ORIENTED_EDGE('',*,*,#18518,.T.) ;
#25701=ORIENTED_EDGE('',*,*,#18519,.T.) ;
#25702=ORIENTED_EDGE('',*,*,#18202,.F.) ;
#25703=ORIENTED_EDGE('',*,*,#18520,.T.) ;
#25704=ORIENTED_EDGE('',*,*,#17614,.T.) ;
#25705=ORIENTED_EDGE('',*,*,#18521,.F.) ;
#25706=ORIENTED_EDGE('',*,*,#18520,.F.) ;
#25707=ORIENTED_EDGE('',*,*,#18201,.F.) ;
#25708=ORIENTED_EDGE('',*,*,#18522,.F.) ;
#25709=ORIENTED_EDGE('',*,*,#18203,.F.) ;
#25710=ORIENTED_EDGE('',*,*,#18519,.F.) ;
#25711=ORIENTED_EDGE('',*,*,#18523,.F.) ;
#25712=ORIENTED_EDGE('',*,*,#18524,.T.) ;
#25713=ORIENTED_EDGE('',*,*,#17619,.T.) ;
#25714=ORIENTED_EDGE('',*,*,#17628,.F.) ;
#25715=ORIENTED_EDGE('',*,*,#18525,.T.) ;
#25716=ORIENTED_EDGE('',*,*,#18526,.F.) ;
#25717=ORIENTED_EDGE('',*,*,#18527,.F.) ;
#25718=ORIENTED_EDGE('',*,*,#18525,.F.) ;
#25719=ORIENTED_EDGE('',*,*,#17627,.F.) ;
#25720=ORIENTED_EDGE('',*,*,#18524,.F.) ;
#25721=ORIENTED_EDGE('',*,*,#18528,.F.) ;
#25722=ORIENTED_EDGE('',*,*,#18518,.F.) ;
#25723=ORIENTED_EDGE('',*,*,#18529,.F.) ;
#25724=ORIENTED_EDGE('',*,*,#18530,.F.) ;
#25725=ORIENTED_EDGE('',*,*,#17623,.F.) ;
#25726=ORIENTED_EDGE('',*,*,#18517,.F.) ;
#25727=ORIENTED_EDGE('',*,*,#18531,.F.) ;
#25728=ORIENTED_EDGE('',*,*,#18512,.F.) ;
#25729=ORIENTED_EDGE('',*,*,#18532,.F.) ;
#25730=ORIENTED_EDGE('',*,*,#18516,.F.) ;
#25731=ORIENTED_EDGE('',*,*,#17632,.F.) ;
#25732=ORIENTED_EDGE('',*,*,#18526,.T.) ;
#25733=ORIENTED_EDGE('',*,*,#18533,.F.) ;
#25734=ORIENTED_EDGE('',*,*,#18508,.T.) ;
#25735=ORIENTED_EDGE('',*,*,#18510,.T.) ;
#25736=ORIENTED_EDGE('',*,*,#18199,.F.) ;
#25737=ORIENTED_EDGE('',*,*,#18522,.T.) ;
#25738=ORIENTED_EDGE('',*,*,#18534,.F.) ;
#25739=ORIENTED_EDGE('',*,*,#18535,.F.) ;
#25740=ORIENTED_EDGE('',*,*,#18536,.F.) ;
#25741=ORIENTED_EDGE('',*,*,#18211,.F.) ;
#25742=ORIENTED_EDGE('',*,*,#18534,.T.) ;
#25743=ORIENTED_EDGE('',*,*,#18537,.F.) ;
#25744=ORIENTED_EDGE('',*,*,#18530,.T.) ;
#25745=ORIENTED_EDGE('',*,*,#18514,.T.) ;
#25746=ORIENTED_EDGE('',*,*,#18209,.F.) ;
#25747=ORIENTED_EDGE('',*,*,#18536,.T.) ;
#25748=ORIENTED_EDGE('',*,*,#17612,.F.) ;
#25749=ORIENTED_EDGE('',*,*,#17620,.T.) ;
#25750=ORIENTED_EDGE('',*,*,#18529,.T.) ;
#25751=ORIENTED_EDGE('',*,*,#18521,.T.) ;
#25752=ORIENTED_EDGE('',*,*,#18511,.T.) ;
#25753=ORIENTED_EDGE('',*,*,#18523,.T.) ;
#25754=ORIENTED_EDGE('',*,*,#18528,.T.) ;
#25755=ORIENTED_EDGE('',*,*,#18527,.T.) ;
#25756=ORIENTED_EDGE('',*,*,#18531,.T.) ;
#25757=ORIENTED_EDGE('',*,*,#18532,.T.) ;
#25758=ORIENTED_EDGE('',*,*,#18515,.T.) ;
#25759=ORIENTED_EDGE('',*,*,#18535,.T.) ;
#25760=ORIENTED_EDGE('',*,*,#18538,.T.) ;
#25761=ORIENTED_EDGE('',*,*,#18539,.T.) ;
#25762=ORIENTED_EDGE('',*,*,#18540,.T.) ;
#25763=ORIENTED_EDGE('',*,*,#18541,.T.) ;
#25764=ORIENTED_EDGE('',*,*,#18542,.T.) ;
#25765=ORIENTED_EDGE('',*,*,#18543,.T.) ;
#25766=ORIENTED_EDGE('',*,*,#18544,.F.) ;
#25767=ORIENTED_EDGE('',*,*,#18545,.T.) ;
#25768=ORIENTED_EDGE('',*,*,#18546,.T.) ;
#25769=ORIENTED_EDGE('',*,*,#18547,.F.) ;
#25770=ORIENTED_EDGE('',*,*,#18548,.F.) ;
#25771=ORIENTED_EDGE('',*,*,#18543,.F.) ;
#25772=ORIENTED_EDGE('',*,*,#18538,.F.) ;
#25773=ORIENTED_EDGE('',*,*,#18545,.F.) ;
#25774=ORIENTED_EDGE('',*,*,#18546,.F.) ;
#25775=ORIENTED_EDGE('',*,*,#18541,.F.) ;
#25776=ORIENTED_EDGE('',*,*,#18549,.F.) ;
#25777=ORIENTED_EDGE('',*,*,#17923,.F.) ;
#25778=ORIENTED_EDGE('',*,*,#18542,.F.) ;
#25779=ORIENTED_EDGE('',*,*,#18550,.F.) ;
#25780=ORIENTED_EDGE('',*,*,#18551,.F.) ;
#25781=ORIENTED_EDGE('',*,*,#18539,.F.) ;
#25782=ORIENTED_EDGE('',*,*,#18540,.F.) ;
#25783=ORIENTED_EDGE('',*,*,#18552,.F.) ;
#25784=ORIENTED_EDGE('',*,*,#17919,.F.) ;
#25785=ORIENTED_EDGE('',*,*,#18553,.F.) ;
#25786=ORIENTED_EDGE('',*,*,#18551,.T.) ;
#25787=ORIENTED_EDGE('',*,*,#17916,.T.) ;
#25788=ORIENTED_EDGE('',*,*,#18552,.T.) ;
#25789=ORIENTED_EDGE('',*,*,#17921,.T.) ;
#25790=ORIENTED_EDGE('',*,*,#18549,.T.) ;
#25791=ORIENTED_EDGE('',*,*,#18553,.T.) ;
#25792=ORIENTED_EDGE('',*,*,#17586,.F.) ;
#25793=ORIENTED_EDGE('',*,*,#18170,.F.) ;
#25794=ORIENTED_EDGE('',*,*,#18554,.F.) ;
#25795=ORIENTED_EDGE('',*,*,#17600,.F.) ;
#25796=ORIENTED_EDGE('',*,*,#18555,.F.) ;
#25797=ORIENTED_EDGE('',*,*,#18556,.F.) ;
#25798=ORIENTED_EDGE('',*,*,#18557,.F.) ;
#25799=ORIENTED_EDGE('',*,*,#18558,.F.) ;
#25800=ORIENTED_EDGE('',*,*,#18559,.T.) ;
#25801=ORIENTED_EDGE('',*,*,#18554,.T.) ;
#25802=ORIENTED_EDGE('',*,*,#18169,.F.) ;
#25803=ORIENTED_EDGE('',*,*,#18560,.T.) ;
#25804=ORIENTED_EDGE('',*,*,#18561,.F.) ;
#25805=ORIENTED_EDGE('',*,*,#18562,.F.) ;
#25806=ORIENTED_EDGE('',*,*,#18560,.F.) ;
#25807=ORIENTED_EDGE('',*,*,#18168,.F.) ;
#25808=ORIENTED_EDGE('',*,*,#18563,.T.) ;
#25809=ORIENTED_EDGE('',*,*,#18564,.T.) ;
#25810=ORIENTED_EDGE('',*,*,#17591,.F.) ;
#25811=ORIENTED_EDGE('',*,*,#17599,.T.) ;
#25812=ORIENTED_EDGE('',*,*,#18565,.T.) ;
#25813=ORIENTED_EDGE('',*,*,#18566,.T.) ;
#25814=ORIENTED_EDGE('',*,*,#18165,.F.) ;
#25815=ORIENTED_EDGE('',*,*,#18567,.T.) ;
#25816=ORIENTED_EDGE('',*,*,#17583,.T.) ;
#25817=ORIENTED_EDGE('',*,*,#18568,.F.) ;
#25818=ORIENTED_EDGE('',*,*,#18567,.F.) ;
#25819=ORIENTED_EDGE('',*,*,#18164,.F.) ;
#25820=ORIENTED_EDGE('',*,*,#18569,.F.) ;
#25821=ORIENTED_EDGE('',*,*,#18166,.F.) ;
#25822=ORIENTED_EDGE('',*,*,#18566,.F.) ;
#25823=ORIENTED_EDGE('',*,*,#18570,.F.) ;
#25824=ORIENTED_EDGE('',*,*,#18571,.T.) ;
#25825=ORIENTED_EDGE('',*,*,#17588,.T.) ;
#25826=ORIENTED_EDGE('',*,*,#17597,.F.) ;
#25827=ORIENTED_EDGE('',*,*,#18572,.T.) ;
#25828=ORIENTED_EDGE('',*,*,#18573,.F.) ;
#25829=ORIENTED_EDGE('',*,*,#18574,.F.) ;
#25830=ORIENTED_EDGE('',*,*,#18572,.F.) ;
#25831=ORIENTED_EDGE('',*,*,#17596,.F.) ;
#25832=ORIENTED_EDGE('',*,*,#18571,.F.) ;
#25833=ORIENTED_EDGE('',*,*,#18575,.F.) ;
#25834=ORIENTED_EDGE('',*,*,#18565,.F.) ;
#25835=ORIENTED_EDGE('',*,*,#18576,.F.) ;
#25836=ORIENTED_EDGE('',*,*,#18577,.F.) ;
#25837=ORIENTED_EDGE('',*,*,#17592,.F.) ;
#25838=ORIENTED_EDGE('',*,*,#18564,.F.) ;
#25839=ORIENTED_EDGE('',*,*,#18578,.F.) ;
#25840=ORIENTED_EDGE('',*,*,#18559,.F.) ;
#25841=ORIENTED_EDGE('',*,*,#18579,.F.) ;
#25842=ORIENTED_EDGE('',*,*,#18563,.F.) ;
#25843=ORIENTED_EDGE('',*,*,#17601,.F.) ;
#25844=ORIENTED_EDGE('',*,*,#18573,.T.) ;
#25845=ORIENTED_EDGE('',*,*,#18580,.F.) ;
#25846=ORIENTED_EDGE('',*,*,#18555,.T.) ;
#25847=ORIENTED_EDGE('',*,*,#18557,.T.) ;
#25848=ORIENTED_EDGE('',*,*,#18162,.F.) ;
#25849=ORIENTED_EDGE('',*,*,#18569,.T.) ;
#25850=ORIENTED_EDGE('',*,*,#18581,.F.) ;
#25851=ORIENTED_EDGE('',*,*,#18582,.F.) ;
#25852=ORIENTED_EDGE('',*,*,#18583,.F.) ;
#25853=ORIENTED_EDGE('',*,*,#18174,.F.) ;
#25854=ORIENTED_EDGE('',*,*,#18581,.T.) ;
#25855=ORIENTED_EDGE('',*,*,#18584,.F.) ;
#25856=ORIENTED_EDGE('',*,*,#18577,.T.) ;
#25857=ORIENTED_EDGE('',*,*,#18561,.T.) ;
#25858=ORIENTED_EDGE('',*,*,#18172,.F.) ;
#25859=ORIENTED_EDGE('',*,*,#18583,.T.) ;
#25860=ORIENTED_EDGE('',*,*,#17581,.F.) ;
#25861=ORIENTED_EDGE('',*,*,#17589,.T.) ;
#25862=ORIENTED_EDGE('',*,*,#18576,.T.) ;
#25863=ORIENTED_EDGE('',*,*,#18568,.T.) ;
#25864=ORIENTED_EDGE('',*,*,#18558,.T.) ;
#25865=ORIENTED_EDGE('',*,*,#18570,.T.) ;
#25866=ORIENTED_EDGE('',*,*,#18575,.T.) ;
#25867=ORIENTED_EDGE('',*,*,#18574,.T.) ;
#25868=ORIENTED_EDGE('',*,*,#18578,.T.) ;
#25869=ORIENTED_EDGE('',*,*,#18579,.T.) ;
#25870=ORIENTED_EDGE('',*,*,#18562,.T.) ;
#25871=ORIENTED_EDGE('',*,*,#18582,.T.) ;
#25872=ORIENTED_EDGE('',*,*,#18585,.T.) ;
#25873=ORIENTED_EDGE('',*,*,#18586,.T.) ;
#25874=ORIENTED_EDGE('',*,*,#18587,.T.) ;
#25875=ORIENTED_EDGE('',*,*,#18588,.T.) ;
#25876=ORIENTED_EDGE('',*,*,#18589,.T.) ;
#25877=ORIENTED_EDGE('',*,*,#18590,.T.) ;
#25878=ORIENTED_EDGE('',*,*,#18591,.F.) ;
#25879=ORIENTED_EDGE('',*,*,#18592,.T.) ;
#25880=ORIENTED_EDGE('',*,*,#18593,.T.) ;
#25881=ORIENTED_EDGE('',*,*,#18594,.F.) ;
#25882=ORIENTED_EDGE('',*,*,#18595,.F.) ;
#25883=ORIENTED_EDGE('',*,*,#18590,.F.) ;
#25884=ORIENTED_EDGE('',*,*,#18585,.F.) ;
#25885=ORIENTED_EDGE('',*,*,#18592,.F.) ;
#25886=ORIENTED_EDGE('',*,*,#18593,.F.) ;
#25887=ORIENTED_EDGE('',*,*,#18588,.F.) ;
#25888=ORIENTED_EDGE('',*,*,#18596,.F.) ;
#25889=ORIENTED_EDGE('',*,*,#17890,.F.) ;
#25890=ORIENTED_EDGE('',*,*,#18589,.F.) ;
#25891=ORIENTED_EDGE('',*,*,#18597,.F.) ;
#25892=ORIENTED_EDGE('',*,*,#18598,.F.) ;
#25893=ORIENTED_EDGE('',*,*,#18586,.F.) ;
#25894=ORIENTED_EDGE('',*,*,#18587,.F.) ;
#25895=ORIENTED_EDGE('',*,*,#18599,.F.) ;
#25896=ORIENTED_EDGE('',*,*,#17886,.F.) ;
#25897=ORIENTED_EDGE('',*,*,#18600,.F.) ;
#25898=ORIENTED_EDGE('',*,*,#18598,.T.) ;
#25899=ORIENTED_EDGE('',*,*,#17883,.T.) ;
#25900=ORIENTED_EDGE('',*,*,#18599,.T.) ;
#25901=ORIENTED_EDGE('',*,*,#17888,.T.) ;
#25902=ORIENTED_EDGE('',*,*,#18596,.T.) ;
#25903=ORIENTED_EDGE('',*,*,#18600,.T.) ;
#25904=ORIENTED_EDGE('',*,*,#17555,.F.) ;
#25905=ORIENTED_EDGE('',*,*,#18133,.F.) ;
#25906=ORIENTED_EDGE('',*,*,#18601,.F.) ;
#25907=ORIENTED_EDGE('',*,*,#17569,.F.) ;
#25908=ORIENTED_EDGE('',*,*,#18602,.F.) ;
#25909=ORIENTED_EDGE('',*,*,#18603,.F.) ;
#25910=ORIENTED_EDGE('',*,*,#18604,.F.) ;
#25911=ORIENTED_EDGE('',*,*,#18605,.F.) ;
#25912=ORIENTED_EDGE('',*,*,#18606,.T.) ;
#25913=ORIENTED_EDGE('',*,*,#18601,.T.) ;
#25914=ORIENTED_EDGE('',*,*,#18132,.F.) ;
#25915=ORIENTED_EDGE('',*,*,#18607,.T.) ;
#25916=ORIENTED_EDGE('',*,*,#18608,.F.) ;
#25917=ORIENTED_EDGE('',*,*,#18609,.F.) ;
#25918=ORIENTED_EDGE('',*,*,#18607,.F.) ;
#25919=ORIENTED_EDGE('',*,*,#18131,.F.) ;
#25920=ORIENTED_EDGE('',*,*,#18610,.T.) ;
#25921=ORIENTED_EDGE('',*,*,#18611,.T.) ;
#25922=ORIENTED_EDGE('',*,*,#17560,.F.) ;
#25923=ORIENTED_EDGE('',*,*,#17568,.T.) ;
#25924=ORIENTED_EDGE('',*,*,#18612,.T.) ;
#25925=ORIENTED_EDGE('',*,*,#18613,.T.) ;
#25926=ORIENTED_EDGE('',*,*,#18128,.F.) ;
#25927=ORIENTED_EDGE('',*,*,#18614,.T.) ;
#25928=ORIENTED_EDGE('',*,*,#17552,.T.) ;
#25929=ORIENTED_EDGE('',*,*,#18615,.F.) ;
#25930=ORIENTED_EDGE('',*,*,#18614,.F.) ;
#25931=ORIENTED_EDGE('',*,*,#18127,.F.) ;
#25932=ORIENTED_EDGE('',*,*,#18616,.F.) ;
#25933=ORIENTED_EDGE('',*,*,#18129,.F.) ;
#25934=ORIENTED_EDGE('',*,*,#18613,.F.) ;
#25935=ORIENTED_EDGE('',*,*,#18617,.F.) ;
#25936=ORIENTED_EDGE('',*,*,#18618,.T.) ;
#25937=ORIENTED_EDGE('',*,*,#17557,.T.) ;
#25938=ORIENTED_EDGE('',*,*,#17566,.F.) ;
#25939=ORIENTED_EDGE('',*,*,#18619,.T.) ;
#25940=ORIENTED_EDGE('',*,*,#18620,.F.) ;
#25941=ORIENTED_EDGE('',*,*,#18621,.F.) ;
#25942=ORIENTED_EDGE('',*,*,#18619,.F.) ;
#25943=ORIENTED_EDGE('',*,*,#17565,.F.) ;
#25944=ORIENTED_EDGE('',*,*,#18618,.F.) ;
#25945=ORIENTED_EDGE('',*,*,#18622,.F.) ;
#25946=ORIENTED_EDGE('',*,*,#18612,.F.) ;
#25947=ORIENTED_EDGE('',*,*,#18623,.F.) ;
#25948=ORIENTED_EDGE('',*,*,#18624,.F.) ;
#25949=ORIENTED_EDGE('',*,*,#17561,.F.) ;
#25950=ORIENTED_EDGE('',*,*,#18611,.F.) ;
#25951=ORIENTED_EDGE('',*,*,#18625,.F.) ;
#25952=ORIENTED_EDGE('',*,*,#18606,.F.) ;
#25953=ORIENTED_EDGE('',*,*,#18626,.F.) ;
#25954=ORIENTED_EDGE('',*,*,#18610,.F.) ;
#25955=ORIENTED_EDGE('',*,*,#17570,.F.) ;
#25956=ORIENTED_EDGE('',*,*,#18620,.T.) ;
#25957=ORIENTED_EDGE('',*,*,#18627,.F.) ;
#25958=ORIENTED_EDGE('',*,*,#18602,.T.) ;
#25959=ORIENTED_EDGE('',*,*,#18604,.T.) ;
#25960=ORIENTED_EDGE('',*,*,#18125,.F.) ;
#25961=ORIENTED_EDGE('',*,*,#18616,.T.) ;
#25962=ORIENTED_EDGE('',*,*,#18628,.F.) ;
#25963=ORIENTED_EDGE('',*,*,#18629,.F.) ;
#25964=ORIENTED_EDGE('',*,*,#18630,.F.) ;
#25965=ORIENTED_EDGE('',*,*,#18137,.F.) ;
#25966=ORIENTED_EDGE('',*,*,#18628,.T.) ;
#25967=ORIENTED_EDGE('',*,*,#18631,.F.) ;
#25968=ORIENTED_EDGE('',*,*,#18624,.T.) ;
#25969=ORIENTED_EDGE('',*,*,#18608,.T.) ;
#25970=ORIENTED_EDGE('',*,*,#18135,.F.) ;
#25971=ORIENTED_EDGE('',*,*,#18630,.T.) ;
#25972=ORIENTED_EDGE('',*,*,#17550,.F.) ;
#25973=ORIENTED_EDGE('',*,*,#17558,.T.) ;
#25974=ORIENTED_EDGE('',*,*,#18623,.T.) ;
#25975=ORIENTED_EDGE('',*,*,#18615,.T.) ;
#25976=ORIENTED_EDGE('',*,*,#18605,.T.) ;
#25977=ORIENTED_EDGE('',*,*,#18617,.T.) ;
#25978=ORIENTED_EDGE('',*,*,#18622,.T.) ;
#25979=ORIENTED_EDGE('',*,*,#18621,.T.) ;
#25980=ORIENTED_EDGE('',*,*,#18625,.T.) ;
#25981=ORIENTED_EDGE('',*,*,#18626,.T.) ;
#25982=ORIENTED_EDGE('',*,*,#18609,.T.) ;
#25983=ORIENTED_EDGE('',*,*,#18629,.T.) ;
#25984=ORIENTED_EDGE('',*,*,#18632,.T.) ;
#25985=ORIENTED_EDGE('',*,*,#18633,.T.) ;
#25986=ORIENTED_EDGE('',*,*,#18634,.T.) ;
#25987=ORIENTED_EDGE('',*,*,#18635,.T.) ;
#25988=ORIENTED_EDGE('',*,*,#18636,.T.) ;
#25989=ORIENTED_EDGE('',*,*,#18637,.T.) ;
#25990=ORIENTED_EDGE('',*,*,#18638,.F.) ;
#25991=ORIENTED_EDGE('',*,*,#18639,.T.) ;
#25992=ORIENTED_EDGE('',*,*,#18640,.T.) ;
#25993=ORIENTED_EDGE('',*,*,#18641,.F.) ;
#25994=ORIENTED_EDGE('',*,*,#18642,.F.) ;
#25995=ORIENTED_EDGE('',*,*,#18637,.F.) ;
#25996=ORIENTED_EDGE('',*,*,#18632,.F.) ;
#25997=ORIENTED_EDGE('',*,*,#18639,.F.) ;
#25998=ORIENTED_EDGE('',*,*,#18640,.F.) ;
#25999=ORIENTED_EDGE('',*,*,#18635,.F.) ;
#26000=ORIENTED_EDGE('',*,*,#18643,.F.) ;
#26001=ORIENTED_EDGE('',*,*,#17857,.F.) ;
#26002=ORIENTED_EDGE('',*,*,#18636,.F.) ;
#26003=ORIENTED_EDGE('',*,*,#18644,.F.) ;
#26004=ORIENTED_EDGE('',*,*,#18645,.F.) ;
#26005=ORIENTED_EDGE('',*,*,#18633,.F.) ;
#26006=ORIENTED_EDGE('',*,*,#18634,.F.) ;
#26007=ORIENTED_EDGE('',*,*,#18646,.F.) ;
#26008=ORIENTED_EDGE('',*,*,#17853,.F.) ;
#26009=ORIENTED_EDGE('',*,*,#18647,.F.) ;
#26010=ORIENTED_EDGE('',*,*,#18645,.T.) ;
#26011=ORIENTED_EDGE('',*,*,#17850,.T.) ;
#26012=ORIENTED_EDGE('',*,*,#18646,.T.) ;
#26013=ORIENTED_EDGE('',*,*,#17855,.T.) ;
#26014=ORIENTED_EDGE('',*,*,#18643,.T.) ;
#26015=ORIENTED_EDGE('',*,*,#18647,.T.) ;
#26016=ORIENTED_EDGE('',*,*,#17524,.F.) ;
#26017=ORIENTED_EDGE('',*,*,#18096,.F.) ;
#26018=ORIENTED_EDGE('',*,*,#18648,.F.) ;
#26019=ORIENTED_EDGE('',*,*,#17538,.F.) ;
#26020=ORIENTED_EDGE('',*,*,#18649,.F.) ;
#26021=ORIENTED_EDGE('',*,*,#18650,.F.) ;
#26022=ORIENTED_EDGE('',*,*,#18651,.F.) ;
#26023=ORIENTED_EDGE('',*,*,#18652,.F.) ;
#26024=ORIENTED_EDGE('',*,*,#18653,.T.) ;
#26025=ORIENTED_EDGE('',*,*,#18648,.T.) ;
#26026=ORIENTED_EDGE('',*,*,#18095,.F.) ;
#26027=ORIENTED_EDGE('',*,*,#18654,.T.) ;
#26028=ORIENTED_EDGE('',*,*,#18655,.F.) ;
#26029=ORIENTED_EDGE('',*,*,#18656,.F.) ;
#26030=ORIENTED_EDGE('',*,*,#18654,.F.) ;
#26031=ORIENTED_EDGE('',*,*,#18094,.F.) ;
#26032=ORIENTED_EDGE('',*,*,#18657,.T.) ;
#26033=ORIENTED_EDGE('',*,*,#18658,.T.) ;
#26034=ORIENTED_EDGE('',*,*,#17529,.F.) ;
#26035=ORIENTED_EDGE('',*,*,#17537,.T.) ;
#26036=ORIENTED_EDGE('',*,*,#18659,.T.) ;
#26037=ORIENTED_EDGE('',*,*,#18660,.T.) ;
#26038=ORIENTED_EDGE('',*,*,#18091,.F.) ;
#26039=ORIENTED_EDGE('',*,*,#18661,.T.) ;
#26040=ORIENTED_EDGE('',*,*,#17521,.T.) ;
#26041=ORIENTED_EDGE('',*,*,#18662,.F.) ;
#26042=ORIENTED_EDGE('',*,*,#18661,.F.) ;
#26043=ORIENTED_EDGE('',*,*,#18090,.F.) ;
#26044=ORIENTED_EDGE('',*,*,#18663,.F.) ;
#26045=ORIENTED_EDGE('',*,*,#18092,.F.) ;
#26046=ORIENTED_EDGE('',*,*,#18660,.F.) ;
#26047=ORIENTED_EDGE('',*,*,#18664,.F.) ;
#26048=ORIENTED_EDGE('',*,*,#18665,.T.) ;
#26049=ORIENTED_EDGE('',*,*,#17526,.T.) ;
#26050=ORIENTED_EDGE('',*,*,#17535,.F.) ;
#26051=ORIENTED_EDGE('',*,*,#18666,.T.) ;
#26052=ORIENTED_EDGE('',*,*,#18667,.F.) ;
#26053=ORIENTED_EDGE('',*,*,#18668,.F.) ;
#26054=ORIENTED_EDGE('',*,*,#18666,.F.) ;
#26055=ORIENTED_EDGE('',*,*,#17534,.F.) ;
#26056=ORIENTED_EDGE('',*,*,#18665,.F.) ;
#26057=ORIENTED_EDGE('',*,*,#18669,.F.) ;
#26058=ORIENTED_EDGE('',*,*,#18659,.F.) ;
#26059=ORIENTED_EDGE('',*,*,#18670,.F.) ;
#26060=ORIENTED_EDGE('',*,*,#18671,.F.) ;
#26061=ORIENTED_EDGE('',*,*,#17530,.F.) ;
#26062=ORIENTED_EDGE('',*,*,#18658,.F.) ;
#26063=ORIENTED_EDGE('',*,*,#18672,.F.) ;
#26064=ORIENTED_EDGE('',*,*,#18653,.F.) ;
#26065=ORIENTED_EDGE('',*,*,#18673,.F.) ;
#26066=ORIENTED_EDGE('',*,*,#18657,.F.) ;
#26067=ORIENTED_EDGE('',*,*,#17539,.F.) ;
#26068=ORIENTED_EDGE('',*,*,#18667,.T.) ;
#26069=ORIENTED_EDGE('',*,*,#18674,.F.) ;
#26070=ORIENTED_EDGE('',*,*,#18649,.T.) ;
#26071=ORIENTED_EDGE('',*,*,#18651,.T.) ;
#26072=ORIENTED_EDGE('',*,*,#18088,.F.) ;
#26073=ORIENTED_EDGE('',*,*,#18663,.T.) ;
#26074=ORIENTED_EDGE('',*,*,#18675,.F.) ;
#26075=ORIENTED_EDGE('',*,*,#18676,.F.) ;
#26076=ORIENTED_EDGE('',*,*,#18677,.F.) ;
#26077=ORIENTED_EDGE('',*,*,#18100,.F.) ;
#26078=ORIENTED_EDGE('',*,*,#18675,.T.) ;
#26079=ORIENTED_EDGE('',*,*,#18678,.F.) ;
#26080=ORIENTED_EDGE('',*,*,#18671,.T.) ;
#26081=ORIENTED_EDGE('',*,*,#18655,.T.) ;
#26082=ORIENTED_EDGE('',*,*,#18098,.F.) ;
#26083=ORIENTED_EDGE('',*,*,#18677,.T.) ;
#26084=ORIENTED_EDGE('',*,*,#17519,.F.) ;
#26085=ORIENTED_EDGE('',*,*,#17527,.T.) ;
#26086=ORIENTED_EDGE('',*,*,#18670,.T.) ;
#26087=ORIENTED_EDGE('',*,*,#18662,.T.) ;
#26088=ORIENTED_EDGE('',*,*,#18652,.T.) ;
#26089=ORIENTED_EDGE('',*,*,#18664,.T.) ;
#26090=ORIENTED_EDGE('',*,*,#18669,.T.) ;
#26091=ORIENTED_EDGE('',*,*,#18668,.T.) ;
#26092=ORIENTED_EDGE('',*,*,#18672,.T.) ;
#26093=ORIENTED_EDGE('',*,*,#18673,.T.) ;
#26094=ORIENTED_EDGE('',*,*,#18656,.T.) ;
#26095=ORIENTED_EDGE('',*,*,#18676,.T.) ;
#26096=ORIENTED_EDGE('',*,*,#18679,.T.) ;
#26097=ORIENTED_EDGE('',*,*,#18680,.T.) ;
#26098=ORIENTED_EDGE('',*,*,#18681,.T.) ;
#26099=ORIENTED_EDGE('',*,*,#18682,.T.) ;
#26100=ORIENTED_EDGE('',*,*,#18683,.T.) ;
#26101=ORIENTED_EDGE('',*,*,#18684,.T.) ;
#26102=ORIENTED_EDGE('',*,*,#18685,.F.) ;
#26103=ORIENTED_EDGE('',*,*,#18686,.T.) ;
#26104=ORIENTED_EDGE('',*,*,#18687,.T.) ;
#26105=ORIENTED_EDGE('',*,*,#18688,.F.) ;
#26106=ORIENTED_EDGE('',*,*,#18689,.F.) ;
#26107=ORIENTED_EDGE('',*,*,#18684,.F.) ;
#26108=ORIENTED_EDGE('',*,*,#18679,.F.) ;
#26109=ORIENTED_EDGE('',*,*,#18686,.F.) ;
#26110=ORIENTED_EDGE('',*,*,#18687,.F.) ;
#26111=ORIENTED_EDGE('',*,*,#18682,.F.) ;
#26112=ORIENTED_EDGE('',*,*,#18690,.F.) ;
#26113=ORIENTED_EDGE('',*,*,#17824,.F.) ;
#26114=ORIENTED_EDGE('',*,*,#18683,.F.) ;
#26115=ORIENTED_EDGE('',*,*,#18691,.F.) ;
#26116=ORIENTED_EDGE('',*,*,#18692,.F.) ;
#26117=ORIENTED_EDGE('',*,*,#18680,.F.) ;
#26118=ORIENTED_EDGE('',*,*,#18681,.F.) ;
#26119=ORIENTED_EDGE('',*,*,#18693,.F.) ;
#26120=ORIENTED_EDGE('',*,*,#17820,.F.) ;
#26121=ORIENTED_EDGE('',*,*,#18694,.F.) ;
#26122=ORIENTED_EDGE('',*,*,#18692,.T.) ;
#26123=ORIENTED_EDGE('',*,*,#17817,.T.) ;
#26124=ORIENTED_EDGE('',*,*,#18693,.T.) ;
#26125=ORIENTED_EDGE('',*,*,#17822,.T.) ;
#26126=ORIENTED_EDGE('',*,*,#18690,.T.) ;
#26127=ORIENTED_EDGE('',*,*,#18694,.T.) ;
#26128=ORIENTED_EDGE('',*,*,#17493,.F.) ;
#26129=ORIENTED_EDGE('',*,*,#18059,.F.) ;
#26130=ORIENTED_EDGE('',*,*,#18695,.F.) ;
#26131=ORIENTED_EDGE('',*,*,#17507,.F.) ;
#26132=ORIENTED_EDGE('',*,*,#18696,.F.) ;
#26133=ORIENTED_EDGE('',*,*,#18697,.F.) ;
#26134=ORIENTED_EDGE('',*,*,#18698,.F.) ;
#26135=ORIENTED_EDGE('',*,*,#18699,.F.) ;
#26136=ORIENTED_EDGE('',*,*,#18700,.T.) ;
#26137=ORIENTED_EDGE('',*,*,#18695,.T.) ;
#26138=ORIENTED_EDGE('',*,*,#18058,.F.) ;
#26139=ORIENTED_EDGE('',*,*,#18701,.T.) ;
#26140=ORIENTED_EDGE('',*,*,#18702,.F.) ;
#26141=ORIENTED_EDGE('',*,*,#18703,.F.) ;
#26142=ORIENTED_EDGE('',*,*,#18701,.F.) ;
#26143=ORIENTED_EDGE('',*,*,#18057,.F.) ;
#26144=ORIENTED_EDGE('',*,*,#18704,.T.) ;
#26145=ORIENTED_EDGE('',*,*,#18705,.T.) ;
#26146=ORIENTED_EDGE('',*,*,#17498,.F.) ;
#26147=ORIENTED_EDGE('',*,*,#17506,.T.) ;
#26148=ORIENTED_EDGE('',*,*,#18706,.T.) ;
#26149=ORIENTED_EDGE('',*,*,#18707,.T.) ;
#26150=ORIENTED_EDGE('',*,*,#18054,.F.) ;
#26151=ORIENTED_EDGE('',*,*,#18708,.T.) ;
#26152=ORIENTED_EDGE('',*,*,#17490,.T.) ;
#26153=ORIENTED_EDGE('',*,*,#18709,.F.) ;
#26154=ORIENTED_EDGE('',*,*,#18708,.F.) ;
#26155=ORIENTED_EDGE('',*,*,#18053,.F.) ;
#26156=ORIENTED_EDGE('',*,*,#18710,.F.) ;
#26157=ORIENTED_EDGE('',*,*,#18055,.F.) ;
#26158=ORIENTED_EDGE('',*,*,#18707,.F.) ;
#26159=ORIENTED_EDGE('',*,*,#18711,.F.) ;
#26160=ORIENTED_EDGE('',*,*,#18712,.T.) ;
#26161=ORIENTED_EDGE('',*,*,#17495,.T.) ;
#26162=ORIENTED_EDGE('',*,*,#17504,.F.) ;
#26163=ORIENTED_EDGE('',*,*,#18713,.T.) ;
#26164=ORIENTED_EDGE('',*,*,#18714,.F.) ;
#26165=ORIENTED_EDGE('',*,*,#18715,.F.) ;
#26166=ORIENTED_EDGE('',*,*,#18713,.F.) ;
#26167=ORIENTED_EDGE('',*,*,#17503,.F.) ;
#26168=ORIENTED_EDGE('',*,*,#18712,.F.) ;
#26169=ORIENTED_EDGE('',*,*,#18716,.F.) ;
#26170=ORIENTED_EDGE('',*,*,#18706,.F.) ;
#26171=ORIENTED_EDGE('',*,*,#18717,.F.) ;
#26172=ORIENTED_EDGE('',*,*,#18718,.F.) ;
#26173=ORIENTED_EDGE('',*,*,#17499,.F.) ;
#26174=ORIENTED_EDGE('',*,*,#18705,.F.) ;
#26175=ORIENTED_EDGE('',*,*,#18719,.F.) ;
#26176=ORIENTED_EDGE('',*,*,#18700,.F.) ;
#26177=ORIENTED_EDGE('',*,*,#18720,.F.) ;
#26178=ORIENTED_EDGE('',*,*,#18704,.F.) ;
#26179=ORIENTED_EDGE('',*,*,#17508,.F.) ;
#26180=ORIENTED_EDGE('',*,*,#18714,.T.) ;
#26181=ORIENTED_EDGE('',*,*,#18721,.F.) ;
#26182=ORIENTED_EDGE('',*,*,#18696,.T.) ;
#26183=ORIENTED_EDGE('',*,*,#18698,.T.) ;
#26184=ORIENTED_EDGE('',*,*,#18051,.F.) ;
#26185=ORIENTED_EDGE('',*,*,#18710,.T.) ;
#26186=ORIENTED_EDGE('',*,*,#18722,.F.) ;
#26187=ORIENTED_EDGE('',*,*,#18723,.F.) ;
#26188=ORIENTED_EDGE('',*,*,#18724,.F.) ;
#26189=ORIENTED_EDGE('',*,*,#18063,.F.) ;
#26190=ORIENTED_EDGE('',*,*,#18722,.T.) ;
#26191=ORIENTED_EDGE('',*,*,#18725,.F.) ;
#26192=ORIENTED_EDGE('',*,*,#18718,.T.) ;
#26193=ORIENTED_EDGE('',*,*,#18702,.T.) ;
#26194=ORIENTED_EDGE('',*,*,#18061,.F.) ;
#26195=ORIENTED_EDGE('',*,*,#18724,.T.) ;
#26196=ORIENTED_EDGE('',*,*,#17488,.F.) ;
#26197=ORIENTED_EDGE('',*,*,#17496,.T.) ;
#26198=ORIENTED_EDGE('',*,*,#18717,.T.) ;
#26199=ORIENTED_EDGE('',*,*,#18709,.T.) ;
#26200=ORIENTED_EDGE('',*,*,#18699,.T.) ;
#26201=ORIENTED_EDGE('',*,*,#18711,.T.) ;
#26202=ORIENTED_EDGE('',*,*,#18716,.T.) ;
#26203=ORIENTED_EDGE('',*,*,#18715,.T.) ;
#26204=ORIENTED_EDGE('',*,*,#18719,.T.) ;
#26205=ORIENTED_EDGE('',*,*,#18720,.T.) ;
#26206=ORIENTED_EDGE('',*,*,#18703,.T.) ;
#26207=ORIENTED_EDGE('',*,*,#18723,.T.) ;
#26208=ORIENTED_EDGE('',*,*,#18726,.T.) ;
#26209=ORIENTED_EDGE('',*,*,#18727,.T.) ;
#26210=ORIENTED_EDGE('',*,*,#18728,.T.) ;
#26211=ORIENTED_EDGE('',*,*,#18729,.T.) ;
#26212=ORIENTED_EDGE('',*,*,#18730,.T.) ;
#26213=ORIENTED_EDGE('',*,*,#18731,.T.) ;
#26214=ORIENTED_EDGE('',*,*,#18732,.F.) ;
#26215=ORIENTED_EDGE('',*,*,#18733,.T.) ;
#26216=ORIENTED_EDGE('',*,*,#18734,.T.) ;
#26217=ORIENTED_EDGE('',*,*,#18735,.F.) ;
#26218=ORIENTED_EDGE('',*,*,#18736,.F.) ;
#26219=ORIENTED_EDGE('',*,*,#18731,.F.) ;
#26220=ORIENTED_EDGE('',*,*,#18726,.F.) ;
#26221=ORIENTED_EDGE('',*,*,#18733,.F.) ;
#26222=ORIENTED_EDGE('',*,*,#18734,.F.) ;
#26223=ORIENTED_EDGE('',*,*,#18729,.F.) ;
#26224=ORIENTED_EDGE('',*,*,#18737,.F.) ;
#26225=ORIENTED_EDGE('',*,*,#17791,.F.) ;
#26226=ORIENTED_EDGE('',*,*,#18730,.F.) ;
#26227=ORIENTED_EDGE('',*,*,#18738,.F.) ;
#26228=ORIENTED_EDGE('',*,*,#18739,.F.) ;
#26229=ORIENTED_EDGE('',*,*,#18727,.F.) ;
#26230=ORIENTED_EDGE('',*,*,#18728,.F.) ;
#26231=ORIENTED_EDGE('',*,*,#18740,.F.) ;
#26232=ORIENTED_EDGE('',*,*,#17787,.F.) ;
#26233=ORIENTED_EDGE('',*,*,#18741,.F.) ;
#26234=ORIENTED_EDGE('',*,*,#18739,.T.) ;
#26235=ORIENTED_EDGE('',*,*,#17784,.T.) ;
#26236=ORIENTED_EDGE('',*,*,#18740,.T.) ;
#26237=ORIENTED_EDGE('',*,*,#17789,.T.) ;
#26238=ORIENTED_EDGE('',*,*,#18737,.T.) ;
#26239=ORIENTED_EDGE('',*,*,#18741,.T.) ;
#26240=ORIENTED_EDGE('',*,*,#17462,.F.) ;
#26241=ORIENTED_EDGE('',*,*,#18022,.F.) ;
#26242=ORIENTED_EDGE('',*,*,#18742,.F.) ;
#26243=ORIENTED_EDGE('',*,*,#17476,.F.) ;
#26244=ORIENTED_EDGE('',*,*,#18743,.F.) ;
#26245=ORIENTED_EDGE('',*,*,#18744,.F.) ;
#26246=ORIENTED_EDGE('',*,*,#18745,.F.) ;
#26247=ORIENTED_EDGE('',*,*,#18746,.F.) ;
#26248=ORIENTED_EDGE('',*,*,#18747,.T.) ;
#26249=ORIENTED_EDGE('',*,*,#18742,.T.) ;
#26250=ORIENTED_EDGE('',*,*,#18021,.F.) ;
#26251=ORIENTED_EDGE('',*,*,#18748,.T.) ;
#26252=ORIENTED_EDGE('',*,*,#18749,.F.) ;
#26253=ORIENTED_EDGE('',*,*,#18750,.F.) ;
#26254=ORIENTED_EDGE('',*,*,#18748,.F.) ;
#26255=ORIENTED_EDGE('',*,*,#18020,.F.) ;
#26256=ORIENTED_EDGE('',*,*,#18751,.T.) ;
#26257=ORIENTED_EDGE('',*,*,#18752,.T.) ;
#26258=ORIENTED_EDGE('',*,*,#17467,.F.) ;
#26259=ORIENTED_EDGE('',*,*,#17475,.T.) ;
#26260=ORIENTED_EDGE('',*,*,#18753,.T.) ;
#26261=ORIENTED_EDGE('',*,*,#18754,.T.) ;
#26262=ORIENTED_EDGE('',*,*,#18017,.F.) ;
#26263=ORIENTED_EDGE('',*,*,#18755,.T.) ;
#26264=ORIENTED_EDGE('',*,*,#17459,.T.) ;
#26265=ORIENTED_EDGE('',*,*,#18756,.F.) ;
#26266=ORIENTED_EDGE('',*,*,#18755,.F.) ;
#26267=ORIENTED_EDGE('',*,*,#18016,.F.) ;
#26268=ORIENTED_EDGE('',*,*,#18757,.F.) ;
#26269=ORIENTED_EDGE('',*,*,#18018,.F.) ;
#26270=ORIENTED_EDGE('',*,*,#18754,.F.) ;
#26271=ORIENTED_EDGE('',*,*,#18758,.F.) ;
#26272=ORIENTED_EDGE('',*,*,#18759,.T.) ;
#26273=ORIENTED_EDGE('',*,*,#17464,.T.) ;
#26274=ORIENTED_EDGE('',*,*,#17473,.F.) ;
#26275=ORIENTED_EDGE('',*,*,#18760,.T.) ;
#26276=ORIENTED_EDGE('',*,*,#18761,.F.) ;
#26277=ORIENTED_EDGE('',*,*,#18762,.F.) ;
#26278=ORIENTED_EDGE('',*,*,#18760,.F.) ;
#26279=ORIENTED_EDGE('',*,*,#17472,.F.) ;
#26280=ORIENTED_EDGE('',*,*,#18759,.F.) ;
#26281=ORIENTED_EDGE('',*,*,#18763,.F.) ;
#26282=ORIENTED_EDGE('',*,*,#18753,.F.) ;
#26283=ORIENTED_EDGE('',*,*,#18764,.F.) ;
#26284=ORIENTED_EDGE('',*,*,#18765,.F.) ;
#26285=ORIENTED_EDGE('',*,*,#17468,.F.) ;
#26286=ORIENTED_EDGE('',*,*,#18752,.F.) ;
#26287=ORIENTED_EDGE('',*,*,#18766,.F.) ;
#26288=ORIENTED_EDGE('',*,*,#18747,.F.) ;
#26289=ORIENTED_EDGE('',*,*,#18767,.F.) ;
#26290=ORIENTED_EDGE('',*,*,#18751,.F.) ;
#26291=ORIENTED_EDGE('',*,*,#17477,.F.) ;
#26292=ORIENTED_EDGE('',*,*,#18761,.T.) ;
#26293=ORIENTED_EDGE('',*,*,#18768,.F.) ;
#26294=ORIENTED_EDGE('',*,*,#18743,.T.) ;
#26295=ORIENTED_EDGE('',*,*,#18745,.T.) ;
#26296=ORIENTED_EDGE('',*,*,#18014,.F.) ;
#26297=ORIENTED_EDGE('',*,*,#18757,.T.) ;
#26298=ORIENTED_EDGE('',*,*,#18769,.F.) ;
#26299=ORIENTED_EDGE('',*,*,#18770,.F.) ;
#26300=ORIENTED_EDGE('',*,*,#18771,.F.) ;
#26301=ORIENTED_EDGE('',*,*,#18026,.F.) ;
#26302=ORIENTED_EDGE('',*,*,#18769,.T.) ;
#26303=ORIENTED_EDGE('',*,*,#18772,.F.) ;
#26304=ORIENTED_EDGE('',*,*,#18765,.T.) ;
#26305=ORIENTED_EDGE('',*,*,#18749,.T.) ;
#26306=ORIENTED_EDGE('',*,*,#18024,.F.) ;
#26307=ORIENTED_EDGE('',*,*,#18771,.T.) ;
#26308=ORIENTED_EDGE('',*,*,#17457,.F.) ;
#26309=ORIENTED_EDGE('',*,*,#17465,.T.) ;
#26310=ORIENTED_EDGE('',*,*,#18764,.T.) ;
#26311=ORIENTED_EDGE('',*,*,#18756,.T.) ;
#26312=ORIENTED_EDGE('',*,*,#18746,.T.) ;
#26313=ORIENTED_EDGE('',*,*,#18758,.T.) ;
#26314=ORIENTED_EDGE('',*,*,#18763,.T.) ;
#26315=ORIENTED_EDGE('',*,*,#18762,.T.) ;
#26316=ORIENTED_EDGE('',*,*,#18766,.T.) ;
#26317=ORIENTED_EDGE('',*,*,#18767,.T.) ;
#26318=ORIENTED_EDGE('',*,*,#18750,.T.) ;
#26319=ORIENTED_EDGE('',*,*,#18770,.T.) ;
#26320=ORIENTED_EDGE('',*,*,#18773,.T.) ;
#26321=ORIENTED_EDGE('',*,*,#18774,.T.) ;
#26322=ORIENTED_EDGE('',*,*,#18775,.T.) ;
#26323=ORIENTED_EDGE('',*,*,#18776,.T.) ;
#26324=ORIENTED_EDGE('',*,*,#18777,.T.) ;
#26325=ORIENTED_EDGE('',*,*,#18778,.T.) ;
#26326=ORIENTED_EDGE('',*,*,#18779,.F.) ;
#26327=ORIENTED_EDGE('',*,*,#18780,.T.) ;
#26328=ORIENTED_EDGE('',*,*,#18781,.T.) ;
#26329=ORIENTED_EDGE('',*,*,#18782,.F.) ;
#26330=ORIENTED_EDGE('',*,*,#18783,.F.) ;
#26331=ORIENTED_EDGE('',*,*,#18778,.F.) ;
#26332=ORIENTED_EDGE('',*,*,#18773,.F.) ;
#26333=ORIENTED_EDGE('',*,*,#18780,.F.) ;
#26334=ORIENTED_EDGE('',*,*,#18781,.F.) ;
#26335=ORIENTED_EDGE('',*,*,#18776,.F.) ;
#26336=ORIENTED_EDGE('',*,*,#18784,.F.) ;
#26337=ORIENTED_EDGE('',*,*,#17758,.F.) ;
#26338=ORIENTED_EDGE('',*,*,#18777,.F.) ;
#26339=ORIENTED_EDGE('',*,*,#18785,.F.) ;
#26340=ORIENTED_EDGE('',*,*,#18786,.F.) ;
#26341=ORIENTED_EDGE('',*,*,#18774,.F.) ;
#26342=ORIENTED_EDGE('',*,*,#18775,.F.) ;
#26343=ORIENTED_EDGE('',*,*,#18787,.F.) ;
#26344=ORIENTED_EDGE('',*,*,#17754,.F.) ;
#26345=ORIENTED_EDGE('',*,*,#18788,.F.) ;
#26346=ORIENTED_EDGE('',*,*,#18786,.T.) ;
#26347=ORIENTED_EDGE('',*,*,#17751,.T.) ;
#26348=ORIENTED_EDGE('',*,*,#18787,.T.) ;
#26349=ORIENTED_EDGE('',*,*,#17756,.T.) ;
#26350=ORIENTED_EDGE('',*,*,#18784,.T.) ;
#26351=ORIENTED_EDGE('',*,*,#18788,.T.) ;
#26352=ORIENTED_EDGE('',*,*,#18789,.T.) ;
#26353=ORIENTED_EDGE('',*,*,#17293,.T.) ;
#26354=ORIENTED_EDGE('',*,*,#18790,.T.) ;
#26355=ORIENTED_EDGE('',*,*,#17247,.F.) ;
#26356=ORIENTED_EDGE('',*,*,#18791,.T.) ;
#26357=ORIENTED_EDGE('',*,*,#17251,.F.) ;
#26358=ORIENTED_EDGE('',*,*,#18792,.T.) ;
#26359=ORIENTED_EDGE('',*,*,#17310,.T.) ;
#26360=ORIENTED_EDGE('',*,*,#18793,.T.) ;
#26361=ORIENTED_EDGE('',*,*,#17255,.F.) ;
#26362=ORIENTED_EDGE('',*,*,#18794,.T.) ;
#26363=ORIENTED_EDGE('',*,*,#17327,.T.) ;
#26364=ORIENTED_EDGE('',*,*,#18795,.T.) ;
#26365=ORIENTED_EDGE('',*,*,#17259,.F.) ;
#26366=ORIENTED_EDGE('',*,*,#18796,.T.) ;
#26367=ORIENTED_EDGE('',*,*,#17344,.T.) ;
#26368=ORIENTED_EDGE('',*,*,#18797,.T.) ;
#26369=ORIENTED_EDGE('',*,*,#17263,.F.) ;
#26370=ORIENTED_EDGE('',*,*,#18798,.T.) ;
#26371=ORIENTED_EDGE('',*,*,#17359,.T.) ;
#26372=ORIENTED_EDGE('',*,*,#18799,.T.) ;
#26373=ORIENTED_EDGE('',*,*,#17267,.F.) ;
#26374=ORIENTED_EDGE('',*,*,#18800,.T.) ;
#26375=ORIENTED_EDGE('',*,*,#17376,.T.) ;
#26376=ORIENTED_EDGE('',*,*,#18801,.T.) ;
#26377=ORIENTED_EDGE('',*,*,#17271,.F.) ;
#26378=ORIENTED_EDGE('',*,*,#18802,.T.) ;
#26379=ORIENTED_EDGE('',*,*,#17393,.T.) ;
#26380=ORIENTED_EDGE('',*,*,#18803,.T.) ;
#26381=ORIENTED_EDGE('',*,*,#17275,.F.) ;
#26382=ORIENTED_EDGE('',*,*,#18804,.T.) ;
#26383=ORIENTED_EDGE('',*,*,#17410,.T.) ;
#26384=ORIENTED_EDGE('',*,*,#18805,.T.) ;
#26385=ORIENTED_EDGE('',*,*,#17279,.F.) ;
#26386=ORIENTED_EDGE('',*,*,#18806,.T.) ;
#26387=ORIENTED_EDGE('',*,*,#17425,.T.) ;
#26388=ORIENTED_EDGE('',*,*,#17256,.F.) ;
#26389=ORIENTED_EDGE('',*,*,#18793,.F.) ;
#26390=ORIENTED_EDGE('',*,*,#17326,.T.) ;
#26391=ORIENTED_EDGE('',*,*,#18807,.F.) ;
#26392=ORIENTED_EDGE('',*,*,#17254,.F.) ;
#26393=ORIENTED_EDGE('',*,*,#18808,.F.) ;
#26394=ORIENTED_EDGE('',*,*,#17328,.T.) ;
#26395=ORIENTED_EDGE('',*,*,#18794,.F.) ;
#26396=ORIENTED_EDGE('',*,*,#17270,.F.) ;
#26397=ORIENTED_EDGE('',*,*,#18809,.F.) ;
#26398=ORIENTED_EDGE('',*,*,#17394,.T.) ;
#26399=ORIENTED_EDGE('',*,*,#18802,.F.) ;
#26400=ORIENTED_EDGE('',*,*,#17272,.F.) ;
#26401=ORIENTED_EDGE('',*,*,#18801,.F.) ;
#26402=ORIENTED_EDGE('',*,*,#17396,.T.) ;
#26403=ORIENTED_EDGE('',*,*,#18810,.F.) ;
#26404=ORIENTED_EDGE('',*,*,#17274,.F.) ;
#26405=ORIENTED_EDGE('',*,*,#18811,.F.) ;
#26406=ORIENTED_EDGE('',*,*,#17411,.T.) ;
#26407=ORIENTED_EDGE('',*,*,#18804,.F.) ;
#26408=ORIENTED_EDGE('',*,*,#17276,.F.) ;
#26409=ORIENTED_EDGE('',*,*,#18803,.F.) ;
#26410=ORIENTED_EDGE('',*,*,#17413,.T.) ;
#26411=ORIENTED_EDGE('',*,*,#18812,.F.) ;
#26412=ORIENTED_EDGE('',*,*,#17260,.F.) ;
#26413=ORIENTED_EDGE('',*,*,#18795,.F.) ;
#26414=ORIENTED_EDGE('',*,*,#17343,.T.) ;
#26415=ORIENTED_EDGE('',*,*,#18813,.F.) ;
#26416=ORIENTED_EDGE('',*,*,#17258,.F.) ;
#26417=ORIENTED_EDGE('',*,*,#18814,.F.) ;
#26418=ORIENTED_EDGE('',*,*,#17345,.T.) ;
#26419=ORIENTED_EDGE('',*,*,#18796,.F.) ;
#26420=ORIENTED_EDGE('',*,*,#17252,.F.) ;
#26421=ORIENTED_EDGE('',*,*,#18791,.F.) ;
#26422=ORIENTED_EDGE('',*,*,#17309,.T.) ;
#26423=ORIENTED_EDGE('',*,*,#18815,.F.) ;
#26424=ORIENTED_EDGE('',*,*,#17250,.F.) ;
#26425=ORIENTED_EDGE('',*,*,#18816,.F.) ;
#26426=ORIENTED_EDGE('',*,*,#17311,.T.) ;
#26427=ORIENTED_EDGE('',*,*,#18792,.F.) ;
#26428=ORIENTED_EDGE('',*,*,#17266,.F.) ;
#26429=ORIENTED_EDGE('',*,*,#18817,.F.) ;
#26430=ORIENTED_EDGE('',*,*,#17377,.T.) ;
#26431=ORIENTED_EDGE('',*,*,#18800,.F.) ;
#26432=ORIENTED_EDGE('',*,*,#17268,.F.) ;
#26433=ORIENTED_EDGE('',*,*,#18799,.F.) ;
#26434=ORIENTED_EDGE('',*,*,#17379,.T.) ;
#26435=ORIENTED_EDGE('',*,*,#18818,.F.) ;
#26436=ORIENTED_EDGE('',*,*,#17278,.F.) ;
#26437=ORIENTED_EDGE('',*,*,#18819,.F.) ;
#26438=ORIENTED_EDGE('',*,*,#17426,.T.) ;
#26439=ORIENTED_EDGE('',*,*,#18806,.F.) ;
#26440=ORIENTED_EDGE('',*,*,#17280,.F.) ;
#26441=ORIENTED_EDGE('',*,*,#18805,.F.) ;
#26442=ORIENTED_EDGE('',*,*,#17428,.T.) ;
#26443=ORIENTED_EDGE('',*,*,#18820,.F.) ;
#26444=ORIENTED_EDGE('',*,*,#17262,.F.) ;
#26445=ORIENTED_EDGE('',*,*,#18821,.F.) ;
#26446=ORIENTED_EDGE('',*,*,#17360,.T.) ;
#26447=ORIENTED_EDGE('',*,*,#18798,.F.) ;
#26448=ORIENTED_EDGE('',*,*,#17264,.F.) ;
#26449=ORIENTED_EDGE('',*,*,#18797,.F.) ;
#26450=ORIENTED_EDGE('',*,*,#17362,.T.) ;
#26451=ORIENTED_EDGE('',*,*,#18822,.F.) ;
#26452=ORIENTED_EDGE('',*,*,#17248,.F.) ;
#26453=ORIENTED_EDGE('',*,*,#18790,.F.) ;
#26454=ORIENTED_EDGE('',*,*,#17292,.T.) ;
#26455=ORIENTED_EDGE('',*,*,#18823,.F.) ;
#26456=ORIENTED_EDGE('',*,*,#17246,.F.) ;
#26457=ORIENTED_EDGE('',*,*,#18824,.F.) ;
#26458=ORIENTED_EDGE('',*,*,#17294,.T.) ;
#26459=ORIENTED_EDGE('',*,*,#18789,.F.) ;
#26460=ORIENTED_EDGE('',*,*,#18825,.T.) ;
#26461=ORIENTED_EDGE('',*,*,#18826,.F.) ;
#26462=ORIENTED_EDGE('',*,*,#18827,.T.) ;
#26463=ORIENTED_EDGE('',*,*,#18828,.F.) ;
#26464=ORIENTED_EDGE('',*,*,#18829,.T.) ;
#26465=ORIENTED_EDGE('',*,*,#18830,.F.) ;
#26466=ORIENTED_EDGE('',*,*,#18831,.T.) ;
#26467=ORIENTED_EDGE('',*,*,#18832,.F.) ;
#26468=ORIENTED_EDGE('',*,*,#18833,.T.) ;
#26469=ORIENTED_EDGE('',*,*,#18834,.F.) ;
#26470=ORIENTED_EDGE('',*,*,#18835,.T.) ;
#26471=ORIENTED_EDGE('',*,*,#18836,.F.) ;
#26472=ORIENTED_EDGE('',*,*,#18837,.T.) ;
#26473=ORIENTED_EDGE('',*,*,#18838,.F.) ;
#26474=ORIENTED_EDGE('',*,*,#18839,.T.) ;
#26475=ORIENTED_EDGE('',*,*,#18840,.F.) ;
#26476=ORIENTED_EDGE('',*,*,#18841,.T.) ;
#26477=ORIENTED_EDGE('',*,*,#18842,.F.) ;
#26478=ORIENTED_EDGE('',*,*,#18843,.F.) ;
#26479=ORIENTED_EDGE('',*,*,#18844,.F.) ;
#26480=ORIENTED_EDGE('',*,*,#18845,.T.) ;
#26481=ORIENTED_EDGE('',*,*,#18846,.F.) ;
#26482=ORIENTED_EDGE('',*,*,#18847,.F.) ;
#26483=ORIENTED_EDGE('',*,*,#18848,.F.) ;
#26484=ORIENTED_EDGE('',*,*,#18849,.T.) ;
#26485=ORIENTED_EDGE('',*,*,#18850,.F.) ;
#26486=ORIENTED_EDGE('',*,*,#18851,.F.) ;
#26487=ORIENTED_EDGE('',*,*,#18852,.F.) ;
#26488=ORIENTED_EDGE('',*,*,#18853,.T.) ;
#26489=ORIENTED_EDGE('',*,*,#18854,.F.) ;
#26490=ORIENTED_EDGE('',*,*,#18855,.F.) ;
#26491=ORIENTED_EDGE('',*,*,#18856,.F.) ;
#26492=ORIENTED_EDGE('',*,*,#18857,.T.) ;
#26493=ORIENTED_EDGE('',*,*,#18858,.F.) ;
#26494=ORIENTED_EDGE('',*,*,#18859,.T.) ;
#26495=ORIENTED_EDGE('',*,*,#18860,.F.) ;
#26496=ORIENTED_EDGE('',*,*,#18861,.F.) ;
#26497=ORIENTED_EDGE('',*,*,#18862,.F.) ;
#26498=ORIENTED_EDGE('',*,*,#18863,.F.) ;
#26499=ORIENTED_EDGE('',*,*,#18864,.F.) ;
#26500=ORIENTED_EDGE('',*,*,#18826,.T.) ;
#26501=ORIENTED_EDGE('',*,*,#18865,.T.) ;
#26502=ORIENTED_EDGE('',*,*,#18866,.T.) ;
#26503=ORIENTED_EDGE('',*,*,#18867,.T.) ;
#26504=ORIENTED_EDGE('',*,*,#18825,.F.) ;
#26505=ORIENTED_EDGE('',*,*,#18868,.F.) ;
#26506=ORIENTED_EDGE('',*,*,#18319,.F.) ;
#26507=ORIENTED_EDGE('',*,*,#18869,.F.) ;
#26508=ORIENTED_EDGE('',*,*,#18870,.F.) ;
#26509=ORIENTED_EDGE('',*,*,#18865,.F.) ;
#26510=ORIENTED_EDGE('',*,*,#18871,.T.) ;
#26511=ORIENTED_EDGE('',*,*,#18872,.T.) ;
#26512=ORIENTED_EDGE('',*,*,#18830,.T.) ;
#26513=ORIENTED_EDGE('',*,*,#18873,.T.) ;
#26514=ORIENTED_EDGE('',*,*,#18834,.T.) ;
#26515=ORIENTED_EDGE('',*,*,#18874,.T.) ;
#26516=ORIENTED_EDGE('',*,*,#18875,.T.) ;
#26517=ORIENTED_EDGE('',*,*,#18876,.T.) ;
#26518=ORIENTED_EDGE('',*,*,#18838,.T.) ;
#26519=ORIENTED_EDGE('',*,*,#18877,.T.) ;
#26520=ORIENTED_EDGE('',*,*,#18878,.T.) ;
#26521=ORIENTED_EDGE('',*,*,#18879,.T.) ;
#26522=ORIENTED_EDGE('',*,*,#18880,.T.) ;
#26523=ORIENTED_EDGE('',*,*,#18881,.T.) ;
#26524=ORIENTED_EDGE('',*,*,#18842,.T.) ;
#26525=ORIENTED_EDGE('',*,*,#18882,.T.) ;
#26526=ORIENTED_EDGE('',*,*,#18883,.T.) ;
#26527=ORIENTED_EDGE('',*,*,#18884,.T.) ;
#26528=ORIENTED_EDGE('',*,*,#18846,.T.) ;
#26529=ORIENTED_EDGE('',*,*,#18885,.T.) ;
#26530=ORIENTED_EDGE('',*,*,#18886,.T.) ;
#26531=ORIENTED_EDGE('',*,*,#18887,.T.) ;
#26532=ORIENTED_EDGE('',*,*,#18850,.T.) ;
#26533=ORIENTED_EDGE('',*,*,#18888,.T.) ;
#26534=ORIENTED_EDGE('',*,*,#18854,.T.) ;
#26535=ORIENTED_EDGE('',*,*,#18889,.T.) ;
#26536=ORIENTED_EDGE('',*,*,#18890,.T.) ;
#26537=ORIENTED_EDGE('',*,*,#18891,.T.) ;
#26538=ORIENTED_EDGE('',*,*,#18892,.T.) ;
#26539=ORIENTED_EDGE('',*,*,#18893,.T.) ;
#26540=ORIENTED_EDGE('',*,*,#18858,.T.) ;
#26541=ORIENTED_EDGE('',*,*,#18894,.T.) ;
#26542=ORIENTED_EDGE('',*,*,#18863,.T.) ;
#26543=ORIENTED_EDGE('',*,*,#18895,.F.) ;
#26544=ORIENTED_EDGE('',*,*,#18896,.F.) ;
#26545=ORIENTED_EDGE('',*,*,#18897,.F.) ;
#26546=ORIENTED_EDGE('',*,*,#18321,.F.) ;
#26547=ORIENTED_EDGE('',*,*,#18898,.F.) ;
#26548=ORIENTED_EDGE('',*,*,#18899,.T.) ;
#26549=ORIENTED_EDGE('',*,*,#18895,.T.) ;
#26550=ORIENTED_EDGE('',*,*,#18862,.T.) ;
#26551=ORIENTED_EDGE('',*,*,#18900,.T.) ;
#26552=ORIENTED_EDGE('',*,*,#18897,.T.) ;
#26553=ORIENTED_EDGE('',*,*,#18901,.T.) ;
#26554=ORIENTED_EDGE('',*,*,#18869,.T.) ;
#26555=ORIENTED_EDGE('',*,*,#18322,.T.) ;
#26556=ORIENTED_EDGE('',*,*,#18902,.T.) ;
#26557=ORIENTED_EDGE('',*,*,#18903,.T.) ;
#26558=ORIENTED_EDGE('',*,*,#18904,.T.) ;
#26559=ORIENTED_EDGE('',*,*,#18905,.T.) ;
#26560=ORIENTED_EDGE('',*,*,#18906,.T.) ;
#26561=ORIENTED_EDGE('',*,*,#18907,.T.) ;
#26562=ORIENTED_EDGE('',*,*,#18908,.T.) ;
#26563=ORIENTED_EDGE('',*,*,#18909,.T.) ;
#26564=ORIENTED_EDGE('',*,*,#18910,.T.) ;
#26565=ORIENTED_EDGE('',*,*,#18911,.T.) ;
#26566=ORIENTED_EDGE('',*,*,#18912,.T.) ;
#26567=ORIENTED_EDGE('',*,*,#18913,.T.) ;
#26568=ORIENTED_EDGE('',*,*,#18914,.T.) ;
#26569=ORIENTED_EDGE('',*,*,#18915,.T.) ;
#26570=ORIENTED_EDGE('',*,*,#18916,.T.) ;
#26571=ORIENTED_EDGE('',*,*,#18917,.T.) ;
#26572=ORIENTED_EDGE('',*,*,#18918,.T.) ;
#26573=ORIENTED_EDGE('',*,*,#18919,.T.) ;
#26574=ORIENTED_EDGE('',*,*,#18920,.T.) ;
#26575=ORIENTED_EDGE('',*,*,#18921,.T.) ;
#26576=ORIENTED_EDGE('',*,*,#18922,.T.) ;
#26577=ORIENTED_EDGE('',*,*,#18923,.T.) ;
#26578=ORIENTED_EDGE('',*,*,#18924,.T.) ;
#26579=ORIENTED_EDGE('',*,*,#18925,.T.) ;
#26580=ORIENTED_EDGE('',*,*,#18926,.T.) ;
#26581=ORIENTED_EDGE('',*,*,#18927,.T.) ;
#26582=ORIENTED_EDGE('',*,*,#18928,.T.) ;
#26583=ORIENTED_EDGE('',*,*,#18929,.T.) ;
#26584=ORIENTED_EDGE('',*,*,#18930,.T.) ;
#26585=ORIENTED_EDGE('',*,*,#18931,.T.) ;
#26586=ORIENTED_EDGE('',*,*,#18932,.T.) ;
#26587=ORIENTED_EDGE('',*,*,#18933,.T.) ;
#26588=ORIENTED_EDGE('',*,*,#18934,.F.) ;
#26589=ORIENTED_EDGE('',*,*,#18900,.F.) ;
#26590=ORIENTED_EDGE('',*,*,#18861,.T.) ;
#26591=ORIENTED_EDGE('',*,*,#18935,.F.) ;
#26592=ORIENTED_EDGE('',*,*,#17282,.F.) ;
#26593=ORIENTED_EDGE('',*,*,#18827,.F.) ;
#26594=ORIENTED_EDGE('',*,*,#18867,.F.) ;
#26595=ORIENTED_EDGE('',*,*,#18936,.F.) ;
#26596=ORIENTED_EDGE('',*,*,#18902,.F.) ;
#26597=ORIENTED_EDGE('',*,*,#18937,.F.) ;
#26598=ORIENTED_EDGE('',*,*,#18938,.F.) ;
#26599=ORIENTED_EDGE('',*,*,#18829,.F.) ;
#26600=ORIENTED_EDGE('',*,*,#18939,.F.) ;
#26601=ORIENTED_EDGE('',*,*,#18940,.F.) ;
#26602=ORIENTED_EDGE('',*,*,#18904,.F.) ;
#26603=ORIENTED_EDGE('',*,*,#18941,.F.) ;
#26604=ORIENTED_EDGE('',*,*,#18873,.F.) ;
#26605=ORIENTED_EDGE('',*,*,#18831,.F.) ;
#26606=ORIENTED_EDGE('',*,*,#18872,.F.) ;
#26607=ORIENTED_EDGE('',*,*,#18942,.F.) ;
#26608=ORIENTED_EDGE('',*,*,#18906,.F.) ;
#26609=ORIENTED_EDGE('',*,*,#18943,.F.) ;
#26610=ORIENTED_EDGE('',*,*,#18944,.F.) ;
#26611=ORIENTED_EDGE('',*,*,#18833,.F.) ;
#26612=ORIENTED_EDGE('',*,*,#18945,.F.) ;
#26613=ORIENTED_EDGE('',*,*,#18946,.F.) ;
#26614=ORIENTED_EDGE('',*,*,#18908,.F.) ;
#26615=ORIENTED_EDGE('',*,*,#18947,.F.) ;
#26616=ORIENTED_EDGE('',*,*,#18874,.F.) ;
#26617=ORIENTED_EDGE('',*,*,#18835,.F.) ;
#26618=ORIENTED_EDGE('',*,*,#18876,.F.) ;
#26619=ORIENTED_EDGE('',*,*,#18948,.F.) ;
#26620=ORIENTED_EDGE('',*,*,#18910,.F.) ;
#26621=ORIENTED_EDGE('',*,*,#18949,.F.) ;
#26622=ORIENTED_EDGE('',*,*,#18950,.F.) ;
#26623=ORIENTED_EDGE('',*,*,#18837,.F.) ;
#26624=ORIENTED_EDGE('',*,*,#18951,.F.) ;
#26625=ORIENTED_EDGE('',*,*,#18952,.F.) ;
#26626=ORIENTED_EDGE('',*,*,#18912,.F.) ;
#26627=ORIENTED_EDGE('',*,*,#18953,.F.) ;
#26628=ORIENTED_EDGE('',*,*,#18877,.F.) ;
#26629=ORIENTED_EDGE('',*,*,#18839,.F.) ;
#26630=ORIENTED_EDGE('',*,*,#18879,.F.) ;
#26631=ORIENTED_EDGE('',*,*,#18954,.F.) ;
#26632=ORIENTED_EDGE('',*,*,#18914,.F.) ;
#26633=ORIENTED_EDGE('',*,*,#18955,.F.) ;
#26634=ORIENTED_EDGE('',*,*,#18956,.F.) ;
#26635=ORIENTED_EDGE('',*,*,#18841,.F.) ;
#26636=ORIENTED_EDGE('',*,*,#18957,.F.) ;
#26637=ORIENTED_EDGE('',*,*,#18958,.F.) ;
#26638=ORIENTED_EDGE('',*,*,#18916,.F.) ;
#26639=ORIENTED_EDGE('',*,*,#18959,.F.) ;
#26640=ORIENTED_EDGE('',*,*,#18882,.F.) ;
#26641=ORIENTED_EDGE('',*,*,#18843,.T.) ;
#26642=ORIENTED_EDGE('',*,*,#18881,.F.) ;
#26643=ORIENTED_EDGE('',*,*,#18960,.F.) ;
#26644=ORIENTED_EDGE('',*,*,#18918,.F.) ;
#26645=ORIENTED_EDGE('',*,*,#18961,.F.) ;
#26646=ORIENTED_EDGE('',*,*,#18962,.F.) ;
#26647=ORIENTED_EDGE('',*,*,#18845,.F.) ;
#26648=ORIENTED_EDGE('',*,*,#18963,.F.) ;
#26649=ORIENTED_EDGE('',*,*,#18964,.F.) ;
#26650=ORIENTED_EDGE('',*,*,#18920,.F.) ;
#26651=ORIENTED_EDGE('',*,*,#18965,.F.) ;
#26652=ORIENTED_EDGE('',*,*,#18885,.F.) ;
#26653=ORIENTED_EDGE('',*,*,#18847,.T.) ;
#26654=ORIENTED_EDGE('',*,*,#18884,.F.) ;
#26655=ORIENTED_EDGE('',*,*,#18966,.F.) ;
#26656=ORIENTED_EDGE('',*,*,#18922,.F.) ;
#26657=ORIENTED_EDGE('',*,*,#18967,.F.) ;
#26658=ORIENTED_EDGE('',*,*,#18968,.F.) ;
#26659=ORIENTED_EDGE('',*,*,#18849,.F.) ;
#26660=ORIENTED_EDGE('',*,*,#18969,.F.) ;
#26661=ORIENTED_EDGE('',*,*,#18970,.F.) ;
#26662=ORIENTED_EDGE('',*,*,#18924,.F.) ;
#26663=ORIENTED_EDGE('',*,*,#18971,.F.) ;
#26664=ORIENTED_EDGE('',*,*,#18888,.F.) ;
#26665=ORIENTED_EDGE('',*,*,#18851,.T.) ;
#26666=ORIENTED_EDGE('',*,*,#18887,.F.) ;
#26667=ORIENTED_EDGE('',*,*,#18972,.F.) ;
#26668=ORIENTED_EDGE('',*,*,#18926,.F.) ;
#26669=ORIENTED_EDGE('',*,*,#18973,.F.) ;
#26670=ORIENTED_EDGE('',*,*,#18974,.F.) ;
#26671=ORIENTED_EDGE('',*,*,#18853,.F.) ;
#26672=ORIENTED_EDGE('',*,*,#18975,.F.) ;
#26673=ORIENTED_EDGE('',*,*,#18976,.F.) ;
#26674=ORIENTED_EDGE('',*,*,#18928,.F.) ;
#26675=ORIENTED_EDGE('',*,*,#18977,.F.) ;
#26676=ORIENTED_EDGE('',*,*,#18889,.F.) ;
#26677=ORIENTED_EDGE('',*,*,#18855,.T.) ;
#26678=ORIENTED_EDGE('',*,*,#18891,.F.) ;
#26679=ORIENTED_EDGE('',*,*,#18978,.F.) ;
#26680=ORIENTED_EDGE('',*,*,#18930,.F.) ;
#26681=ORIENTED_EDGE('',*,*,#18979,.F.) ;
#26682=ORIENTED_EDGE('',*,*,#18980,.F.) ;
#26683=ORIENTED_EDGE('',*,*,#18857,.F.) ;
#26684=ORIENTED_EDGE('',*,*,#18981,.F.) ;
#26685=ORIENTED_EDGE('',*,*,#18982,.F.) ;
#26686=ORIENTED_EDGE('',*,*,#18932,.F.) ;
#26687=ORIENTED_EDGE('',*,*,#18983,.F.) ;
#26688=ORIENTED_EDGE('',*,*,#18894,.F.) ;
#26689=ORIENTED_EDGE('',*,*,#18868,.T.) ;
#26690=ORIENTED_EDGE('',*,*,#18864,.T.) ;
#26691=ORIENTED_EDGE('',*,*,#18898,.T.) ;
#26692=ORIENTED_EDGE('',*,*,#18320,.T.) ;
#26693=ORIENTED_EDGE('',*,*,#17145,.T.) ;
#26694=ORIENTED_EDGE('',*,*,#17285,.T.) ;
#26695=ORIENTED_EDGE('',*,*,#17186,.T.) ;
#26696=ORIENTED_EDGE('',*,*,#17182,.T.) ;
#26697=ORIENTED_EDGE('',*,*,#17189,.T.) ;
#26698=ORIENTED_EDGE('',*,*,#17284,.T.) ;
#26699=ORIENTED_EDGE('',*,*,#17230,.T.) ;
#26700=ORIENTED_EDGE('',*,*,#17226,.T.) ;
#26701=ORIENTED_EDGE('',*,*,#17233,.T.) ;
#26702=ORIENTED_EDGE('',*,*,#17283,.T.) ;
#26703=ORIENTED_EDGE('',*,*,#18935,.T.) ;
#26704=ORIENTED_EDGE('',*,*,#18860,.T.) ;
#26705=ORIENTED_EDGE('',*,*,#18984,.T.) ;
#26706=ORIENTED_EDGE('',*,*,#17243,.T.) ;
#26707=ORIENTED_EDGE('',*,*,#17211,.T.) ;
#26708=ORIENTED_EDGE('',*,*,#17208,.T.) ;
#26709=ORIENTED_EDGE('',*,*,#17204,.T.) ;
#26710=ORIENTED_EDGE('',*,*,#17242,.T.) ;
#26711=ORIENTED_EDGE('',*,*,#17167,.T.) ;
#26712=ORIENTED_EDGE('',*,*,#17164,.T.) ;
#26713=ORIENTED_EDGE('',*,*,#17160,.T.) ;
#26714=ORIENTED_EDGE('',*,*,#17241,.T.) ;
#26715=ORIENTED_EDGE('',*,*,#17153,.T.) ;
#26716=ORIENTED_EDGE('',*,*,#17149,.T.) ;
#26717=ORIENTED_EDGE('',*,*,#17156,.T.) ;
#26718=ORIENTED_EDGE('',*,*,#17240,.T.) ;
#26719=ORIENTED_EDGE('',*,*,#17197,.T.) ;
#26720=ORIENTED_EDGE('',*,*,#17193,.T.) ;
#26721=ORIENTED_EDGE('',*,*,#17200,.T.) ;
#26722=ORIENTED_EDGE('',*,*,#17239,.T.) ;
#26723=ORIENTED_EDGE('',*,*,#17219,.T.) ;
#26724=ORIENTED_EDGE('',*,*,#17215,.T.) ;
#26725=ORIENTED_EDGE('',*,*,#17222,.T.) ;
#26726=ORIENTED_EDGE('',*,*,#17238,.T.) ;
#26727=ORIENTED_EDGE('',*,*,#17175,.T.) ;
#26728=ORIENTED_EDGE('',*,*,#17171,.T.) ;
#26729=ORIENTED_EDGE('',*,*,#17178,.T.) ;
#26730=ORIENTED_EDGE('',*,*,#17237,.T.) ;
#26731=ORIENTED_EDGE('',*,*,#17142,.T.) ;
#26732=ORIENTED_EDGE('',*,*,#17138,.T.) ;
#26733=ORIENTED_EDGE('',*,*,#18938,.T.) ;
#26734=ORIENTED_EDGE('',*,*,#18985,.T.) ;
#26735=ORIENTED_EDGE('',*,*,#18939,.T.) ;
#26736=ORIENTED_EDGE('',*,*,#18828,.T.) ;
#26737=ORIENTED_EDGE('',*,*,#18944,.T.) ;
#26738=ORIENTED_EDGE('',*,*,#18986,.T.) ;
#26739=ORIENTED_EDGE('',*,*,#18945,.T.) ;
#26740=ORIENTED_EDGE('',*,*,#18832,.T.) ;
#26741=ORIENTED_EDGE('',*,*,#18950,.T.) ;
#26742=ORIENTED_EDGE('',*,*,#18987,.T.) ;
#26743=ORIENTED_EDGE('',*,*,#18951,.T.) ;
#26744=ORIENTED_EDGE('',*,*,#18836,.T.) ;
#26745=ORIENTED_EDGE('',*,*,#18956,.T.) ;
#26746=ORIENTED_EDGE('',*,*,#18988,.T.) ;
#26747=ORIENTED_EDGE('',*,*,#18957,.T.) ;
#26748=ORIENTED_EDGE('',*,*,#18840,.T.) ;
#26749=ORIENTED_EDGE('',*,*,#18962,.T.) ;
#26750=ORIENTED_EDGE('',*,*,#18989,.T.) ;
#26751=ORIENTED_EDGE('',*,*,#18963,.T.) ;
#26752=ORIENTED_EDGE('',*,*,#18844,.T.) ;
#26753=ORIENTED_EDGE('',*,*,#18968,.T.) ;
#26754=ORIENTED_EDGE('',*,*,#18990,.T.) ;
#26755=ORIENTED_EDGE('',*,*,#18969,.T.) ;
#26756=ORIENTED_EDGE('',*,*,#18848,.T.) ;
#26757=ORIENTED_EDGE('',*,*,#18974,.T.) ;
#26758=ORIENTED_EDGE('',*,*,#18991,.T.) ;
#26759=ORIENTED_EDGE('',*,*,#18975,.T.) ;
#26760=ORIENTED_EDGE('',*,*,#18852,.T.) ;
#26761=ORIENTED_EDGE('',*,*,#18980,.T.) ;
#26762=ORIENTED_EDGE('',*,*,#18992,.T.) ;
#26763=ORIENTED_EDGE('',*,*,#18981,.T.) ;
#26764=ORIENTED_EDGE('',*,*,#18856,.T.) ;
#26765=ORIENTED_EDGE('',*,*,#18979,.T.) ;
#26766=ORIENTED_EDGE('',*,*,#18933,.F.) ;
#26767=ORIENTED_EDGE('',*,*,#18982,.T.) ;
#26768=ORIENTED_EDGE('',*,*,#18992,.F.) ;
#26769=ORIENTED_EDGE('',*,*,#17729,.T.) ;
#26770=ORIENTED_EDGE('',*,*,#17731,.F.) ;
#26771=ORIENTED_EDGE('',*,*,#17734,.T.) ;
#26772=ORIENTED_EDGE('',*,*,#17737,.F.) ;
#26773=ORIENTED_EDGE('',*,*,#17740,.T.) ;
#26774=ORIENTED_EDGE('',*,*,#17743,.F.) ;
#26775=ORIENTED_EDGE('',*,*,#17746,.T.) ;
#26776=ORIENTED_EDGE('',*,*,#17748,.F.) ;
#26777=ORIENTED_EDGE('',*,*,#17993,.T.) ;
#26778=ORIENTED_EDGE('',*,*,#17995,.F.) ;
#26779=ORIENTED_EDGE('',*,*,#17998,.T.) ;
#26780=ORIENTED_EDGE('',*,*,#18001,.F.) ;
#26781=ORIENTED_EDGE('',*,*,#18004,.T.) ;
#26782=ORIENTED_EDGE('',*,*,#18007,.F.) ;
#26783=ORIENTED_EDGE('',*,*,#18010,.T.) ;
#26784=ORIENTED_EDGE('',*,*,#18011,.F.) ;
#26785=ORIENTED_EDGE('',*,*,#18993,.T.) ;
#26786=ORIENTED_EDGE('',*,*,#18994,.F.) ;
#26787=ORIENTED_EDGE('',*,*,#18995,.F.) ;
#26788=ORIENTED_EDGE('',*,*,#18996,.T.) ;
#26789=ORIENTED_EDGE('',*,*,#18993,.F.) ;
#26790=ORIENTED_EDGE('',*,*,#18996,.F.) ;
#26791=ORIENTED_EDGE('',*,*,#18997,.T.) ;
#26792=ORIENTED_EDGE('',*,*,#18998,.T.) ;
#26793=ORIENTED_EDGE('',*,*,#18994,.T.) ;
#26794=ORIENTED_EDGE('',*,*,#18995,.T.) ;
#26795=ORIENTED_EDGE('',*,*,#18998,.F.) ;
#26796=ORIENTED_EDGE('',*,*,#18997,.F.) ;
#26797=ORIENTED_EDGE('',*,*,#18999,.T.) ;
#26798=ORIENTED_EDGE('',*,*,#17439,.F.) ;
#26799=ORIENTED_EDGE('',*,*,#18999,.F.) ;
#26800=ORIENTED_EDGE('',*,*,#18005,.F.) ;
#26801=ORIENTED_EDGE('',*,*,#18015,.F.) ;
#26802=ORIENTED_EDGE('',*,*,#18744,.T.) ;
#26803=ORIENTED_EDGE('',*,*,#19000,.T.) ;
#26804=ORIENTED_EDGE('',*,*,#18008,.F.) ;
#26805=ORIENTED_EDGE('',*,*,#19000,.F.) ;
#26806=ORIENTED_EDGE('',*,*,#18768,.T.) ;
#26807=ORIENTED_EDGE('',*,*,#17471,.F.) ;
#26808=ORIENTED_EDGE('',*,*,#18973,.T.) ;
#26809=ORIENTED_EDGE('',*,*,#18929,.F.) ;
#26810=ORIENTED_EDGE('',*,*,#18976,.T.) ;
#26811=ORIENTED_EDGE('',*,*,#18991,.F.) ;
#26812=ORIENTED_EDGE('',*,*,#17762,.T.) ;
#26813=ORIENTED_EDGE('',*,*,#17764,.F.) ;
#26814=ORIENTED_EDGE('',*,*,#17767,.T.) ;
#26815=ORIENTED_EDGE('',*,*,#17770,.F.) ;
#26816=ORIENTED_EDGE('',*,*,#17773,.T.) ;
#26817=ORIENTED_EDGE('',*,*,#17776,.F.) ;
#26818=ORIENTED_EDGE('',*,*,#17779,.T.) ;
#26819=ORIENTED_EDGE('',*,*,#17781,.F.) ;
#26820=ORIENTED_EDGE('',*,*,#18030,.T.) ;
#26821=ORIENTED_EDGE('',*,*,#18032,.F.) ;
#26822=ORIENTED_EDGE('',*,*,#18035,.T.) ;
#26823=ORIENTED_EDGE('',*,*,#18038,.F.) ;
#26824=ORIENTED_EDGE('',*,*,#18041,.T.) ;
#26825=ORIENTED_EDGE('',*,*,#18044,.F.) ;
#26826=ORIENTED_EDGE('',*,*,#18047,.T.) ;
#26827=ORIENTED_EDGE('',*,*,#18048,.F.) ;
#26828=ORIENTED_EDGE('',*,*,#19001,.T.) ;
#26829=ORIENTED_EDGE('',*,*,#19002,.F.) ;
#26830=ORIENTED_EDGE('',*,*,#19003,.F.) ;
#26831=ORIENTED_EDGE('',*,*,#19004,.T.) ;
#26832=ORIENTED_EDGE('',*,*,#19001,.F.) ;
#26833=ORIENTED_EDGE('',*,*,#19004,.F.) ;
#26834=ORIENTED_EDGE('',*,*,#19005,.T.) ;
#26835=ORIENTED_EDGE('',*,*,#19006,.T.) ;
#26836=ORIENTED_EDGE('',*,*,#19002,.T.) ;
#26837=ORIENTED_EDGE('',*,*,#19003,.T.) ;
#26838=ORIENTED_EDGE('',*,*,#19006,.F.) ;
#26839=ORIENTED_EDGE('',*,*,#19005,.F.) ;
#26840=ORIENTED_EDGE('',*,*,#19007,.T.) ;
#26841=ORIENTED_EDGE('',*,*,#17440,.F.) ;
#26842=ORIENTED_EDGE('',*,*,#19007,.F.) ;
#26843=ORIENTED_EDGE('',*,*,#18042,.F.) ;
#26844=ORIENTED_EDGE('',*,*,#18052,.F.) ;
#26845=ORIENTED_EDGE('',*,*,#18697,.T.) ;
#26846=ORIENTED_EDGE('',*,*,#19008,.T.) ;
#26847=ORIENTED_EDGE('',*,*,#18045,.F.) ;
#26848=ORIENTED_EDGE('',*,*,#19008,.F.) ;
#26849=ORIENTED_EDGE('',*,*,#18721,.T.) ;
#26850=ORIENTED_EDGE('',*,*,#17502,.F.) ;
#26851=ORIENTED_EDGE('',*,*,#18967,.T.) ;
#26852=ORIENTED_EDGE('',*,*,#18925,.F.) ;
#26853=ORIENTED_EDGE('',*,*,#18970,.T.) ;
#26854=ORIENTED_EDGE('',*,*,#18990,.F.) ;
#26855=ORIENTED_EDGE('',*,*,#17795,.T.) ;
#26856=ORIENTED_EDGE('',*,*,#17797,.F.) ;
#26857=ORIENTED_EDGE('',*,*,#17800,.T.) ;
#26858=ORIENTED_EDGE('',*,*,#17803,.F.) ;
#26859=ORIENTED_EDGE('',*,*,#17806,.T.) ;
#26860=ORIENTED_EDGE('',*,*,#17809,.F.) ;
#26861=ORIENTED_EDGE('',*,*,#17812,.T.) ;
#26862=ORIENTED_EDGE('',*,*,#17814,.F.) ;
#26863=ORIENTED_EDGE('',*,*,#18067,.T.) ;
#26864=ORIENTED_EDGE('',*,*,#18069,.F.) ;
#26865=ORIENTED_EDGE('',*,*,#18072,.T.) ;
#26866=ORIENTED_EDGE('',*,*,#18075,.F.) ;
#26867=ORIENTED_EDGE('',*,*,#18078,.T.) ;
#26868=ORIENTED_EDGE('',*,*,#18081,.F.) ;
#26869=ORIENTED_EDGE('',*,*,#18084,.T.) ;
#26870=ORIENTED_EDGE('',*,*,#18085,.F.) ;
#26871=ORIENTED_EDGE('',*,*,#19009,.T.) ;
#26872=ORIENTED_EDGE('',*,*,#19010,.F.) ;
#26873=ORIENTED_EDGE('',*,*,#19011,.F.) ;
#26874=ORIENTED_EDGE('',*,*,#19012,.T.) ;
#26875=ORIENTED_EDGE('',*,*,#19009,.F.) ;
#26876=ORIENTED_EDGE('',*,*,#19012,.F.) ;
#26877=ORIENTED_EDGE('',*,*,#19013,.T.) ;
#26878=ORIENTED_EDGE('',*,*,#19014,.T.) ;
#26879=ORIENTED_EDGE('',*,*,#19010,.T.) ;
#26880=ORIENTED_EDGE('',*,*,#19011,.T.) ;
#26881=ORIENTED_EDGE('',*,*,#19014,.F.) ;
#26882=ORIENTED_EDGE('',*,*,#19013,.F.) ;
#26883=ORIENTED_EDGE('',*,*,#19015,.T.) ;
#26884=ORIENTED_EDGE('',*,*,#17441,.F.) ;
#26885=ORIENTED_EDGE('',*,*,#19015,.F.) ;
#26886=ORIENTED_EDGE('',*,*,#18079,.F.) ;
#26887=ORIENTED_EDGE('',*,*,#18089,.F.) ;
#26888=ORIENTED_EDGE('',*,*,#18650,.T.) ;
#26889=ORIENTED_EDGE('',*,*,#19016,.T.) ;
#26890=ORIENTED_EDGE('',*,*,#18082,.F.) ;
#26891=ORIENTED_EDGE('',*,*,#19016,.F.) ;
#26892=ORIENTED_EDGE('',*,*,#18674,.T.) ;
#26893=ORIENTED_EDGE('',*,*,#17533,.F.) ;
#26894=ORIENTED_EDGE('',*,*,#18961,.T.) ;
#26895=ORIENTED_EDGE('',*,*,#18921,.F.) ;
#26896=ORIENTED_EDGE('',*,*,#18964,.T.) ;
#26897=ORIENTED_EDGE('',*,*,#18989,.F.) ;
#26898=ORIENTED_EDGE('',*,*,#17828,.T.) ;
#26899=ORIENTED_EDGE('',*,*,#17830,.F.) ;
#26900=ORIENTED_EDGE('',*,*,#17833,.T.) ;
#26901=ORIENTED_EDGE('',*,*,#17836,.F.) ;
#26902=ORIENTED_EDGE('',*,*,#17839,.T.) ;
#26903=ORIENTED_EDGE('',*,*,#17842,.F.) ;
#26904=ORIENTED_EDGE('',*,*,#17845,.T.) ;
#26905=ORIENTED_EDGE('',*,*,#17847,.F.) ;
#26906=ORIENTED_EDGE('',*,*,#18104,.T.) ;
#26907=ORIENTED_EDGE('',*,*,#18106,.F.) ;
#26908=ORIENTED_EDGE('',*,*,#18109,.T.) ;
#26909=ORIENTED_EDGE('',*,*,#18112,.F.) ;
#26910=ORIENTED_EDGE('',*,*,#18115,.T.) ;
#26911=ORIENTED_EDGE('',*,*,#18118,.F.) ;
#26912=ORIENTED_EDGE('',*,*,#18121,.T.) ;
#26913=ORIENTED_EDGE('',*,*,#18122,.F.) ;
#26914=ORIENTED_EDGE('',*,*,#19017,.T.) ;
#26915=ORIENTED_EDGE('',*,*,#19018,.F.) ;
#26916=ORIENTED_EDGE('',*,*,#19019,.F.) ;
#26917=ORIENTED_EDGE('',*,*,#19020,.T.) ;
#26918=ORIENTED_EDGE('',*,*,#19017,.F.) ;
#26919=ORIENTED_EDGE('',*,*,#19020,.F.) ;
#26920=ORIENTED_EDGE('',*,*,#19021,.T.) ;
#26921=ORIENTED_EDGE('',*,*,#19022,.T.) ;
#26922=ORIENTED_EDGE('',*,*,#19018,.T.) ;
#26923=ORIENTED_EDGE('',*,*,#19019,.T.) ;
#26924=ORIENTED_EDGE('',*,*,#19022,.F.) ;
#26925=ORIENTED_EDGE('',*,*,#19021,.F.) ;
#26926=ORIENTED_EDGE('',*,*,#19023,.T.) ;
#26927=ORIENTED_EDGE('',*,*,#17442,.F.) ;
#26928=ORIENTED_EDGE('',*,*,#19023,.F.) ;
#26929=ORIENTED_EDGE('',*,*,#18116,.F.) ;
#26930=ORIENTED_EDGE('',*,*,#18126,.F.) ;
#26931=ORIENTED_EDGE('',*,*,#18603,.T.) ;
#26932=ORIENTED_EDGE('',*,*,#19024,.T.) ;
#26933=ORIENTED_EDGE('',*,*,#18119,.F.) ;
#26934=ORIENTED_EDGE('',*,*,#19024,.F.) ;
#26935=ORIENTED_EDGE('',*,*,#18627,.T.) ;
#26936=ORIENTED_EDGE('',*,*,#17564,.F.) ;
#26937=ORIENTED_EDGE('',*,*,#18955,.T.) ;
#26938=ORIENTED_EDGE('',*,*,#18917,.F.) ;
#26939=ORIENTED_EDGE('',*,*,#18958,.T.) ;
#26940=ORIENTED_EDGE('',*,*,#18988,.F.) ;
#26941=ORIENTED_EDGE('',*,*,#17861,.T.) ;
#26942=ORIENTED_EDGE('',*,*,#17863,.F.) ;
#26943=ORIENTED_EDGE('',*,*,#17866,.T.) ;
#26944=ORIENTED_EDGE('',*,*,#17869,.F.) ;
#26945=ORIENTED_EDGE('',*,*,#17872,.T.) ;
#26946=ORIENTED_EDGE('',*,*,#17875,.F.) ;
#26947=ORIENTED_EDGE('',*,*,#17878,.T.) ;
#26948=ORIENTED_EDGE('',*,*,#17880,.F.) ;
#26949=ORIENTED_EDGE('',*,*,#18141,.T.) ;
#26950=ORIENTED_EDGE('',*,*,#18143,.F.) ;
#26951=ORIENTED_EDGE('',*,*,#18146,.T.) ;
#26952=ORIENTED_EDGE('',*,*,#18149,.F.) ;
#26953=ORIENTED_EDGE('',*,*,#18152,.T.) ;
#26954=ORIENTED_EDGE('',*,*,#18155,.F.) ;
#26955=ORIENTED_EDGE('',*,*,#18158,.T.) ;
#26956=ORIENTED_EDGE('',*,*,#18159,.F.) ;
#26957=ORIENTED_EDGE('',*,*,#19025,.T.) ;
#26958=ORIENTED_EDGE('',*,*,#19026,.F.) ;
#26959=ORIENTED_EDGE('',*,*,#19027,.F.) ;
#26960=ORIENTED_EDGE('',*,*,#19028,.T.) ;
#26961=ORIENTED_EDGE('',*,*,#19025,.F.) ;
#26962=ORIENTED_EDGE('',*,*,#19028,.F.) ;
#26963=ORIENTED_EDGE('',*,*,#19029,.T.) ;
#26964=ORIENTED_EDGE('',*,*,#19030,.T.) ;
#26965=ORIENTED_EDGE('',*,*,#19026,.T.) ;
#26966=ORIENTED_EDGE('',*,*,#19027,.T.) ;
#26967=ORIENTED_EDGE('',*,*,#19030,.F.) ;
#26968=ORIENTED_EDGE('',*,*,#19029,.F.) ;
#26969=ORIENTED_EDGE('',*,*,#19031,.T.) ;
#26970=ORIENTED_EDGE('',*,*,#17443,.F.) ;
#26971=ORIENTED_EDGE('',*,*,#19031,.F.) ;
#26972=ORIENTED_EDGE('',*,*,#18153,.F.) ;
#26973=ORIENTED_EDGE('',*,*,#18163,.F.) ;
#26974=ORIENTED_EDGE('',*,*,#18556,.T.) ;
#26975=ORIENTED_EDGE('',*,*,#19032,.T.) ;
#26976=ORIENTED_EDGE('',*,*,#18156,.F.) ;
#26977=ORIENTED_EDGE('',*,*,#19032,.F.) ;
#26978=ORIENTED_EDGE('',*,*,#18580,.T.) ;
#26979=ORIENTED_EDGE('',*,*,#17595,.F.) ;
#26980=ORIENTED_EDGE('',*,*,#18949,.T.) ;
#26981=ORIENTED_EDGE('',*,*,#18913,.F.) ;
#26982=ORIENTED_EDGE('',*,*,#18952,.T.) ;
#26983=ORIENTED_EDGE('',*,*,#18987,.F.) ;
#26984=ORIENTED_EDGE('',*,*,#17894,.T.) ;
#26985=ORIENTED_EDGE('',*,*,#17896,.F.) ;
#26986=ORIENTED_EDGE('',*,*,#17899,.T.) ;
#26987=ORIENTED_EDGE('',*,*,#17902,.F.) ;
#26988=ORIENTED_EDGE('',*,*,#17905,.T.) ;
#26989=ORIENTED_EDGE('',*,*,#17908,.F.) ;
#26990=ORIENTED_EDGE('',*,*,#17911,.T.) ;
#26991=ORIENTED_EDGE('',*,*,#17913,.F.) ;
#26992=ORIENTED_EDGE('',*,*,#18178,.T.) ;
#26993=ORIENTED_EDGE('',*,*,#18180,.F.) ;
#26994=ORIENTED_EDGE('',*,*,#18183,.T.) ;
#26995=ORIENTED_EDGE('',*,*,#18186,.F.) ;
#26996=ORIENTED_EDGE('',*,*,#18189,.T.) ;
#26997=ORIENTED_EDGE('',*,*,#18192,.F.) ;
#26998=ORIENTED_EDGE('',*,*,#18195,.T.) ;
#26999=ORIENTED_EDGE('',*,*,#18196,.F.) ;
#27000=ORIENTED_EDGE('',*,*,#19033,.T.) ;
#27001=ORIENTED_EDGE('',*,*,#19034,.F.) ;
#27002=ORIENTED_EDGE('',*,*,#19035,.F.) ;
#27003=ORIENTED_EDGE('',*,*,#19036,.T.) ;
#27004=ORIENTED_EDGE('',*,*,#19033,.F.) ;
#27005=ORIENTED_EDGE('',*,*,#19036,.F.) ;
#27006=ORIENTED_EDGE('',*,*,#19037,.T.) ;
#27007=ORIENTED_EDGE('',*,*,#19038,.T.) ;
#27008=ORIENTED_EDGE('',*,*,#19034,.T.) ;
#27009=ORIENTED_EDGE('',*,*,#19035,.T.) ;
#27010=ORIENTED_EDGE('',*,*,#19038,.F.) ;
#27011=ORIENTED_EDGE('',*,*,#19037,.F.) ;
#27012=ORIENTED_EDGE('',*,*,#19039,.T.) ;
#27013=ORIENTED_EDGE('',*,*,#17444,.F.) ;
#27014=ORIENTED_EDGE('',*,*,#19039,.F.) ;
#27015=ORIENTED_EDGE('',*,*,#18190,.F.) ;
#27016=ORIENTED_EDGE('',*,*,#18200,.F.) ;
#27017=ORIENTED_EDGE('',*,*,#18509,.T.) ;
#27018=ORIENTED_EDGE('',*,*,#19040,.T.) ;
#27019=ORIENTED_EDGE('',*,*,#18193,.F.) ;
#27020=ORIENTED_EDGE('',*,*,#19040,.F.) ;
#27021=ORIENTED_EDGE('',*,*,#18533,.T.) ;
#27022=ORIENTED_EDGE('',*,*,#17626,.F.) ;
#27023=ORIENTED_EDGE('',*,*,#18943,.T.) ;
#27024=ORIENTED_EDGE('',*,*,#18909,.F.) ;
#27025=ORIENTED_EDGE('',*,*,#18946,.T.) ;
#27026=ORIENTED_EDGE('',*,*,#18986,.F.) ;
#27027=ORIENTED_EDGE('',*,*,#17927,.T.) ;
#27028=ORIENTED_EDGE('',*,*,#17929,.F.) ;
#27029=ORIENTED_EDGE('',*,*,#17932,.T.) ;
#27030=ORIENTED_EDGE('',*,*,#17935,.F.) ;
#27031=ORIENTED_EDGE('',*,*,#17938,.T.) ;
#27032=ORIENTED_EDGE('',*,*,#17941,.F.) ;
#27033=ORIENTED_EDGE('',*,*,#17944,.T.) ;
#27034=ORIENTED_EDGE('',*,*,#17946,.F.) ;
#27035=ORIENTED_EDGE('',*,*,#18215,.T.) ;
#27036=ORIENTED_EDGE('',*,*,#18217,.F.) ;
#27037=ORIENTED_EDGE('',*,*,#18220,.T.) ;
#27038=ORIENTED_EDGE('',*,*,#18223,.F.) ;
#27039=ORIENTED_EDGE('',*,*,#18226,.T.) ;
#27040=ORIENTED_EDGE('',*,*,#18229,.F.) ;
#27041=ORIENTED_EDGE('',*,*,#18232,.T.) ;
#27042=ORIENTED_EDGE('',*,*,#18233,.F.) ;
#27043=ORIENTED_EDGE('',*,*,#19041,.T.) ;
#27044=ORIENTED_EDGE('',*,*,#19042,.F.) ;
#27045=ORIENTED_EDGE('',*,*,#19043,.F.) ;
#27046=ORIENTED_EDGE('',*,*,#19044,.T.) ;
#27047=ORIENTED_EDGE('',*,*,#19041,.F.) ;
#27048=ORIENTED_EDGE('',*,*,#19044,.F.) ;
#27049=ORIENTED_EDGE('',*,*,#19045,.T.) ;
#27050=ORIENTED_EDGE('',*,*,#19046,.T.) ;
#27051=ORIENTED_EDGE('',*,*,#19042,.T.) ;
#27052=ORIENTED_EDGE('',*,*,#19043,.T.) ;
#27053=ORIENTED_EDGE('',*,*,#19046,.F.) ;
#27054=ORIENTED_EDGE('',*,*,#19045,.F.) ;
#27055=ORIENTED_EDGE('',*,*,#19047,.T.) ;
#27056=ORIENTED_EDGE('',*,*,#17445,.F.) ;
#27057=ORIENTED_EDGE('',*,*,#19047,.F.) ;
#27058=ORIENTED_EDGE('',*,*,#18227,.F.) ;
#27059=ORIENTED_EDGE('',*,*,#18237,.F.) ;
#27060=ORIENTED_EDGE('',*,*,#18462,.T.) ;
#27061=ORIENTED_EDGE('',*,*,#19048,.T.) ;
#27062=ORIENTED_EDGE('',*,*,#18230,.F.) ;
#27063=ORIENTED_EDGE('',*,*,#19048,.F.) ;
#27064=ORIENTED_EDGE('',*,*,#18486,.T.) ;
#27065=ORIENTED_EDGE('',*,*,#17657,.F.) ;
#27066=ORIENTED_EDGE('',*,*,#18937,.T.) ;
#27067=ORIENTED_EDGE('',*,*,#18905,.F.) ;
#27068=ORIENTED_EDGE('',*,*,#18940,.T.) ;
#27069=ORIENTED_EDGE('',*,*,#18985,.F.) ;
#27070=ORIENTED_EDGE('',*,*,#17960,.T.) ;
#27071=ORIENTED_EDGE('',*,*,#17962,.F.) ;
#27072=ORIENTED_EDGE('',*,*,#17965,.T.) ;
#27073=ORIENTED_EDGE('',*,*,#17968,.F.) ;
#27074=ORIENTED_EDGE('',*,*,#17971,.T.) ;
#27075=ORIENTED_EDGE('',*,*,#17974,.F.) ;
#27076=ORIENTED_EDGE('',*,*,#17977,.T.) ;
#27077=ORIENTED_EDGE('',*,*,#17979,.F.) ;
#27078=ORIENTED_EDGE('',*,*,#18252,.T.) ;
#27079=ORIENTED_EDGE('',*,*,#18254,.F.) ;
#27080=ORIENTED_EDGE('',*,*,#18257,.T.) ;
#27081=ORIENTED_EDGE('',*,*,#18260,.F.) ;
#27082=ORIENTED_EDGE('',*,*,#18263,.T.) ;
#27083=ORIENTED_EDGE('',*,*,#18266,.F.) ;
#27084=ORIENTED_EDGE('',*,*,#18269,.T.) ;
#27085=ORIENTED_EDGE('',*,*,#18270,.F.) ;
#27086=ORIENTED_EDGE('',*,*,#19049,.T.) ;
#27087=ORIENTED_EDGE('',*,*,#19050,.F.) ;
#27088=ORIENTED_EDGE('',*,*,#19051,.F.) ;
#27089=ORIENTED_EDGE('',*,*,#19052,.T.) ;
#27090=ORIENTED_EDGE('',*,*,#19049,.F.) ;
#27091=ORIENTED_EDGE('',*,*,#19052,.F.) ;
#27092=ORIENTED_EDGE('',*,*,#19053,.T.) ;
#27093=ORIENTED_EDGE('',*,*,#19054,.T.) ;
#27094=ORIENTED_EDGE('',*,*,#19050,.T.) ;
#27095=ORIENTED_EDGE('',*,*,#19051,.T.) ;
#27096=ORIENTED_EDGE('',*,*,#19054,.F.) ;
#27097=ORIENTED_EDGE('',*,*,#19053,.F.) ;
#27098=ORIENTED_EDGE('',*,*,#19055,.T.) ;
#27099=ORIENTED_EDGE('',*,*,#17446,.F.) ;
#27100=ORIENTED_EDGE('',*,*,#19055,.F.) ;
#27101=ORIENTED_EDGE('',*,*,#18264,.F.) ;
#27102=ORIENTED_EDGE('',*,*,#18274,.F.) ;
#27103=ORIENTED_EDGE('',*,*,#18415,.T.) ;
#27104=ORIENTED_EDGE('',*,*,#19056,.T.) ;
#27105=ORIENTED_EDGE('',*,*,#18267,.F.) ;
#27106=ORIENTED_EDGE('',*,*,#19056,.F.) ;
#27107=ORIENTED_EDGE('',*,*,#18439,.T.) ;
#27108=ORIENTED_EDGE('',*,*,#17688,.F.) ;
#27109=ORIENTED_EDGE('',*,*,#19057,.F.) ;
#27110=ORIENTED_EDGE('',*,*,#19058,.F.) ;
#27111=ORIENTED_EDGE('',*,*,#19059,.T.) ;
#27112=ORIENTED_EDGE('',*,*,#18331,.F.) ;
#27113=ORIENTED_EDGE('',*,*,#19059,.F.) ;
#27114=ORIENTED_EDGE('',*,*,#19060,.T.) ;
#27115=ORIENTED_EDGE('',*,*,#19061,.T.) ;
#27116=ORIENTED_EDGE('',*,*,#19057,.T.) ;
#27117=ORIENTED_EDGE('',*,*,#19058,.T.) ;
#27118=ORIENTED_EDGE('',*,*,#19061,.F.) ;
#27119=ORIENTED_EDGE('',*,*,#19060,.F.) ;
#27120=ORIENTED_EDGE('',*,*,#19062,.T.) ;
#27121=ORIENTED_EDGE('',*,*,#18372,.F.) ;
#27122=ORIENTED_EDGE('',*,*,#19062,.F.) ;
#27123=ORIENTED_EDGE('',*,*,#18984,.F.) ;
#27124=ORIENTED_EDGE('',*,*,#18859,.F.) ;
#27125=ORIENTED_EDGE('',*,*,#18893,.F.) ;
#27126=ORIENTED_EDGE('',*,*,#19063,.F.) ;
#27127=ORIENTED_EDGE('',*,*,#17244,.T.) ;
#27128=ORIENTED_EDGE('',*,*,#19063,.T.) ;
#27129=ORIENTED_EDGE('',*,*,#18892,.F.) ;
#27130=ORIENTED_EDGE('',*,*,#18983,.T.) ;
#27131=ORIENTED_EDGE('',*,*,#18931,.F.) ;
#27132=ORIENTED_EDGE('',*,*,#18978,.T.) ;
#27133=ORIENTED_EDGE('',*,*,#18890,.F.) ;
#27134=ORIENTED_EDGE('',*,*,#18977,.T.) ;
#27135=ORIENTED_EDGE('',*,*,#18927,.F.) ;
#27136=ORIENTED_EDGE('',*,*,#18972,.T.) ;
#27137=ORIENTED_EDGE('',*,*,#18886,.F.) ;
#27138=ORIENTED_EDGE('',*,*,#18971,.T.) ;
#27139=ORIENTED_EDGE('',*,*,#18923,.F.) ;
#27140=ORIENTED_EDGE('',*,*,#18966,.T.) ;
#27141=ORIENTED_EDGE('',*,*,#18883,.F.) ;
#27142=ORIENTED_EDGE('',*,*,#18965,.T.) ;
#27143=ORIENTED_EDGE('',*,*,#18919,.F.) ;
#27144=ORIENTED_EDGE('',*,*,#18960,.T.) ;
#27145=ORIENTED_EDGE('',*,*,#18880,.F.) ;
#27146=ORIENTED_EDGE('',*,*,#18959,.T.) ;
#27147=ORIENTED_EDGE('',*,*,#18915,.F.) ;
#27148=ORIENTED_EDGE('',*,*,#18954,.T.) ;
#27149=ORIENTED_EDGE('',*,*,#18878,.F.) ;
#27150=ORIENTED_EDGE('',*,*,#18953,.T.) ;
#27151=ORIENTED_EDGE('',*,*,#18911,.F.) ;
#27152=ORIENTED_EDGE('',*,*,#18948,.T.) ;
#27153=ORIENTED_EDGE('',*,*,#18875,.F.) ;
#27154=ORIENTED_EDGE('',*,*,#18947,.T.) ;
#27155=ORIENTED_EDGE('',*,*,#18907,.F.) ;
#27156=ORIENTED_EDGE('',*,*,#18942,.T.) ;
#27157=ORIENTED_EDGE('',*,*,#18871,.F.) ;
#27158=ORIENTED_EDGE('',*,*,#18941,.T.) ;
#27159=ORIENTED_EDGE('',*,*,#18903,.F.) ;
#27160=ORIENTED_EDGE('',*,*,#18936,.T.) ;
#27161=ORIENTED_EDGE('',*,*,#18866,.F.) ;
#27162=ORIENTED_EDGE('',*,*,#18870,.T.) ;
#27163=ORIENTED_EDGE('',*,*,#18901,.F.) ;
#27164=ORIENTED_EDGE('',*,*,#18896,.T.) ;
#27165=ORIENTED_EDGE('',*,*,#18899,.F.) ;
#27166=ORIENTED_EDGE('',*,*,#18934,.T.) ;
#27167=ORIENTED_EDGE('',*,*,#17281,.F.) ;
#27168=ORIENTED_EDGE('',*,*,#18820,.T.) ;
#27169=ORIENTED_EDGE('',*,*,#17427,.T.) ;
#27170=ORIENTED_EDGE('',*,*,#18819,.T.) ;
#27171=ORIENTED_EDGE('',*,*,#17277,.F.) ;
#27172=ORIENTED_EDGE('',*,*,#18812,.T.) ;
#27173=ORIENTED_EDGE('',*,*,#17412,.T.) ;
#27174=ORIENTED_EDGE('',*,*,#18811,.T.) ;
#27175=ORIENTED_EDGE('',*,*,#17273,.F.) ;
#27176=ORIENTED_EDGE('',*,*,#18810,.T.) ;
#27177=ORIENTED_EDGE('',*,*,#17395,.T.) ;
#27178=ORIENTED_EDGE('',*,*,#18809,.T.) ;
#27179=ORIENTED_EDGE('',*,*,#17269,.F.) ;
#27180=ORIENTED_EDGE('',*,*,#18818,.T.) ;
#27181=ORIENTED_EDGE('',*,*,#17378,.T.) ;
#27182=ORIENTED_EDGE('',*,*,#18817,.T.) ;
#27183=ORIENTED_EDGE('',*,*,#17265,.F.) ;
#27184=ORIENTED_EDGE('',*,*,#18822,.T.) ;
#27185=ORIENTED_EDGE('',*,*,#17361,.T.) ;
#27186=ORIENTED_EDGE('',*,*,#18821,.T.) ;
#27187=ORIENTED_EDGE('',*,*,#17261,.F.) ;
#27188=ORIENTED_EDGE('',*,*,#18813,.T.) ;
#27189=ORIENTED_EDGE('',*,*,#17342,.T.) ;
#27190=ORIENTED_EDGE('',*,*,#18814,.T.) ;
#27191=ORIENTED_EDGE('',*,*,#17257,.F.) ;
#27192=ORIENTED_EDGE('',*,*,#18807,.T.) ;
#27193=ORIENTED_EDGE('',*,*,#17325,.T.) ;
#27194=ORIENTED_EDGE('',*,*,#18808,.T.) ;
#27195=ORIENTED_EDGE('',*,*,#17253,.F.) ;
#27196=ORIENTED_EDGE('',*,*,#18815,.T.) ;
#27197=ORIENTED_EDGE('',*,*,#17308,.T.) ;
#27198=ORIENTED_EDGE('',*,*,#18816,.T.) ;
#27199=ORIENTED_EDGE('',*,*,#17249,.F.) ;
#27200=ORIENTED_EDGE('',*,*,#18823,.T.) ;
#27201=ORIENTED_EDGE('',*,*,#17291,.T.) ;
#27202=ORIENTED_EDGE('',*,*,#18824,.T.) ;
#27203=ORIENTED_EDGE('',*,*,#17245,.F.) ;
#27204=ORIENTED_EDGE('',*,*,#17749,.T.) ;
#27205=ORIENTED_EDGE('',*,*,#19064,.F.) ;
#27206=ORIENTED_EDGE('',*,*,#18782,.T.) ;
#27207=ORIENTED_EDGE('',*,*,#17757,.F.) ;
#27208=ORIENTED_EDGE('',*,*,#17747,.F.) ;
#27209=ORIENTED_EDGE('',*,*,#19065,.T.) ;
#27210=ORIENTED_EDGE('',*,*,#18783,.T.) ;
#27211=ORIENTED_EDGE('',*,*,#19064,.T.) ;
#27212=ORIENTED_EDGE('',*,*,#17744,.F.) ;
#27213=ORIENTED_EDGE('',*,*,#19066,.F.) ;
#27214=ORIENTED_EDGE('',*,*,#18779,.T.) ;
#27215=ORIENTED_EDGE('',*,*,#19065,.F.) ;
#27216=ORIENTED_EDGE('',*,*,#17741,.F.) ;
#27217=ORIENTED_EDGE('',*,*,#17752,.T.) ;
#27218=ORIENTED_EDGE('',*,*,#18785,.T.) ;
#27219=ORIENTED_EDGE('',*,*,#19066,.T.) ;
#27220=ORIENTED_EDGE('',*,*,#18012,.T.) ;
#27221=ORIENTED_EDGE('',*,*,#17469,.F.) ;
#27222=ORIENTED_EDGE('',*,*,#18772,.T.) ;
#27223=ORIENTED_EDGE('',*,*,#18025,.F.) ;
#27224=ORIENTED_EDGE('',*,*,#17782,.T.) ;
#27225=ORIENTED_EDGE('',*,*,#19067,.F.) ;
#27226=ORIENTED_EDGE('',*,*,#18735,.T.) ;
#27227=ORIENTED_EDGE('',*,*,#17790,.F.) ;
#27228=ORIENTED_EDGE('',*,*,#17780,.F.) ;
#27229=ORIENTED_EDGE('',*,*,#19068,.T.) ;
#27230=ORIENTED_EDGE('',*,*,#18736,.T.) ;
#27231=ORIENTED_EDGE('',*,*,#19067,.T.) ;
#27232=ORIENTED_EDGE('',*,*,#17777,.F.) ;
#27233=ORIENTED_EDGE('',*,*,#19069,.F.) ;
#27234=ORIENTED_EDGE('',*,*,#18732,.T.) ;
#27235=ORIENTED_EDGE('',*,*,#19068,.F.) ;
#27236=ORIENTED_EDGE('',*,*,#17774,.F.) ;
#27237=ORIENTED_EDGE('',*,*,#17785,.T.) ;
#27238=ORIENTED_EDGE('',*,*,#18738,.T.) ;
#27239=ORIENTED_EDGE('',*,*,#19069,.T.) ;
#27240=ORIENTED_EDGE('',*,*,#18049,.T.) ;
#27241=ORIENTED_EDGE('',*,*,#17500,.F.) ;
#27242=ORIENTED_EDGE('',*,*,#18725,.T.) ;
#27243=ORIENTED_EDGE('',*,*,#18062,.F.) ;
#27244=ORIENTED_EDGE('',*,*,#17815,.T.) ;
#27245=ORIENTED_EDGE('',*,*,#19070,.F.) ;
#27246=ORIENTED_EDGE('',*,*,#18688,.T.) ;
#27247=ORIENTED_EDGE('',*,*,#17823,.F.) ;
#27248=ORIENTED_EDGE('',*,*,#17813,.F.) ;
#27249=ORIENTED_EDGE('',*,*,#19071,.T.) ;
#27250=ORIENTED_EDGE('',*,*,#18689,.T.) ;
#27251=ORIENTED_EDGE('',*,*,#19070,.T.) ;
#27252=ORIENTED_EDGE('',*,*,#17810,.F.) ;
#27253=ORIENTED_EDGE('',*,*,#19072,.F.) ;
#27254=ORIENTED_EDGE('',*,*,#18685,.T.) ;
#27255=ORIENTED_EDGE('',*,*,#19071,.F.) ;
#27256=ORIENTED_EDGE('',*,*,#17807,.F.) ;
#27257=ORIENTED_EDGE('',*,*,#17818,.T.) ;
#27258=ORIENTED_EDGE('',*,*,#18691,.T.) ;
#27259=ORIENTED_EDGE('',*,*,#19072,.T.) ;
#27260=ORIENTED_EDGE('',*,*,#18086,.T.) ;
#27261=ORIENTED_EDGE('',*,*,#17531,.F.) ;
#27262=ORIENTED_EDGE('',*,*,#18678,.T.) ;
#27263=ORIENTED_EDGE('',*,*,#18099,.F.) ;
#27264=ORIENTED_EDGE('',*,*,#17848,.T.) ;
#27265=ORIENTED_EDGE('',*,*,#19073,.F.) ;
#27266=ORIENTED_EDGE('',*,*,#18641,.T.) ;
#27267=ORIENTED_EDGE('',*,*,#17856,.F.) ;
#27268=ORIENTED_EDGE('',*,*,#17846,.F.) ;
#27269=ORIENTED_EDGE('',*,*,#19074,.T.) ;
#27270=ORIENTED_EDGE('',*,*,#18642,.T.) ;
#27271=ORIENTED_EDGE('',*,*,#19073,.T.) ;
#27272=ORIENTED_EDGE('',*,*,#17843,.F.) ;
#27273=ORIENTED_EDGE('',*,*,#19075,.F.) ;
#27274=ORIENTED_EDGE('',*,*,#18638,.T.) ;
#27275=ORIENTED_EDGE('',*,*,#19074,.F.) ;
#27276=ORIENTED_EDGE('',*,*,#17840,.F.) ;
#27277=ORIENTED_EDGE('',*,*,#17851,.T.) ;
#27278=ORIENTED_EDGE('',*,*,#18644,.T.) ;
#27279=ORIENTED_EDGE('',*,*,#19075,.T.) ;
#27280=ORIENTED_EDGE('',*,*,#18123,.T.) ;
#27281=ORIENTED_EDGE('',*,*,#17562,.F.) ;
#27282=ORIENTED_EDGE('',*,*,#18631,.T.) ;
#27283=ORIENTED_EDGE('',*,*,#18136,.F.) ;
#27284=ORIENTED_EDGE('',*,*,#17881,.T.) ;
#27285=ORIENTED_EDGE('',*,*,#19076,.F.) ;
#27286=ORIENTED_EDGE('',*,*,#18594,.T.) ;
#27287=ORIENTED_EDGE('',*,*,#17889,.F.) ;
#27288=ORIENTED_EDGE('',*,*,#17879,.F.) ;
#27289=ORIENTED_EDGE('',*,*,#19077,.T.) ;
#27290=ORIENTED_EDGE('',*,*,#18595,.T.) ;
#27291=ORIENTED_EDGE('',*,*,#19076,.T.) ;
#27292=ORIENTED_EDGE('',*,*,#17876,.F.) ;
#27293=ORIENTED_EDGE('',*,*,#19078,.F.) ;
#27294=ORIENTED_EDGE('',*,*,#18591,.T.) ;
#27295=ORIENTED_EDGE('',*,*,#19077,.F.) ;
#27296=ORIENTED_EDGE('',*,*,#17873,.F.) ;
#27297=ORIENTED_EDGE('',*,*,#17884,.T.) ;
#27298=ORIENTED_EDGE('',*,*,#18597,.T.) ;
#27299=ORIENTED_EDGE('',*,*,#19078,.T.) ;
#27300=ORIENTED_EDGE('',*,*,#18160,.T.) ;
#27301=ORIENTED_EDGE('',*,*,#17593,.F.) ;
#27302=ORIENTED_EDGE('',*,*,#18584,.T.) ;
#27303=ORIENTED_EDGE('',*,*,#18173,.F.) ;
#27304=ORIENTED_EDGE('',*,*,#17914,.T.) ;
#27305=ORIENTED_EDGE('',*,*,#19079,.F.) ;
#27306=ORIENTED_EDGE('',*,*,#18547,.T.) ;
#27307=ORIENTED_EDGE('',*,*,#17922,.F.) ;
#27308=ORIENTED_EDGE('',*,*,#17912,.F.) ;
#27309=ORIENTED_EDGE('',*,*,#19080,.T.) ;
#27310=ORIENTED_EDGE('',*,*,#18548,.T.) ;
#27311=ORIENTED_EDGE('',*,*,#19079,.T.) ;
#27312=ORIENTED_EDGE('',*,*,#17909,.F.) ;
#27313=ORIENTED_EDGE('',*,*,#19081,.F.) ;
#27314=ORIENTED_EDGE('',*,*,#18544,.T.) ;
#27315=ORIENTED_EDGE('',*,*,#19080,.F.) ;
#27316=ORIENTED_EDGE('',*,*,#17906,.F.) ;
#27317=ORIENTED_EDGE('',*,*,#17917,.T.) ;
#27318=ORIENTED_EDGE('',*,*,#18550,.T.) ;
#27319=ORIENTED_EDGE('',*,*,#19081,.T.) ;
#27320=ORIENTED_EDGE('',*,*,#18197,.T.) ;
#27321=ORIENTED_EDGE('',*,*,#17624,.F.) ;
#27322=ORIENTED_EDGE('',*,*,#18537,.T.) ;
#27323=ORIENTED_EDGE('',*,*,#18210,.F.) ;
#27324=ORIENTED_EDGE('',*,*,#17947,.T.) ;
#27325=ORIENTED_EDGE('',*,*,#19082,.F.) ;
#27326=ORIENTED_EDGE('',*,*,#18500,.T.) ;
#27327=ORIENTED_EDGE('',*,*,#17955,.F.) ;
#27328=ORIENTED_EDGE('',*,*,#17945,.F.) ;
#27329=ORIENTED_EDGE('',*,*,#19083,.T.) ;
#27330=ORIENTED_EDGE('',*,*,#18501,.T.) ;
#27331=ORIENTED_EDGE('',*,*,#19082,.T.) ;
#27332=ORIENTED_EDGE('',*,*,#17942,.F.) ;
#27333=ORIENTED_EDGE('',*,*,#19084,.F.) ;
#27334=ORIENTED_EDGE('',*,*,#18497,.T.) ;
#27335=ORIENTED_EDGE('',*,*,#19083,.F.) ;
#27336=ORIENTED_EDGE('',*,*,#17939,.F.) ;
#27337=ORIENTED_EDGE('',*,*,#17950,.T.) ;
#27338=ORIENTED_EDGE('',*,*,#18503,.T.) ;
#27339=ORIENTED_EDGE('',*,*,#19084,.T.) ;
#27340=ORIENTED_EDGE('',*,*,#18234,.T.) ;
#27341=ORIENTED_EDGE('',*,*,#17655,.F.) ;
#27342=ORIENTED_EDGE('',*,*,#18490,.T.) ;
#27343=ORIENTED_EDGE('',*,*,#18247,.F.) ;
#27344=ORIENTED_EDGE('',*,*,#17980,.T.) ;
#27345=ORIENTED_EDGE('',*,*,#19085,.F.) ;
#27346=ORIENTED_EDGE('',*,*,#18453,.T.) ;
#27347=ORIENTED_EDGE('',*,*,#17988,.F.) ;
#27348=ORIENTED_EDGE('',*,*,#17978,.F.) ;
#27349=ORIENTED_EDGE('',*,*,#19086,.T.) ;
#27350=ORIENTED_EDGE('',*,*,#18454,.T.) ;
#27351=ORIENTED_EDGE('',*,*,#19085,.T.) ;
#27352=ORIENTED_EDGE('',*,*,#17975,.F.) ;
#27353=ORIENTED_EDGE('',*,*,#19087,.F.) ;
#27354=ORIENTED_EDGE('',*,*,#18450,.T.) ;
#27355=ORIENTED_EDGE('',*,*,#19086,.F.) ;
#27356=ORIENTED_EDGE('',*,*,#17972,.F.) ;
#27357=ORIENTED_EDGE('',*,*,#17983,.T.) ;
#27358=ORIENTED_EDGE('',*,*,#18456,.T.) ;
#27359=ORIENTED_EDGE('',*,*,#19087,.T.) ;
#27360=ORIENTED_EDGE('',*,*,#18271,.T.) ;
#27361=ORIENTED_EDGE('',*,*,#17686,.F.) ;
#27362=ORIENTED_EDGE('',*,*,#18443,.T.) ;
#27363=ORIENTED_EDGE('',*,*,#18284,.F.) ;
#30195=CYLINDRICAL_SURFACE('',#33760,1.5) ;
#30196=CYLINDRICAL_SURFACE('',#33771,1.5) ;
#30197=CYLINDRICAL_SURFACE('',#33782,1.5) ;
#30198=CYLINDRICAL_SURFACE('',#33793,1.5) ;
#30199=CYLINDRICAL_SURFACE('',#33804,1.5) ;
#30200=CYLINDRICAL_SURFACE('',#33815,1.5) ;
#30201=CYLINDRICAL_SURFACE('',#33826,1.5) ;
#30202=CYLINDRICAL_SURFACE('',#33837,1.5) ;
#30203=CYLINDRICAL_SURFACE('',#33853,1.5) ;
#30204=CYLINDRICAL_SURFACE('',#33871,0.25) ;
#30205=CYLINDRICAL_SURFACE('',#33877,0.25) ;
#30206=CYLINDRICAL_SURFACE('',#33882,0.25) ;
#30207=CYLINDRICAL_SURFACE('',#33887,0.25) ;
#30208=CYLINDRICAL_SURFACE('',#33891,0.125) ;
#30209=CYLINDRICAL_SURFACE('',#33896,0.125) ;
#30210=CYLINDRICAL_SURFACE('',#33899,0.25) ;
#30211=CYLINDRICAL_SURFACE('',#33905,0.25) ;
#30212=CYLINDRICAL_SURFACE('',#33910,0.25) ;
#30213=CYLINDRICAL_SURFACE('',#33915,0.25) ;
#30214=CYLINDRICAL_SURFACE('',#33919,0.125) ;
#30215=CYLINDRICAL_SURFACE('',#33924,0.125) ;
#30216=CYLINDRICAL_SURFACE('',#33927,0.25) ;
#30217=CYLINDRICAL_SURFACE('',#33933,0.25) ;
#30218=CYLINDRICAL_SURFACE('',#33938,0.25) ;
#30219=CYLINDRICAL_SURFACE('',#33943,0.25) ;
#30220=CYLINDRICAL_SURFACE('',#33947,0.125) ;
#30221=CYLINDRICAL_SURFACE('',#33952,0.125) ;
#30222=CYLINDRICAL_SURFACE('',#33955,0.25) ;
#30223=CYLINDRICAL_SURFACE('',#33961,0.25) ;
#30224=CYLINDRICAL_SURFACE('',#33966,0.25) ;
#30225=CYLINDRICAL_SURFACE('',#33971,0.25) ;
#30226=CYLINDRICAL_SURFACE('',#33975,0.125) ;
#30227=CYLINDRICAL_SURFACE('',#33980,0.125) ;
#30228=CYLINDRICAL_SURFACE('',#33983,0.25) ;
#30229=CYLINDRICAL_SURFACE('',#33989,0.25) ;
#30230=CYLINDRICAL_SURFACE('',#33994,0.25) ;
#30231=CYLINDRICAL_SURFACE('',#33999,0.25) ;
#30232=CYLINDRICAL_SURFACE('',#34003,0.125) ;
#30233=CYLINDRICAL_SURFACE('',#34008,0.125) ;
#30234=CYLINDRICAL_SURFACE('',#34011,0.25) ;
#30235=CYLINDRICAL_SURFACE('',#34017,0.25) ;
#30236=CYLINDRICAL_SURFACE('',#34022,0.25) ;
#30237=CYLINDRICAL_SURFACE('',#34027,0.25) ;
#30238=CYLINDRICAL_SURFACE('',#34031,0.125) ;
#30239=CYLINDRICAL_SURFACE('',#34036,0.125) ;
#30240=CYLINDRICAL_SURFACE('',#34039,0.25) ;
#30241=CYLINDRICAL_SURFACE('',#34045,0.25) ;
#30242=CYLINDRICAL_SURFACE('',#34050,0.25) ;
#30243=CYLINDRICAL_SURFACE('',#34055,0.25) ;
#30244=CYLINDRICAL_SURFACE('',#34059,0.125) ;
#30245=CYLINDRICAL_SURFACE('',#34064,0.125) ;
#30246=CYLINDRICAL_SURFACE('',#34067,0.25) ;
#30247=CYLINDRICAL_SURFACE('',#34073,0.25) ;
#30248=CYLINDRICAL_SURFACE('',#34078,0.25) ;
#30249=CYLINDRICAL_SURFACE('',#34083,0.25) ;
#30250=CYLINDRICAL_SURFACE('',#34087,0.125) ;
#30251=CYLINDRICAL_SURFACE('',#34092,0.125) ;
#30252=CYLINDRICAL_SURFACE('',#34095,0.25) ;
#30253=CYLINDRICAL_SURFACE('',#34101,0.25) ;
#30254=CYLINDRICAL_SURFACE('',#34106,0.25) ;
#30255=CYLINDRICAL_SURFACE('',#34111,0.25) ;
#30256=CYLINDRICAL_SURFACE('',#34115,0.125) ;
#30257=CYLINDRICAL_SURFACE('',#34120,0.125) ;
#30258=CYLINDRICAL_SURFACE('',#34123,0.25) ;
#30259=CYLINDRICAL_SURFACE('',#34130,0.25) ;
#30260=CYLINDRICAL_SURFACE('',#34136,0.25) ;
#30261=CYLINDRICAL_SURFACE('',#34142,0.25) ;
#30262=CYLINDRICAL_SURFACE('',#34147,0.125) ;
#30263=CYLINDRICAL_SURFACE('',#34150,0.125) ;
#30264=CYLINDRICAL_SURFACE('',#34153,0.25) ;
#30265=CYLINDRICAL_SURFACE('',#34160,0.25) ;
#30266=CYLINDRICAL_SURFACE('',#34166,0.25) ;
#30267=CYLINDRICAL_SURFACE('',#34172,0.25) ;
#30268=CYLINDRICAL_SURFACE('',#34177,0.125) ;
#30269=CYLINDRICAL_SURFACE('',#34180,0.125) ;
#30270=CYLINDRICAL_SURFACE('',#34183,0.25) ;
#30271=CYLINDRICAL_SURFACE('',#34190,0.25) ;
#30272=CYLINDRICAL_SURFACE('',#34196,0.25) ;
#30273=CYLINDRICAL_SURFACE('',#34202,0.25) ;
#30274=CYLINDRICAL_SURFACE('',#34207,0.125) ;
#30275=CYLINDRICAL_SURFACE('',#34210,0.125) ;
#30276=CYLINDRICAL_SURFACE('',#34213,0.25) ;
#30277=CYLINDRICAL_SURFACE('',#34220,0.25) ;
#30278=CYLINDRICAL_SURFACE('',#34226,0.25) ;
#30279=CYLINDRICAL_SURFACE('',#34232,0.25) ;
#30280=CYLINDRICAL_SURFACE('',#34237,0.125) ;
#30281=CYLINDRICAL_SURFACE('',#34240,0.125) ;
#30282=CYLINDRICAL_SURFACE('',#34243,0.25) ;
#30283=CYLINDRICAL_SURFACE('',#34250,0.25) ;
#30284=CYLINDRICAL_SURFACE('',#34256,0.25) ;
#30285=CYLINDRICAL_SURFACE('',#34262,0.25) ;
#30286=CYLINDRICAL_SURFACE('',#34267,0.125) ;
#30287=CYLINDRICAL_SURFACE('',#34270,0.125) ;
#30288=CYLINDRICAL_SURFACE('',#34273,0.25) ;
#30289=CYLINDRICAL_SURFACE('',#34280,0.25) ;
#30290=CYLINDRICAL_SURFACE('',#34286,0.25) ;
#30291=CYLINDRICAL_SURFACE('',#34292,0.25) ;
#30292=CYLINDRICAL_SURFACE('',#34297,0.125) ;
#30293=CYLINDRICAL_SURFACE('',#34300,0.125) ;
#30294=CYLINDRICAL_SURFACE('',#34303,0.25) ;
#30295=CYLINDRICAL_SURFACE('',#34310,0.25) ;
#30296=CYLINDRICAL_SURFACE('',#34316,0.25) ;
#30297=CYLINDRICAL_SURFACE('',#34322,0.25) ;
#30298=CYLINDRICAL_SURFACE('',#34327,0.125) ;
#30299=CYLINDRICAL_SURFACE('',#34330,0.125) ;
#30300=CYLINDRICAL_SURFACE('',#34333,0.25) ;
#30301=CYLINDRICAL_SURFACE('',#34340,0.25) ;
#30302=CYLINDRICAL_SURFACE('',#34346,0.25) ;
#30303=CYLINDRICAL_SURFACE('',#34352,0.25) ;
#30304=CYLINDRICAL_SURFACE('',#34357,0.125) ;
#30305=CYLINDRICAL_SURFACE('',#34360,0.125) ;
#30306=CYLINDRICAL_SURFACE('',#34363,0.25) ;
#30307=CYLINDRICAL_SURFACE('',#34370,0.25) ;
#30308=CYLINDRICAL_SURFACE('',#34376,0.25) ;
#30309=CYLINDRICAL_SURFACE('',#34382,0.25) ;
#30310=CYLINDRICAL_SURFACE('',#34387,0.125) ;
#30311=CYLINDRICAL_SURFACE('',#34392,0.125) ;
#30312=CYLINDRICAL_SURFACE('',#34395,0.25) ;
#30313=CYLINDRICAL_SURFACE('',#34402,0.25) ;
#30314=CYLINDRICAL_SURFACE('',#34408,0.25) ;
#30315=CYLINDRICAL_SURFACE('',#34414,0.25) ;
#30316=CYLINDRICAL_SURFACE('',#34419,0.125) ;
#30317=CYLINDRICAL_SURFACE('',#34424,0.125) ;
#30318=CYLINDRICAL_SURFACE('',#34427,0.25) ;
#30319=CYLINDRICAL_SURFACE('',#34434,0.25) ;
#30320=CYLINDRICAL_SURFACE('',#34440,0.25) ;
#30321=CYLINDRICAL_SURFACE('',#34446,0.25) ;
#30322=CYLINDRICAL_SURFACE('',#34451,0.125) ;
#30323=CYLINDRICAL_SURFACE('',#34456,0.125) ;
#30324=CYLINDRICAL_SURFACE('',#34459,0.25) ;
#30325=CYLINDRICAL_SURFACE('',#34466,0.25) ;
#30326=CYLINDRICAL_SURFACE('',#34472,0.25) ;
#30327=CYLINDRICAL_SURFACE('',#34478,0.25) ;
#30328=CYLINDRICAL_SURFACE('',#34483,0.125) ;
#30329=CYLINDRICAL_SURFACE('',#34488,0.125) ;
#30330=CYLINDRICAL_SURFACE('',#34491,0.25) ;
#30331=CYLINDRICAL_SURFACE('',#34498,0.25) ;
#30332=CYLINDRICAL_SURFACE('',#34504,0.25) ;
#30333=CYLINDRICAL_SURFACE('',#34510,0.25) ;
#30334=CYLINDRICAL_SURFACE('',#34515,0.125) ;
#30335=CYLINDRICAL_SURFACE('',#34520,0.125) ;
#30336=CYLINDRICAL_SURFACE('',#34523,0.25) ;
#30337=CYLINDRICAL_SURFACE('',#34530,0.25) ;
#30338=CYLINDRICAL_SURFACE('',#34536,0.25) ;
#30339=CYLINDRICAL_SURFACE('',#34542,0.25) ;
#30340=CYLINDRICAL_SURFACE('',#34547,0.125) ;
#30341=CYLINDRICAL_SURFACE('',#34552,0.125) ;
#30342=CYLINDRICAL_SURFACE('',#34555,0.25) ;
#30343=CYLINDRICAL_SURFACE('',#34562,0.25) ;
#30344=CYLINDRICAL_SURFACE('',#34568,0.25) ;
#30345=CYLINDRICAL_SURFACE('',#34574,0.25) ;
#30346=CYLINDRICAL_SURFACE('',#34579,0.125) ;
#30347=CYLINDRICAL_SURFACE('',#34584,0.125) ;
#30348=CYLINDRICAL_SURFACE('',#34587,0.25) ;
#30349=CYLINDRICAL_SURFACE('',#34594,0.25) ;
#30350=CYLINDRICAL_SURFACE('',#34600,0.25) ;
#30351=CYLINDRICAL_SURFACE('',#34606,0.25) ;
#30352=CYLINDRICAL_SURFACE('',#34611,0.125) ;
#30353=CYLINDRICAL_SURFACE('',#34616,0.125) ;
#30354=CYLINDRICAL_SURFACE('',#34619,0.25) ;
#30355=CYLINDRICAL_SURFACE('',#34626,0.25) ;
#30356=CYLINDRICAL_SURFACE('',#34632,0.25) ;
#30357=CYLINDRICAL_SURFACE('',#34638,0.25) ;
#30358=CYLINDRICAL_SURFACE('',#34643,0.125) ;
#30359=CYLINDRICAL_SURFACE('',#34646,0.125) ;
#30360=CYLINDRICAL_SURFACE('',#34655,0.25) ;
#30361=CYLINDRICAL_SURFACE('',#34661,0.25) ;
#30362=CYLINDRICAL_SURFACE('',#34666,0.25) ;
#30363=CYLINDRICAL_SURFACE('',#34671,0.25) ;
#30364=CYLINDRICAL_SURFACE('',#34675,0.125) ;
#30365=CYLINDRICAL_SURFACE('',#34680,0.125) ;
#30366=CYLINDRICAL_SURFACE('',#34684,0.125) ;
#30367=CYLINDRICAL_SURFACE('',#34686,0.125) ;
#30368=CYLINDRICAL_SURFACE('',#34689,0.125) ;
#30369=CYLINDRICAL_SURFACE('',#34691,0.125) ;
#30370=CYLINDRICAL_SURFACE('',#34696,0.125) ;
#30371=CYLINDRICAL_SURFACE('',#34698,0.125) ;
#30372=CYLINDRICAL_SURFACE('',#34704,0.125) ;
#30373=CYLINDRICAL_SURFACE('',#34713,0.125) ;
#30374=CYLINDRICAL_SURFACE('',#34714,0.125) ;
#30375=CYLINDRICAL_SURFACE('',#34719,0.125) ;
#30376=CYLINDRICAL_SURFACE('',#34721,0.0635000000000012) ;
#30377=CYLINDRICAL_SURFACE('',#34722,0.125) ;
#30378=CYLINDRICAL_SURFACE('',#34724,0.0634999999999974) ;
#30379=CYLINDRICAL_SURFACE('',#34727,0.125) ;
#30380=CYLINDRICAL_SURFACE('',#34742,0.125) ;
#30381=CYLINDRICAL_SURFACE('',#34743,0.125) ;
#30382=CYLINDRICAL_SURFACE('',#34745,0.125) ;
#30383=CYLINDRICAL_SURFACE('',#34747,0.125) ;
#30384=CYLINDRICAL_SURFACE('',#34752,0.125) ;
#30385=CYLINDRICAL_SURFACE('',#34754,0.125) ;
#30386=CYLINDRICAL_SURFACE('',#34760,0.125) ;
#30387=CYLINDRICAL_SURFACE('',#34769,0.125) ;
#30388=CYLINDRICAL_SURFACE('',#34770,0.125) ;
#30389=CYLINDRICAL_SURFACE('',#34775,0.125) ;
#30390=CYLINDRICAL_SURFACE('',#34777,0.0635000000000012) ;
#30391=CYLINDRICAL_SURFACE('',#34778,0.125) ;
#30392=CYLINDRICAL_SURFACE('',#34780,0.0634999999999974) ;
#30393=CYLINDRICAL_SURFACE('',#34784,0.125) ;
#30394=CYLINDRICAL_SURFACE('',#34802,0.125) ;
#30395=CYLINDRICAL_SURFACE('',#34803,0.125) ;
#30396=CYLINDRICAL_SURFACE('',#34805,0.125) ;
#30397=CYLINDRICAL_SURFACE('',#34807,0.125) ;
#30398=CYLINDRICAL_SURFACE('',#34812,0.125) ;
#30399=CYLINDRICAL_SURFACE('',#34814,0.125) ;
#30400=CYLINDRICAL_SURFACE('',#34820,0.125) ;
#30401=CYLINDRICAL_SURFACE('',#34829,0.125) ;
#30402=CYLINDRICAL_SURFACE('',#34830,0.125) ;
#30403=CYLINDRICAL_SURFACE('',#34835,0.125) ;
#30404=CYLINDRICAL_SURFACE('',#34837,0.0635000000000012) ;
#30405=CYLINDRICAL_SURFACE('',#34838,0.125) ;
#30406=CYLINDRICAL_SURFACE('',#34840,0.0634999999999974) ;
#30407=CYLINDRICAL_SURFACE('',#34844,0.125) ;
#30408=CYLINDRICAL_SURFACE('',#34862,0.125) ;
#30409=CYLINDRICAL_SURFACE('',#34863,0.125) ;
#30410=CYLINDRICAL_SURFACE('',#34865,0.125) ;
#30411=CYLINDRICAL_SURFACE('',#34867,0.125) ;
#30412=CYLINDRICAL_SURFACE('',#34872,0.125) ;
#30413=CYLINDRICAL_SURFACE('',#34874,0.125) ;
#30414=CYLINDRICAL_SURFACE('',#34880,0.125) ;
#30415=CYLINDRICAL_SURFACE('',#34889,0.125) ;
#30416=CYLINDRICAL_SURFACE('',#34890,0.125) ;
#30417=CYLINDRICAL_SURFACE('',#34895,0.125) ;
#30418=CYLINDRICAL_SURFACE('',#34897,0.0635000000000012) ;
#30419=CYLINDRICAL_SURFACE('',#34898,0.125) ;
#30420=CYLINDRICAL_SURFACE('',#34900,0.0634999999999974) ;
#30421=CYLINDRICAL_SURFACE('',#34904,0.125) ;
#30422=CYLINDRICAL_SURFACE('',#34922,0.125) ;
#30423=CYLINDRICAL_SURFACE('',#34923,0.125) ;
#30424=CYLINDRICAL_SURFACE('',#34925,0.125) ;
#30425=CYLINDRICAL_SURFACE('',#34927,0.125) ;
#30426=CYLINDRICAL_SURFACE('',#34932,0.125) ;
#30427=CYLINDRICAL_SURFACE('',#34934,0.125) ;
#30428=CYLINDRICAL_SURFACE('',#34940,0.125) ;
#30429=CYLINDRICAL_SURFACE('',#34949,0.125) ;
#30430=CYLINDRICAL_SURFACE('',#34950,0.125) ;
#30431=CYLINDRICAL_SURFACE('',#34955,0.125) ;
#30432=CYLINDRICAL_SURFACE('',#34957,0.0635000000000012) ;
#30433=CYLINDRICAL_SURFACE('',#34958,0.125) ;
#30434=CYLINDRICAL_SURFACE('',#34960,0.0634999999999974) ;
#30435=CYLINDRICAL_SURFACE('',#34964,0.125) ;
#30436=CYLINDRICAL_SURFACE('',#34982,0.125) ;
#30437=CYLINDRICAL_SURFACE('',#34983,0.125) ;
#30438=CYLINDRICAL_SURFACE('',#34985,0.125) ;
#30439=CYLINDRICAL_SURFACE('',#34987,0.125) ;
#30440=CYLINDRICAL_SURFACE('',#34992,0.125) ;
#30441=CYLINDRICAL_SURFACE('',#34994,0.125) ;
#30442=CYLINDRICAL_SURFACE('',#35000,0.125) ;
#30443=CYLINDRICAL_SURFACE('',#35009,0.125) ;
#30444=CYLINDRICAL_SURFACE('',#35010,0.125) ;
#30445=CYLINDRICAL_SURFACE('',#35015,0.125) ;
#30446=CYLINDRICAL_SURFACE('',#35017,0.0635000000000012) ;
#30447=CYLINDRICAL_SURFACE('',#35018,0.125) ;
#30448=CYLINDRICAL_SURFACE('',#35020,0.0634999999999974) ;
#30449=CYLINDRICAL_SURFACE('',#35024,0.125) ;
#30450=CYLINDRICAL_SURFACE('',#35042,0.125) ;
#30451=CYLINDRICAL_SURFACE('',#35043,0.125) ;
#30452=CYLINDRICAL_SURFACE('',#35045,0.125) ;
#30453=CYLINDRICAL_SURFACE('',#35047,0.125) ;
#30454=CYLINDRICAL_SURFACE('',#35052,0.125) ;
#30455=CYLINDRICAL_SURFACE('',#35054,0.125) ;
#30456=CYLINDRICAL_SURFACE('',#35060,0.125) ;
#30457=CYLINDRICAL_SURFACE('',#35069,0.125) ;
#30458=CYLINDRICAL_SURFACE('',#35070,0.125) ;
#30459=CYLINDRICAL_SURFACE('',#35075,0.125) ;
#30460=CYLINDRICAL_SURFACE('',#35077,0.0635000000000012) ;
#30461=CYLINDRICAL_SURFACE('',#35078,0.125) ;
#30462=CYLINDRICAL_SURFACE('',#35080,0.0634999999999974) ;
#30463=CYLINDRICAL_SURFACE('',#35084,0.125) ;
#30464=CYLINDRICAL_SURFACE('',#35102,0.125) ;
#30465=CYLINDRICAL_SURFACE('',#35103,0.125) ;
#30466=CYLINDRICAL_SURFACE('',#35105,0.125) ;
#30467=CYLINDRICAL_SURFACE('',#35107,0.125) ;
#30468=CYLINDRICAL_SURFACE('',#35112,0.125) ;
#30469=CYLINDRICAL_SURFACE('',#35114,0.125) ;
#30470=CYLINDRICAL_SURFACE('',#35120,0.125) ;
#30471=CYLINDRICAL_SURFACE('',#35129,0.125) ;
#30472=CYLINDRICAL_SURFACE('',#35130,0.125) ;
#30473=CYLINDRICAL_SURFACE('',#35135,0.125) ;
#30474=CYLINDRICAL_SURFACE('',#35137,0.0635000000000012) ;
#30475=CYLINDRICAL_SURFACE('',#35138,0.125) ;
#30476=CYLINDRICAL_SURFACE('',#35140,0.0634999999999974) ;
#30477=CYLINDRICAL_SURFACE('',#35144,0.125) ;
#30478=CYLINDRICAL_SURFACE('',#35162,0.125) ;
#30479=CYLINDRICAL_SURFACE('',#35163,0.125) ;
#30480=CYLINDRICAL_SURFACE('',#35165,0.125) ;
#30481=CYLINDRICAL_SURFACE('',#35167,0.125) ;
#30482=CYLINDRICAL_SURFACE('',#35172,0.125) ;
#30483=CYLINDRICAL_SURFACE('',#35174,0.125) ;
#30484=CYLINDRICAL_SURFACE('',#35180,0.125) ;
#30485=CYLINDRICAL_SURFACE('',#35189,0.125) ;
#30486=CYLINDRICAL_SURFACE('',#35190,0.125) ;
#30487=CYLINDRICAL_SURFACE('',#35195,0.125) ;
#30488=CYLINDRICAL_SURFACE('',#35197,0.0635000000000012) ;
#30489=CYLINDRICAL_SURFACE('',#35198,0.125) ;
#30490=CYLINDRICAL_SURFACE('',#35200,0.0634999999999974) ;
#30491=CYLINDRICAL_SURFACE('',#35204,0.125) ;
#30492=CYLINDRICAL_SURFACE('',#35222,0.125) ;
#30493=CYLINDRICAL_SURFACE('',#35223,0.125) ;
#30494=CYLINDRICAL_SURFACE('',#35225,0.125) ;
#30495=CYLINDRICAL_SURFACE('',#35227,0.125) ;
#30496=CYLINDRICAL_SURFACE('',#35260,0.75) ;
#30497=CYLINDRICAL_SURFACE('',#35264,0.75) ;
#30498=CYLINDRICAL_SURFACE('',#35267,0.75) ;
#30499=CYLINDRICAL_SURFACE('',#35270,0.75) ;
#30500=CYLINDRICAL_SURFACE('',#35273,0.75) ;
#30501=CYLINDRICAL_SURFACE('',#35276,0.75) ;
#30502=CYLINDRICAL_SURFACE('',#35279,0.75) ;
#30503=CYLINDRICAL_SURFACE('',#35282,0.75) ;
#30504=CYLINDRICAL_SURFACE('',#35285,0.75) ;
#30505=CYLINDRICAL_SURFACE('',#35290,0.75) ;
#30506=CYLINDRICAL_SURFACE('',#35334,2.8575) ;
#30507=CYLINDRICAL_SURFACE('',#35339,0.125) ;
#30508=CYLINDRICAL_SURFACE('',#35346,2.8575) ;
#30509=CYLINDRICAL_SURFACE('',#35351,0.125) ;
#30510=CYLINDRICAL_SURFACE('',#35358,2.8575) ;
#30511=CYLINDRICAL_SURFACE('',#35363,0.125) ;
#30512=CYLINDRICAL_SURFACE('',#35370,2.8575) ;
#30513=CYLINDRICAL_SURFACE('',#35375,0.125) ;
#30514=CYLINDRICAL_SURFACE('',#35382,2.8575) ;
#30515=CYLINDRICAL_SURFACE('',#35387,0.125) ;
#30516=CYLINDRICAL_SURFACE('',#35394,2.8575) ;
#30517=CYLINDRICAL_SURFACE('',#35399,0.125) ;
#30518=CYLINDRICAL_SURFACE('',#35406,2.8575) ;
#30519=CYLINDRICAL_SURFACE('',#35411,0.125) ;
#30520=CYLINDRICAL_SURFACE('',#35418,2.8575) ;
#30521=CYLINDRICAL_SURFACE('',#35423,0.125) ;
#30522=CYLINDRICAL_SURFACE('',#35428,2.8575) ;
#30523=CYLINDRICAL_SURFACE('',#35434,0.125) ;
#30524=CYLINDRICAL_SURFACE('',#35436,0.125) ;
#30525=CYLINDRICAL_SURFACE('',#35438,0.125) ;
#30526=CYLINDRICAL_SURFACE('',#35439,0.125) ;
#30527=CYLINDRICAL_SURFACE('',#35441,0.125) ;
#30528=CYLINDRICAL_SURFACE('',#35443,0.125) ;
#30529=CYLINDRICAL_SURFACE('',#35444,0.125) ;
#30530=CYLINDRICAL_SURFACE('',#35446,0.125) ;
#30531=CYLINDRICAL_SURFACE('',#35448,0.125) ;
#30532=CYLINDRICAL_SURFACE('',#35449,0.125) ;
#30533=CYLINDRICAL_SURFACE('',#35451,0.125) ;
#30534=CYLINDRICAL_SURFACE('',#35453,0.125) ;
#30535=CYLINDRICAL_SURFACE('',#35454,0.125) ;
#30536=CYLINDRICAL_SURFACE('',#35456,0.125) ;
#30537=CYLINDRICAL_SURFACE('',#35458,0.125) ;
#30538=CYLINDRICAL_SURFACE('',#35459,0.125) ;
#30539=CYLINDRICAL_SURFACE('',#35461,0.125) ;
#30540=CYLINDRICAL_SURFACE('',#35463,0.125) ;
#30541=CYLINDRICAL_SURFACE('',#35464,0.125) ;
#30542=CYLINDRICAL_SURFACE('',#35466,0.125) ;
#30543=CYLINDRICAL_SURFACE('',#35468,0.125) ;
#30544=CYLINDRICAL_SURFACE('',#35469,0.125) ;
#30545=CYLINDRICAL_SURFACE('',#35471,0.125) ;
#30546=CYLINDRICAL_SURFACE('',#35473,0.125) ;
#31259=ADVANCED_FACE('',(#2780),#1899,.F.) ;
#31260=ADVANCED_FACE('',(#2781),#1900,.F.) ;
#31261=ADVANCED_FACE('',(#2782),#1901,.F.) ;
#31262=ADVANCED_FACE('',(#2783),#1902,.F.) ;
#31263=ADVANCED_FACE('',(#2784),#1903,.F.) ;
#31264=ADVANCED_FACE('',(#2785),#1904,.F.) ;
#31265=ADVANCED_FACE('',(#2786),#1905,.F.) ;
#31266=ADVANCED_FACE('',(#2787),#1906,.F.) ;
#31267=ADVANCED_FACE('',(#2788),#1907,.F.) ;
#31268=ADVANCED_FACE('',(#2789),#1908,.F.) ;
#31269=ADVANCED_FACE('',(#2790),#1909,.F.) ;
#31270=ADVANCED_FACE('',(#2791),#1910,.F.) ;
#31271=ADVANCED_FACE('',(#2792),#1911,.F.) ;
#31272=ADVANCED_FACE('',(#2793),#1912,.F.) ;
#31273=ADVANCED_FACE('',(#2794),#1913,.F.) ;
#31274=ADVANCED_FACE('',(#2795),#1914,.F.) ;
#31275=ADVANCED_FACE('',(#2796),#1915,.F.) ;
#31276=ADVANCED_FACE('',(#2797),#1916,.F.) ;
#31277=ADVANCED_FACE('',(#2798),#1917,.F.) ;
#31278=ADVANCED_FACE('',(#2799),#1918,.F.) ;
#31279=ADVANCED_FACE('',(#2800),#1919,.F.) ;
#31280=ADVANCED_FACE('',(#2801),#1920,.F.) ;
#31281=ADVANCED_FACE('',(#2802),#1921,.F.) ;
#31282=ADVANCED_FACE('',(#2803),#1922,.F.) ;
#31283=ADVANCED_FACE('',(#2804),#1923,.F.) ;
#31284=ADVANCED_FACE('',(#2805),#1924,.F.) ;
#31285=ADVANCED_FACE('',(#2806),#1925,.F.) ;
#31286=ADVANCED_FACE('',(#2807),#1926,.F.) ;
#31287=ADVANCED_FACE('',(#2808),#1927,.F.) ;
#31288=ADVANCED_FACE('',(#2809),#1928,.F.) ;
#31289=ADVANCED_FACE('',(#2810),#1929,.F.) ;
#31290=ADVANCED_FACE('',(#2811),#1930,.F.) ;
#31291=ADVANCED_FACE('',(#2812),#1931,.F.) ;
#31292=ADVANCED_FACE('',(#2813),#1932,.F.) ;
#31293=ADVANCED_FACE('',(#2814),#1933,.F.) ;
#31294=ADVANCED_FACE('',(#2815),#1934,.F.) ;
#31295=ADVANCED_FACE('',(#2816),#1935,.T.) ;
#31296=ADVANCED_FACE('',(#2817),#239,.T.) ;
#31297=ADVANCED_FACE('',(#2818),#30195,.F.) ;
#31298=ADVANCED_FACE('',(#2819,#1115,#1116),#1936,.T.) ;
#31299=ADVANCED_FACE('',(#2820),#240,.T.) ;
#31300=ADVANCED_FACE('',(#2821),#30196,.F.) ;
#31301=ADVANCED_FACE('',(#2822,#1117,#1118),#1937,.T.) ;
#31302=ADVANCED_FACE('',(#2823),#241,.T.) ;
#31303=ADVANCED_FACE('',(#2824),#30197,.F.) ;
#31304=ADVANCED_FACE('',(#2825,#1119,#1120),#1938,.T.) ;
#31305=ADVANCED_FACE('',(#2826),#242,.T.) ;
#31306=ADVANCED_FACE('',(#2827),#30198,.F.) ;
#31307=ADVANCED_FACE('',(#2828,#1121,#1122),#1939,.T.) ;
#31308=ADVANCED_FACE('',(#2829),#243,.T.) ;
#31309=ADVANCED_FACE('',(#2830),#30199,.F.) ;
#31310=ADVANCED_FACE('',(#2831,#1123,#1124),#1940,.T.) ;
#31311=ADVANCED_FACE('',(#2832),#244,.T.) ;
#31312=ADVANCED_FACE('',(#2833),#30200,.F.) ;
#31313=ADVANCED_FACE('',(#2834,#1125,#1126),#1941,.T.) ;
#31314=ADVANCED_FACE('',(#2835),#245,.T.) ;
#31315=ADVANCED_FACE('',(#2836),#30201,.F.) ;
#31316=ADVANCED_FACE('',(#2837,#1127,#1128),#1942,.T.) ;
#31317=ADVANCED_FACE('',(#2838),#246,.T.) ;
#31318=ADVANCED_FACE('',(#2839),#30202,.F.) ;
#31319=ADVANCED_FACE('',(#2840,#1129,#1130),#1943,.T.) ;
#31320=ADVANCED_FACE('',(#2841),#247,.T.) ;
#31321=ADVANCED_FACE('',(#2842,#1131,#1132),#1944,.T.) ;
#31322=ADVANCED_FACE('',(#2843),#30203,.F.) ;
#31323=ADVANCED_FACE('',(#2844,#1133),#1945,.F.) ;
#31324=ADVANCED_FACE('',(#2845,#1134),#1946,.F.) ;
#31325=ADVANCED_FACE('',(#2846,#1135),#1947,.F.) ;
#31326=ADVANCED_FACE('',(#2847,#1136),#1948,.F.) ;
#31327=ADVANCED_FACE('',(#2848,#1137),#1949,.F.) ;
#31328=ADVANCED_FACE('',(#2849,#1138),#1950,.F.) ;
#31329=ADVANCED_FACE('',(#2850,#1139),#1951,.F.) ;
#31330=ADVANCED_FACE('',(#2851,#1140),#1952,.F.) ;
#31331=ADVANCED_FACE('',(#2852),#30204,.T.) ;
#31332=ADVANCED_FACE('',(#2853),#248,.T.) ;
#31333=ADVANCED_FACE('',(#2854),#30205,.T.) ;
#31334=ADVANCED_FACE('',(#2855),#249,.T.) ;
#31335=ADVANCED_FACE('',(#2856),#30206,.T.) ;
#31336=ADVANCED_FACE('',(#2857),#250,.T.) ;
#31337=ADVANCED_FACE('',(#2858),#30207,.T.) ;
#31338=ADVANCED_FACE('',(#2859),#251,.T.) ;
#31339=ADVANCED_FACE('',(#2860),#30208,.F.) ;
#31340=ADVANCED_FACE('',(#2861),#1953,.F.) ;
#31341=ADVANCED_FACE('',(#2862),#30209,.F.) ;
#31342=ADVANCED_FACE('',(#2863),#1954,.F.) ;
#31343=ADVANCED_FACE('',(#2864),#30210,.T.) ;
#31344=ADVANCED_FACE('',(#2865),#252,.T.) ;
#31345=ADVANCED_FACE('',(#2866),#30211,.T.) ;
#31346=ADVANCED_FACE('',(#2867),#253,.T.) ;
#31347=ADVANCED_FACE('',(#2868),#30212,.T.) ;
#31348=ADVANCED_FACE('',(#2869),#254,.T.) ;
#31349=ADVANCED_FACE('',(#2870),#30213,.T.) ;
#31350=ADVANCED_FACE('',(#2871),#255,.T.) ;
#31351=ADVANCED_FACE('',(#2872),#30214,.F.) ;
#31352=ADVANCED_FACE('',(#2873),#1955,.F.) ;
#31353=ADVANCED_FACE('',(#2874),#30215,.F.) ;
#31354=ADVANCED_FACE('',(#2875),#1956,.F.) ;
#31355=ADVANCED_FACE('',(#2876),#30216,.T.) ;
#31356=ADVANCED_FACE('',(#2877),#256,.T.) ;
#31357=ADVANCED_FACE('',(#2878),#30217,.T.) ;
#31358=ADVANCED_FACE('',(#2879),#257,.T.) ;
#31359=ADVANCED_FACE('',(#2880),#30218,.T.) ;
#31360=ADVANCED_FACE('',(#2881),#258,.T.) ;
#31361=ADVANCED_FACE('',(#2882),#30219,.T.) ;
#31362=ADVANCED_FACE('',(#2883),#259,.T.) ;
#31363=ADVANCED_FACE('',(#2884),#30220,.F.) ;
#31364=ADVANCED_FACE('',(#2885),#1957,.F.) ;
#31365=ADVANCED_FACE('',(#2886),#30221,.F.) ;
#31366=ADVANCED_FACE('',(#2887),#1958,.F.) ;
#31367=ADVANCED_FACE('',(#2888),#30222,.T.) ;
#31368=ADVANCED_FACE('',(#2889),#260,.T.) ;
#31369=ADVANCED_FACE('',(#2890),#30223,.T.) ;
#31370=ADVANCED_FACE('',(#2891),#261,.T.) ;
#31371=ADVANCED_FACE('',(#2892),#30224,.T.) ;
#31372=ADVANCED_FACE('',(#2893),#262,.T.) ;
#31373=ADVANCED_FACE('',(#2894),#30225,.T.) ;
#31374=ADVANCED_FACE('',(#2895),#263,.T.) ;
#31375=ADVANCED_FACE('',(#2896),#30226,.F.) ;
#31376=ADVANCED_FACE('',(#2897),#1959,.F.) ;
#31377=ADVANCED_FACE('',(#2898),#30227,.F.) ;
#31378=ADVANCED_FACE('',(#2899),#1960,.F.) ;
#31379=ADVANCED_FACE('',(#2900),#30228,.T.) ;
#31380=ADVANCED_FACE('',(#2901),#264,.T.) ;
#31381=ADVANCED_FACE('',(#2902),#30229,.T.) ;
#31382=ADVANCED_FACE('',(#2903),#265,.T.) ;
#31383=ADVANCED_FACE('',(#2904),#30230,.T.) ;
#31384=ADVANCED_FACE('',(#2905),#266,.T.) ;
#31385=ADVANCED_FACE('',(#2906),#30231,.T.) ;
#31386=ADVANCED_FACE('',(#2907),#267,.T.) ;
#31387=ADVANCED_FACE('',(#2908),#30232,.F.) ;
#31388=ADVANCED_FACE('',(#2909),#1961,.F.) ;
#31389=ADVANCED_FACE('',(#2910),#30233,.F.) ;
#31390=ADVANCED_FACE('',(#2911),#1962,.F.) ;
#31391=ADVANCED_FACE('',(#2912),#30234,.T.) ;
#31392=ADVANCED_FACE('',(#2913),#268,.T.) ;
#31393=ADVANCED_FACE('',(#2914),#30235,.T.) ;
#31394=ADVANCED_FACE('',(#2915),#269,.T.) ;
#31395=ADVANCED_FACE('',(#2916),#30236,.T.) ;
#31396=ADVANCED_FACE('',(#2917),#270,.T.) ;
#31397=ADVANCED_FACE('',(#2918),#30237,.T.) ;
#31398=ADVANCED_FACE('',(#2919),#271,.T.) ;
#31399=ADVANCED_FACE('',(#2920),#30238,.F.) ;
#31400=ADVANCED_FACE('',(#2921),#1963,.F.) ;
#31401=ADVANCED_FACE('',(#2922),#30239,.F.) ;
#31402=ADVANCED_FACE('',(#2923),#1964,.F.) ;
#31403=ADVANCED_FACE('',(#2924),#30240,.T.) ;
#31404=ADVANCED_FACE('',(#2925),#272,.T.) ;
#31405=ADVANCED_FACE('',(#2926),#30241,.T.) ;
#31406=ADVANCED_FACE('',(#2927),#273,.T.) ;
#31407=ADVANCED_FACE('',(#2928),#30242,.T.) ;
#31408=ADVANCED_FACE('',(#2929),#274,.T.) ;
#31409=ADVANCED_FACE('',(#2930),#30243,.T.) ;
#31410=ADVANCED_FACE('',(#2931),#275,.T.) ;
#31411=ADVANCED_FACE('',(#2932),#30244,.F.) ;
#31412=ADVANCED_FACE('',(#2933),#1965,.F.) ;
#31413=ADVANCED_FACE('',(#2934),#30245,.F.) ;
#31414=ADVANCED_FACE('',(#2935),#1966,.F.) ;
#31415=ADVANCED_FACE('',(#2936),#30246,.T.) ;
#31416=ADVANCED_FACE('',(#2937),#276,.T.) ;
#31417=ADVANCED_FACE('',(#2938),#30247,.T.) ;
#31418=ADVANCED_FACE('',(#2939),#277,.T.) ;
#31419=ADVANCED_FACE('',(#2940),#30248,.T.) ;
#31420=ADVANCED_FACE('',(#2941),#278,.T.) ;
#31421=ADVANCED_FACE('',(#2942),#30249,.T.) ;
#31422=ADVANCED_FACE('',(#2943),#279,.T.) ;
#31423=ADVANCED_FACE('',(#2944),#30250,.F.) ;
#31424=ADVANCED_FACE('',(#2945),#1967,.F.) ;
#31425=ADVANCED_FACE('',(#2946),#30251,.F.) ;
#31426=ADVANCED_FACE('',(#2947),#1968,.F.) ;
#31427=ADVANCED_FACE('',(#2948),#30252,.T.) ;
#31428=ADVANCED_FACE('',(#2949),#280,.T.) ;
#31429=ADVANCED_FACE('',(#2950),#30253,.T.) ;
#31430=ADVANCED_FACE('',(#2951),#281,.T.) ;
#31431=ADVANCED_FACE('',(#2952),#30254,.T.) ;
#31432=ADVANCED_FACE('',(#2953),#282,.T.) ;
#31433=ADVANCED_FACE('',(#2954),#30255,.T.) ;
#31434=ADVANCED_FACE('',(#2955),#283,.T.) ;
#31435=ADVANCED_FACE('',(#2956),#30256,.F.) ;
#31436=ADVANCED_FACE('',(#2957),#1969,.F.) ;
#31437=ADVANCED_FACE('',(#2958),#30257,.F.) ;
#31438=ADVANCED_FACE('',(#2959),#1970,.F.) ;
#31439=ADVANCED_FACE('',(#2960),#30258,.T.) ;
#31440=ADVANCED_FACE('',(#2961),#284,.T.) ;
#31441=ADVANCED_FACE('',(#2962),#30259,.T.) ;
#31442=ADVANCED_FACE('',(#2963),#285,.T.) ;
#31443=ADVANCED_FACE('',(#2964),#30260,.T.) ;
#31444=ADVANCED_FACE('',(#2965),#286,.T.) ;
#31445=ADVANCED_FACE('',(#2966),#30261,.T.) ;
#31446=ADVANCED_FACE('',(#2967),#287,.T.) ;
#31447=ADVANCED_FACE('',(#2968),#30262,.F.) ;
#31448=ADVANCED_FACE('',(#2969),#1971,.F.) ;
#31449=ADVANCED_FACE('',(#2970),#30263,.F.) ;
#31450=ADVANCED_FACE('',(#2971),#1972,.F.) ;
#31451=ADVANCED_FACE('',(#2972),#30264,.T.) ;
#31452=ADVANCED_FACE('',(#2973),#288,.T.) ;
#31453=ADVANCED_FACE('',(#2974),#30265,.T.) ;
#31454=ADVANCED_FACE('',(#2975),#289,.T.) ;
#31455=ADVANCED_FACE('',(#2976),#30266,.T.) ;
#31456=ADVANCED_FACE('',(#2977),#290,.T.) ;
#31457=ADVANCED_FACE('',(#2978),#30267,.T.) ;
#31458=ADVANCED_FACE('',(#2979),#291,.T.) ;
#31459=ADVANCED_FACE('',(#2980),#30268,.F.) ;
#31460=ADVANCED_FACE('',(#2981),#1973,.F.) ;
#31461=ADVANCED_FACE('',(#2982),#30269,.F.) ;
#31462=ADVANCED_FACE('',(#2983),#1974,.F.) ;
#31463=ADVANCED_FACE('',(#2984),#30270,.T.) ;
#31464=ADVANCED_FACE('',(#2985),#292,.T.) ;
#31465=ADVANCED_FACE('',(#2986),#30271,.T.) ;
#31466=ADVANCED_FACE('',(#2987),#293,.T.) ;
#31467=ADVANCED_FACE('',(#2988),#30272,.T.) ;
#31468=ADVANCED_FACE('',(#2989),#294,.T.) ;
#31469=ADVANCED_FACE('',(#2990),#30273,.T.) ;
#31470=ADVANCED_FACE('',(#2991),#295,.T.) ;
#31471=ADVANCED_FACE('',(#2992),#30274,.F.) ;
#31472=ADVANCED_FACE('',(#2993),#1975,.F.) ;
#31473=ADVANCED_FACE('',(#2994),#30275,.F.) ;
#31474=ADVANCED_FACE('',(#2995),#1976,.F.) ;
#31475=ADVANCED_FACE('',(#2996),#30276,.T.) ;
#31476=ADVANCED_FACE('',(#2997),#296,.T.) ;
#31477=ADVANCED_FACE('',(#2998),#30277,.T.) ;
#31478=ADVANCED_FACE('',(#2999),#297,.T.) ;
#31479=ADVANCED_FACE('',(#3000),#30278,.T.) ;
#31480=ADVANCED_FACE('',(#3001),#298,.T.) ;
#31481=ADVANCED_FACE('',(#3002),#30279,.T.) ;
#31482=ADVANCED_FACE('',(#3003),#299,.T.) ;
#31483=ADVANCED_FACE('',(#3004),#30280,.F.) ;
#31484=ADVANCED_FACE('',(#3005),#1977,.F.) ;
#31485=ADVANCED_FACE('',(#3006),#30281,.F.) ;
#31486=ADVANCED_FACE('',(#3007),#1978,.F.) ;
#31487=ADVANCED_FACE('',(#3008),#30282,.T.) ;
#31488=ADVANCED_FACE('',(#3009),#300,.T.) ;
#31489=ADVANCED_FACE('',(#3010),#30283,.T.) ;
#31490=ADVANCED_FACE('',(#3011),#301,.T.) ;
#31491=ADVANCED_FACE('',(#3012),#30284,.T.) ;
#31492=ADVANCED_FACE('',(#3013),#302,.T.) ;
#31493=ADVANCED_FACE('',(#3014),#30285,.T.) ;
#31494=ADVANCED_FACE('',(#3015),#303,.T.) ;
#31495=ADVANCED_FACE('',(#3016),#30286,.F.) ;
#31496=ADVANCED_FACE('',(#3017),#1979,.F.) ;
#31497=ADVANCED_FACE('',(#3018),#30287,.F.) ;
#31498=ADVANCED_FACE('',(#3019),#1980,.F.) ;
#31499=ADVANCED_FACE('',(#3020),#30288,.T.) ;
#31500=ADVANCED_FACE('',(#3021),#304,.T.) ;
#31501=ADVANCED_FACE('',(#3022),#30289,.T.) ;
#31502=ADVANCED_FACE('',(#3023),#305,.T.) ;
#31503=ADVANCED_FACE('',(#3024),#30290,.T.) ;
#31504=ADVANCED_FACE('',(#3025),#306,.T.) ;
#31505=ADVANCED_FACE('',(#3026),#30291,.T.) ;
#31506=ADVANCED_FACE('',(#3027),#307,.T.) ;
#31507=ADVANCED_FACE('',(#3028),#30292,.F.) ;
#31508=ADVANCED_FACE('',(#3029),#1981,.F.) ;
#31509=ADVANCED_FACE('',(#3030),#30293,.F.) ;
#31510=ADVANCED_FACE('',(#3031),#1982,.F.) ;
#31511=ADVANCED_FACE('',(#3032),#30294,.T.) ;
#31512=ADVANCED_FACE('',(#3033),#308,.T.) ;
#31513=ADVANCED_FACE('',(#3034),#30295,.T.) ;
#31514=ADVANCED_FACE('',(#3035),#309,.T.) ;
#31515=ADVANCED_FACE('',(#3036),#30296,.T.) ;
#31516=ADVANCED_FACE('',(#3037),#310,.T.) ;
#31517=ADVANCED_FACE('',(#3038),#30297,.T.) ;
#31518=ADVANCED_FACE('',(#3039),#311,.T.) ;
#31519=ADVANCED_FACE('',(#3040),#30298,.F.) ;
#31520=ADVANCED_FACE('',(#3041),#1983,.F.) ;
#31521=ADVANCED_FACE('',(#3042),#30299,.F.) ;
#31522=ADVANCED_FACE('',(#3043),#1984,.F.) ;
#31523=ADVANCED_FACE('',(#3044),#30300,.T.) ;
#31524=ADVANCED_FACE('',(#3045),#312,.T.) ;
#31525=ADVANCED_FACE('',(#3046),#30301,.T.) ;
#31526=ADVANCED_FACE('',(#3047),#313,.T.) ;
#31527=ADVANCED_FACE('',(#3048),#30302,.T.) ;
#31528=ADVANCED_FACE('',(#3049),#314,.T.) ;
#31529=ADVANCED_FACE('',(#3050),#30303,.T.) ;
#31530=ADVANCED_FACE('',(#3051),#315,.T.) ;
#31531=ADVANCED_FACE('',(#3052),#30304,.F.) ;
#31532=ADVANCED_FACE('',(#3053),#1985,.F.) ;
#31533=ADVANCED_FACE('',(#3054),#30305,.F.) ;
#31534=ADVANCED_FACE('',(#3055),#1986,.F.) ;
#31535=ADVANCED_FACE('',(#3056),#30306,.T.) ;
#31536=ADVANCED_FACE('',(#3057),#316,.T.) ;
#31537=ADVANCED_FACE('',(#3058),#30307,.T.) ;
#31538=ADVANCED_FACE('',(#3059),#317,.T.) ;
#31539=ADVANCED_FACE('',(#3060),#30308,.T.) ;
#31540=ADVANCED_FACE('',(#3061),#318,.T.) ;
#31541=ADVANCED_FACE('',(#3062),#30309,.T.) ;
#31542=ADVANCED_FACE('',(#3063),#319,.T.) ;
#31543=ADVANCED_FACE('',(#3064),#30310,.F.) ;
#31544=ADVANCED_FACE('',(#3065),#1987,.F.) ;
#31545=ADVANCED_FACE('',(#3066),#30311,.F.) ;
#31546=ADVANCED_FACE('',(#3067),#1988,.F.) ;
#31547=ADVANCED_FACE('',(#3068),#30312,.T.) ;
#31548=ADVANCED_FACE('',(#3069),#320,.T.) ;
#31549=ADVANCED_FACE('',(#3070),#30313,.T.) ;
#31550=ADVANCED_FACE('',(#3071),#321,.T.) ;
#31551=ADVANCED_FACE('',(#3072),#30314,.T.) ;
#31552=ADVANCED_FACE('',(#3073),#322,.T.) ;
#31553=ADVANCED_FACE('',(#3074),#30315,.T.) ;
#31554=ADVANCED_FACE('',(#3075),#323,.T.) ;
#31555=ADVANCED_FACE('',(#3076),#30316,.F.) ;
#31556=ADVANCED_FACE('',(#3077),#1989,.F.) ;
#31557=ADVANCED_FACE('',(#3078),#30317,.F.) ;
#31558=ADVANCED_FACE('',(#3079),#1990,.F.) ;
#31559=ADVANCED_FACE('',(#3080),#30318,.T.) ;
#31560=ADVANCED_FACE('',(#3081),#324,.T.) ;
#31561=ADVANCED_FACE('',(#3082),#30319,.T.) ;
#31562=ADVANCED_FACE('',(#3083),#325,.T.) ;
#31563=ADVANCED_FACE('',(#3084),#30320,.T.) ;
#31564=ADVANCED_FACE('',(#3085),#326,.T.) ;
#31565=ADVANCED_FACE('',(#3086),#30321,.T.) ;
#31566=ADVANCED_FACE('',(#3087),#327,.T.) ;
#31567=ADVANCED_FACE('',(#3088),#30322,.F.) ;
#31568=ADVANCED_FACE('',(#3089),#1991,.F.) ;
#31569=ADVANCED_FACE('',(#3090),#30323,.F.) ;
#31570=ADVANCED_FACE('',(#3091),#1992,.F.) ;
#31571=ADVANCED_FACE('',(#3092),#30324,.T.) ;
#31572=ADVANCED_FACE('',(#3093),#328,.T.) ;
#31573=ADVANCED_FACE('',(#3094),#30325,.T.) ;
#31574=ADVANCED_FACE('',(#3095),#329,.T.) ;
#31575=ADVANCED_FACE('',(#3096),#30326,.T.) ;
#31576=ADVANCED_FACE('',(#3097),#330,.T.) ;
#31577=ADVANCED_FACE('',(#3098),#30327,.T.) ;
#31578=ADVANCED_FACE('',(#3099),#331,.T.) ;
#31579=ADVANCED_FACE('',(#3100),#30328,.F.) ;
#31580=ADVANCED_FACE('',(#3101),#1993,.F.) ;
#31581=ADVANCED_FACE('',(#3102),#30329,.F.) ;
#31582=ADVANCED_FACE('',(#3103),#1994,.F.) ;
#31583=ADVANCED_FACE('',(#3104),#30330,.T.) ;
#31584=ADVANCED_FACE('',(#3105),#332,.T.) ;
#31585=ADVANCED_FACE('',(#3106),#30331,.T.) ;
#31586=ADVANCED_FACE('',(#3107),#333,.T.) ;
#31587=ADVANCED_FACE('',(#3108),#30332,.T.) ;
#31588=ADVANCED_FACE('',(#3109),#334,.T.) ;
#31589=ADVANCED_FACE('',(#3110),#30333,.T.) ;
#31590=ADVANCED_FACE('',(#3111),#335,.T.) ;
#31591=ADVANCED_FACE('',(#3112),#30334,.F.) ;
#31592=ADVANCED_FACE('',(#3113),#1995,.F.) ;
#31593=ADVANCED_FACE('',(#3114),#30335,.F.) ;
#31594=ADVANCED_FACE('',(#3115),#1996,.F.) ;
#31595=ADVANCED_FACE('',(#3116),#30336,.T.) ;
#31596=ADVANCED_FACE('',(#3117),#336,.T.) ;
#31597=ADVANCED_FACE('',(#3118),#30337,.T.) ;
#31598=ADVANCED_FACE('',(#3119),#337,.T.) ;
#31599=ADVANCED_FACE('',(#3120),#30338,.T.) ;
#31600=ADVANCED_FACE('',(#3121),#338,.T.) ;
#31601=ADVANCED_FACE('',(#3122),#30339,.T.) ;
#31602=ADVANCED_FACE('',(#3123),#339,.T.) ;
#31603=ADVANCED_FACE('',(#3124),#30340,.F.) ;
#31604=ADVANCED_FACE('',(#3125),#1997,.F.) ;
#31605=ADVANCED_FACE('',(#3126),#30341,.F.) ;
#31606=ADVANCED_FACE('',(#3127),#1998,.F.) ;
#31607=ADVANCED_FACE('',(#3128),#30342,.T.) ;
#31608=ADVANCED_FACE('',(#3129),#340,.T.) ;
#31609=ADVANCED_FACE('',(#3130),#30343,.T.) ;
#31610=ADVANCED_FACE('',(#3131),#341,.T.) ;
#31611=ADVANCED_FACE('',(#3132),#30344,.T.) ;
#31612=ADVANCED_FACE('',(#3133),#342,.T.) ;
#31613=ADVANCED_FACE('',(#3134),#30345,.T.) ;
#31614=ADVANCED_FACE('',(#3135),#343,.T.) ;
#31615=ADVANCED_FACE('',(#3136),#30346,.F.) ;
#31616=ADVANCED_FACE('',(#3137),#1999,.F.) ;
#31617=ADVANCED_FACE('',(#3138),#30347,.F.) ;
#31618=ADVANCED_FACE('',(#3139),#2000,.F.) ;
#31619=ADVANCED_FACE('',(#3140),#30348,.T.) ;
#31620=ADVANCED_FACE('',(#3141),#344,.T.) ;
#31621=ADVANCED_FACE('',(#3142),#30349,.T.) ;
#31622=ADVANCED_FACE('',(#3143),#345,.T.) ;
#31623=ADVANCED_FACE('',(#3144),#30350,.T.) ;
#31624=ADVANCED_FACE('',(#3145),#346,.T.) ;
#31625=ADVANCED_FACE('',(#3146),#30351,.T.) ;
#31626=ADVANCED_FACE('',(#3147),#347,.T.) ;
#31627=ADVANCED_FACE('',(#3148),#30352,.F.) ;
#31628=ADVANCED_FACE('',(#3149),#2001,.F.) ;
#31629=ADVANCED_FACE('',(#3150),#30353,.F.) ;
#31630=ADVANCED_FACE('',(#3151),#2002,.F.) ;
#31631=ADVANCED_FACE('',(#3152),#30354,.T.) ;
#31632=ADVANCED_FACE('',(#3153),#348,.T.) ;
#31633=ADVANCED_FACE('',(#3154),#30355,.T.) ;
#31634=ADVANCED_FACE('',(#3155),#349,.T.) ;
#31635=ADVANCED_FACE('',(#3156),#30356,.T.) ;
#31636=ADVANCED_FACE('',(#3157),#350,.T.) ;
#31637=ADVANCED_FACE('',(#3158),#30357,.T.) ;
#31638=ADVANCED_FACE('',(#3159),#351,.T.) ;
#31639=ADVANCED_FACE('',(#3160),#30358,.F.) ;
#31640=ADVANCED_FACE('',(#3161),#2003,.F.) ;
#31641=ADVANCED_FACE('',(#3162),#30359,.F.) ;
#31642=ADVANCED_FACE('',(#3163),#2004,.F.) ;
#31643=ADVANCED_FACE('',(#3164,#1141,#1142,#1143),#2005,.T.) ;
#31644=ADVANCED_FACE('',(#3165),#30360,.T.) ;
#31645=ADVANCED_FACE('',(#3166),#352,.T.) ;
#31646=ADVANCED_FACE('',(#3167),#30361,.T.) ;
#31647=ADVANCED_FACE('',(#3168),#353,.T.) ;
#31648=ADVANCED_FACE('',(#3169),#30362,.T.) ;
#31649=ADVANCED_FACE('',(#3170),#354,.T.) ;
#31650=ADVANCED_FACE('',(#3171),#30363,.T.) ;
#31651=ADVANCED_FACE('',(#3172),#355,.T.) ;
#31652=ADVANCED_FACE('',(#3173),#30364,.F.) ;
#31653=ADVANCED_FACE('',(#3174),#2006,.F.) ;
#31654=ADVANCED_FACE('',(#3175),#30365,.F.) ;
#31655=ADVANCED_FACE('',(#3176),#2007,.F.) ;
#31656=ADVANCED_FACE('',(#3177),#2008,.F.) ;
#31657=ADVANCED_FACE('',(#3178),#30366,.F.) ;
#31658=ADVANCED_FACE('',(#3179),#30367,.F.) ;
#31659=ADVANCED_FACE('',(#3180),#2009,.F.) ;
#31660=ADVANCED_FACE('',(#3181),#30368,.F.) ;
#31661=ADVANCED_FACE('',(#3182),#30369,.F.) ;
#31662=ADVANCED_FACE('',(#3183),#2010,.F.) ;
#31663=ADVANCED_FACE('',(#3184,#1144),#2011,.F.) ;
#31664=ADVANCED_FACE('',(#3185),#30370,.F.) ;
#31665=ADVANCED_FACE('',(#3186),#30371,.F.) ;
#31666=ADVANCED_FACE('',(#3187),#356,.F.) ;
#31667=ADVANCED_FACE('',(#3188),#30372,.F.) ;
#31668=ADVANCED_FACE('',(#3189),#357,.F.) ;
#31669=ADVANCED_FACE('',(#3190),#358,.F.) ;
#31670=ADVANCED_FACE('',(#3191),#30373,.F.) ;
#31671=ADVANCED_FACE('',(#3192),#30374,.F.) ;
#31672=ADVANCED_FACE('',(#3193),#359,.F.) ;
#31673=ADVANCED_FACE('',(#3194),#30375,.F.) ;
#31674=ADVANCED_FACE('',(#3195),#30376,.T.) ;
#31675=ADVANCED_FACE('',(#3196),#30377,.F.) ;
#31676=ADVANCED_FACE('',(#3197),#30378,.T.) ;
#31677=ADVANCED_FACE('',(#3198),#11,.F.) ;
#31678=ADVANCED_FACE('',(#3199),#12,.F.) ;
#31679=ADVANCED_FACE('',(#3200),#30379,.F.) ;
#31680=ADVANCED_FACE('',(#3201),#13,.F.) ;
#31681=ADVANCED_FACE('',(#3202),#14,.F.) ;
#31682=ADVANCED_FACE('',(#3203),#2012,.F.) ;
#31683=ADVANCED_FACE('',(#3204),#2013,.F.) ;
#31684=ADVANCED_FACE('',(#3205),#2014,.F.) ;
#31685=ADVANCED_FACE('',(#3206),#2015,.F.) ;
#31686=ADVANCED_FACE('',(#3207),#15,.F.) ;
#31687=ADVANCED_FACE('',(#3208),#16,.F.) ;
#31688=ADVANCED_FACE('',(#3209),#30380,.F.) ;
#31689=ADVANCED_FACE('',(#3210),#30381,.F.) ;
#31690=ADVANCED_FACE('',(#3211),#30382,.F.) ;
#31691=ADVANCED_FACE('',(#3212),#30383,.F.) ;
#31692=ADVANCED_FACE('',(#3213),#17,.F.) ;
#31693=ADVANCED_FACE('',(#3214),#18,.F.) ;
#31694=ADVANCED_FACE('',(#3215),#30384,.F.) ;
#31695=ADVANCED_FACE('',(#3216),#30385,.F.) ;
#31696=ADVANCED_FACE('',(#3217),#360,.F.) ;
#31697=ADVANCED_FACE('',(#3218),#30386,.F.) ;
#31698=ADVANCED_FACE('',(#3219),#361,.F.) ;
#31699=ADVANCED_FACE('',(#3220),#362,.F.) ;
#31700=ADVANCED_FACE('',(#3221),#30387,.F.) ;
#31701=ADVANCED_FACE('',(#3222),#30388,.F.) ;
#31702=ADVANCED_FACE('',(#3223),#363,.F.) ;
#31703=ADVANCED_FACE('',(#3224),#30389,.F.) ;
#31704=ADVANCED_FACE('',(#3225),#30390,.T.) ;
#31705=ADVANCED_FACE('',(#3226),#30391,.F.) ;
#31706=ADVANCED_FACE('',(#3227),#30392,.T.) ;
#31707=ADVANCED_FACE('',(#3228),#19,.F.) ;
#31708=ADVANCED_FACE('',(#3229),#20,.F.) ;
#31709=ADVANCED_FACE('',(#3230),#30393,.F.) ;
#31710=ADVANCED_FACE('',(#3231),#21,.F.) ;
#31711=ADVANCED_FACE('',(#3232),#22,.F.) ;
#31712=ADVANCED_FACE('',(#3233),#2016,.F.) ;
#31713=ADVANCED_FACE('',(#3234),#2017,.F.) ;
#31714=ADVANCED_FACE('',(#3235),#2018,.F.) ;
#31715=ADVANCED_FACE('',(#3236),#2019,.F.) ;
#31716=ADVANCED_FACE('',(#3237),#23,.F.) ;
#31717=ADVANCED_FACE('',(#3238),#24,.F.) ;
#31718=ADVANCED_FACE('',(#3239),#30394,.F.) ;
#31719=ADVANCED_FACE('',(#3240),#30395,.F.) ;
#31720=ADVANCED_FACE('',(#3241),#30396,.F.) ;
#31721=ADVANCED_FACE('',(#3242),#30397,.F.) ;
#31722=ADVANCED_FACE('',(#3243),#25,.F.) ;
#31723=ADVANCED_FACE('',(#3244),#26,.F.) ;
#31724=ADVANCED_FACE('',(#3245),#30398,.F.) ;
#31725=ADVANCED_FACE('',(#3246),#30399,.F.) ;
#31726=ADVANCED_FACE('',(#3247),#364,.F.) ;
#31727=ADVANCED_FACE('',(#3248),#30400,.F.) ;
#31728=ADVANCED_FACE('',(#3249),#365,.F.) ;
#31729=ADVANCED_FACE('',(#3250),#366,.F.) ;
#31730=ADVANCED_FACE('',(#3251),#30401,.F.) ;
#31731=ADVANCED_FACE('',(#3252),#30402,.F.) ;
#31732=ADVANCED_FACE('',(#3253),#367,.F.) ;
#31733=ADVANCED_FACE('',(#3254),#30403,.F.) ;
#31734=ADVANCED_FACE('',(#3255),#30404,.T.) ;
#31735=ADVANCED_FACE('',(#3256),#30405,.F.) ;
#31736=ADVANCED_FACE('',(#3257),#30406,.T.) ;
#31737=ADVANCED_FACE('',(#3258),#27,.F.) ;
#31738=ADVANCED_FACE('',(#3259),#28,.F.) ;
#31739=ADVANCED_FACE('',(#3260),#30407,.F.) ;
#31740=ADVANCED_FACE('',(#3261),#29,.F.) ;
#31741=ADVANCED_FACE('',(#3262),#30,.F.) ;
#31742=ADVANCED_FACE('',(#3263),#2020,.F.) ;
#31743=ADVANCED_FACE('',(#3264),#2021,.F.) ;
#31744=ADVANCED_FACE('',(#3265),#2022,.F.) ;
#31745=ADVANCED_FACE('',(#3266),#2023,.F.) ;
#31746=ADVANCED_FACE('',(#3267),#31,.F.) ;
#31747=ADVANCED_FACE('',(#3268),#32,.F.) ;
#31748=ADVANCED_FACE('',(#3269),#30408,.F.) ;
#31749=ADVANCED_FACE('',(#3270),#30409,.F.) ;
#31750=ADVANCED_FACE('',(#3271),#30410,.F.) ;
#31751=ADVANCED_FACE('',(#3272),#30411,.F.) ;
#31752=ADVANCED_FACE('',(#3273),#33,.F.) ;
#31753=ADVANCED_FACE('',(#3274),#34,.F.) ;
#31754=ADVANCED_FACE('',(#3275),#30412,.F.) ;
#31755=ADVANCED_FACE('',(#3276),#30413,.F.) ;
#31756=ADVANCED_FACE('',(#3277),#368,.F.) ;
#31757=ADVANCED_FACE('',(#3278),#30414,.F.) ;
#31758=ADVANCED_FACE('',(#3279),#369,.F.) ;
#31759=ADVANCED_FACE('',(#3280),#370,.F.) ;
#31760=ADVANCED_FACE('',(#3281),#30415,.F.) ;
#31761=ADVANCED_FACE('',(#3282),#30416,.F.) ;
#31762=ADVANCED_FACE('',(#3283),#371,.F.) ;
#31763=ADVANCED_FACE('',(#3284),#30417,.F.) ;
#31764=ADVANCED_FACE('',(#3285),#30418,.T.) ;
#31765=ADVANCED_FACE('',(#3286),#30419,.F.) ;
#31766=ADVANCED_FACE('',(#3287),#30420,.T.) ;
#31767=ADVANCED_FACE('',(#3288),#35,.F.) ;
#31768=ADVANCED_FACE('',(#3289),#36,.F.) ;
#31769=ADVANCED_FACE('',(#3290),#30421,.F.) ;
#31770=ADVANCED_FACE('',(#3291),#37,.F.) ;
#31771=ADVANCED_FACE('',(#3292),#38,.F.) ;
#31772=ADVANCED_FACE('',(#3293),#2024,.F.) ;
#31773=ADVANCED_FACE('',(#3294),#2025,.F.) ;
#31774=ADVANCED_FACE('',(#3295),#2026,.F.) ;
#31775=ADVANCED_FACE('',(#3296),#2027,.F.) ;
#31776=ADVANCED_FACE('',(#3297),#39,.F.) ;
#31777=ADVANCED_FACE('',(#3298),#40,.F.) ;
#31778=ADVANCED_FACE('',(#3299),#30422,.F.) ;
#31779=ADVANCED_FACE('',(#3300),#30423,.F.) ;
#31780=ADVANCED_FACE('',(#3301),#30424,.F.) ;
#31781=ADVANCED_FACE('',(#3302),#30425,.F.) ;
#31782=ADVANCED_FACE('',(#3303),#41,.F.) ;
#31783=ADVANCED_FACE('',(#3304),#42,.F.) ;
#31784=ADVANCED_FACE('',(#3305),#30426,.F.) ;
#31785=ADVANCED_FACE('',(#3306),#30427,.F.) ;
#31786=ADVANCED_FACE('',(#3307),#372,.F.) ;
#31787=ADVANCED_FACE('',(#3308),#30428,.F.) ;
#31788=ADVANCED_FACE('',(#3309),#373,.F.) ;
#31789=ADVANCED_FACE('',(#3310),#374,.F.) ;
#31790=ADVANCED_FACE('',(#3311),#30429,.F.) ;
#31791=ADVANCED_FACE('',(#3312),#30430,.F.) ;
#31792=ADVANCED_FACE('',(#3313),#375,.F.) ;
#31793=ADVANCED_FACE('',(#3314),#30431,.F.) ;
#31794=ADVANCED_FACE('',(#3315),#30432,.T.) ;
#31795=ADVANCED_FACE('',(#3316),#30433,.F.) ;
#31796=ADVANCED_FACE('',(#3317),#30434,.T.) ;
#31797=ADVANCED_FACE('',(#3318),#43,.F.) ;
#31798=ADVANCED_FACE('',(#3319),#44,.F.) ;
#31799=ADVANCED_FACE('',(#3320),#30435,.F.) ;
#31800=ADVANCED_FACE('',(#3321),#45,.F.) ;
#31801=ADVANCED_FACE('',(#3322),#46,.F.) ;
#31802=ADVANCED_FACE('',(#3323),#2028,.F.) ;
#31803=ADVANCED_FACE('',(#3324),#2029,.F.) ;
#31804=ADVANCED_FACE('',(#3325),#2030,.F.) ;
#31805=ADVANCED_FACE('',(#3326),#2031,.F.) ;
#31806=ADVANCED_FACE('',(#3327),#47,.F.) ;
#31807=ADVANCED_FACE('',(#3328),#48,.F.) ;
#31808=ADVANCED_FACE('',(#3329),#30436,.F.) ;
#31809=ADVANCED_FACE('',(#3330),#30437,.F.) ;
#31810=ADVANCED_FACE('',(#3331),#30438,.F.) ;
#31811=ADVANCED_FACE('',(#3332),#30439,.F.) ;
#31812=ADVANCED_FACE('',(#3333),#49,.F.) ;
#31813=ADVANCED_FACE('',(#3334),#50,.F.) ;
#31814=ADVANCED_FACE('',(#3335),#30440,.F.) ;
#31815=ADVANCED_FACE('',(#3336),#30441,.F.) ;
#31816=ADVANCED_FACE('',(#3337),#376,.F.) ;
#31817=ADVANCED_FACE('',(#3338),#30442,.F.) ;
#31818=ADVANCED_FACE('',(#3339),#377,.F.) ;
#31819=ADVANCED_FACE('',(#3340),#378,.F.) ;
#31820=ADVANCED_FACE('',(#3341),#30443,.F.) ;
#31821=ADVANCED_FACE('',(#3342),#30444,.F.) ;
#31822=ADVANCED_FACE('',(#3343),#379,.F.) ;
#31823=ADVANCED_FACE('',(#3344),#30445,.F.) ;
#31824=ADVANCED_FACE('',(#3345),#30446,.T.) ;
#31825=ADVANCED_FACE('',(#3346),#30447,.F.) ;
#31826=ADVANCED_FACE('',(#3347),#30448,.T.) ;
#31827=ADVANCED_FACE('',(#3348),#51,.F.) ;
#31828=ADVANCED_FACE('',(#3349),#52,.F.) ;
#31829=ADVANCED_FACE('',(#3350),#30449,.F.) ;
#31830=ADVANCED_FACE('',(#3351),#53,.F.) ;
#31831=ADVANCED_FACE('',(#3352),#54,.F.) ;
#31832=ADVANCED_FACE('',(#3353),#2032,.F.) ;
#31833=ADVANCED_FACE('',(#3354),#2033,.F.) ;
#31834=ADVANCED_FACE('',(#3355),#2034,.F.) ;
#31835=ADVANCED_FACE('',(#3356),#2035,.F.) ;
#31836=ADVANCED_FACE('',(#3357),#55,.F.) ;
#31837=ADVANCED_FACE('',(#3358),#56,.F.) ;
#31838=ADVANCED_FACE('',(#3359),#30450,.F.) ;
#31839=ADVANCED_FACE('',(#3360),#30451,.F.) ;
#31840=ADVANCED_FACE('',(#3361),#30452,.F.) ;
#31841=ADVANCED_FACE('',(#3362),#30453,.F.) ;
#31842=ADVANCED_FACE('',(#3363),#57,.F.) ;
#31843=ADVANCED_FACE('',(#3364),#58,.F.) ;
#31844=ADVANCED_FACE('',(#3365),#30454,.F.) ;
#31845=ADVANCED_FACE('',(#3366),#30455,.F.) ;
#31846=ADVANCED_FACE('',(#3367),#380,.F.) ;
#31847=ADVANCED_FACE('',(#3368),#30456,.F.) ;
#31848=ADVANCED_FACE('',(#3369),#381,.F.) ;
#31849=ADVANCED_FACE('',(#3370),#382,.F.) ;
#31850=ADVANCED_FACE('',(#3371),#30457,.F.) ;
#31851=ADVANCED_FACE('',(#3372),#30458,.F.) ;
#31852=ADVANCED_FACE('',(#3373),#383,.F.) ;
#31853=ADVANCED_FACE('',(#3374),#30459,.F.) ;
#31854=ADVANCED_FACE('',(#3375),#30460,.T.) ;
#31855=ADVANCED_FACE('',(#3376),#30461,.F.) ;
#31856=ADVANCED_FACE('',(#3377),#30462,.T.) ;
#31857=ADVANCED_FACE('',(#3378),#59,.F.) ;
#31858=ADVANCED_FACE('',(#3379),#60,.F.) ;
#31859=ADVANCED_FACE('',(#3380),#30463,.F.) ;
#31860=ADVANCED_FACE('',(#3381),#61,.F.) ;
#31861=ADVANCED_FACE('',(#3382),#62,.F.) ;
#31862=ADVANCED_FACE('',(#3383),#2036,.F.) ;
#31863=ADVANCED_FACE('',(#3384),#2037,.F.) ;
#31864=ADVANCED_FACE('',(#3385),#2038,.F.) ;
#31865=ADVANCED_FACE('',(#3386),#2039,.F.) ;
#31866=ADVANCED_FACE('',(#3387),#63,.F.) ;
#31867=ADVANCED_FACE('',(#3388),#64,.F.) ;
#31868=ADVANCED_FACE('',(#3389),#30464,.F.) ;
#31869=ADVANCED_FACE('',(#3390),#30465,.F.) ;
#31870=ADVANCED_FACE('',(#3391),#30466,.F.) ;
#31871=ADVANCED_FACE('',(#3392),#30467,.F.) ;
#31872=ADVANCED_FACE('',(#3393),#65,.F.) ;
#31873=ADVANCED_FACE('',(#3394),#66,.F.) ;
#31874=ADVANCED_FACE('',(#3395),#30468,.F.) ;
#31875=ADVANCED_FACE('',(#3396),#30469,.F.) ;
#31876=ADVANCED_FACE('',(#3397),#384,.F.) ;
#31877=ADVANCED_FACE('',(#3398),#30470,.F.) ;
#31878=ADVANCED_FACE('',(#3399),#385,.F.) ;
#31879=ADVANCED_FACE('',(#3400),#386,.F.) ;
#31880=ADVANCED_FACE('',(#3401),#30471,.F.) ;
#31881=ADVANCED_FACE('',(#3402),#30472,.F.) ;
#31882=ADVANCED_FACE('',(#3403),#387,.F.) ;
#31883=ADVANCED_FACE('',(#3404),#30473,.F.) ;
#31884=ADVANCED_FACE('',(#3405),#30474,.T.) ;
#31885=ADVANCED_FACE('',(#3406),#30475,.F.) ;
#31886=ADVANCED_FACE('',(#3407),#30476,.T.) ;
#31887=ADVANCED_FACE('',(#3408),#67,.F.) ;
#31888=ADVANCED_FACE('',(#3409),#68,.F.) ;
#31889=ADVANCED_FACE('',(#3410),#30477,.F.) ;
#31890=ADVANCED_FACE('',(#3411),#69,.F.) ;
#31891=ADVANCED_FACE('',(#3412),#70,.F.) ;
#31892=ADVANCED_FACE('',(#3413),#2040,.F.) ;
#31893=ADVANCED_FACE('',(#3414),#2041,.F.) ;
#31894=ADVANCED_FACE('',(#3415),#2042,.F.) ;
#31895=ADVANCED_FACE('',(#3416),#2043,.F.) ;
#31896=ADVANCED_FACE('',(#3417),#71,.F.) ;
#31897=ADVANCED_FACE('',(#3418),#72,.F.) ;
#31898=ADVANCED_FACE('',(#3419),#30478,.F.) ;
#31899=ADVANCED_FACE('',(#3420),#30479,.F.) ;
#31900=ADVANCED_FACE('',(#3421),#30480,.F.) ;
#31901=ADVANCED_FACE('',(#3422),#30481,.F.) ;
#31902=ADVANCED_FACE('',(#3423),#73,.F.) ;
#31903=ADVANCED_FACE('',(#3424),#74,.F.) ;
#31904=ADVANCED_FACE('',(#3425),#30482,.F.) ;
#31905=ADVANCED_FACE('',(#3426),#30483,.F.) ;
#31906=ADVANCED_FACE('',(#3427),#388,.F.) ;
#31907=ADVANCED_FACE('',(#3428),#30484,.F.) ;
#31908=ADVANCED_FACE('',(#3429),#389,.F.) ;
#31909=ADVANCED_FACE('',(#3430),#390,.F.) ;
#31910=ADVANCED_FACE('',(#3431),#30485,.F.) ;
#31911=ADVANCED_FACE('',(#3432),#30486,.F.) ;
#31912=ADVANCED_FACE('',(#3433),#391,.F.) ;
#31913=ADVANCED_FACE('',(#3434),#30487,.F.) ;
#31914=ADVANCED_FACE('',(#3435),#30488,.T.) ;
#31915=ADVANCED_FACE('',(#3436),#30489,.F.) ;
#31916=ADVANCED_FACE('',(#3437),#30490,.T.) ;
#31917=ADVANCED_FACE('',(#3438),#75,.F.) ;
#31918=ADVANCED_FACE('',(#3439),#76,.F.) ;
#31919=ADVANCED_FACE('',(#3440),#30491,.F.) ;
#31920=ADVANCED_FACE('',(#3441),#77,.F.) ;
#31921=ADVANCED_FACE('',(#3442),#78,.F.) ;
#31922=ADVANCED_FACE('',(#3443),#2044,.F.) ;
#31923=ADVANCED_FACE('',(#3444),#2045,.F.) ;
#31924=ADVANCED_FACE('',(#3445),#2046,.F.) ;
#31925=ADVANCED_FACE('',(#3446),#2047,.F.) ;
#31926=ADVANCED_FACE('',(#3447),#79,.F.) ;
#31927=ADVANCED_FACE('',(#3448),#80,.F.) ;
#31928=ADVANCED_FACE('',(#3449),#30492,.F.) ;
#31929=ADVANCED_FACE('',(#3450),#30493,.F.) ;
#31930=ADVANCED_FACE('',(#3451),#30494,.F.) ;
#31931=ADVANCED_FACE('',(#3452),#30495,.F.) ;
#31932=ADVANCED_FACE('',(#3453),#81,.F.) ;
#31933=ADVANCED_FACE('',(#3454),#82,.F.) ;
#31934=ADVANCED_FACE('',(#3455),#2048,.F.) ;
#31935=ADVANCED_FACE('',(#3456),#2049,.F.) ;
#31936=ADVANCED_FACE('',(#3457),#2050,.F.) ;
#31937=ADVANCED_FACE('',(#3458),#2051,.F.) ;
#31938=ADVANCED_FACE('',(#3459),#2052,.F.) ;
#31939=ADVANCED_FACE('',(#3460),#2053,.F.) ;
#31940=ADVANCED_FACE('',(#3461),#2054,.F.) ;
#31941=ADVANCED_FACE('',(#3462),#2055,.F.) ;
#31942=ADVANCED_FACE('',(#3463),#2056,.F.) ;
#31943=ADVANCED_FACE('',(#3464),#2057,.F.) ;
#31944=ADVANCED_FACE('',(#3465),#2058,.F.) ;
#31945=ADVANCED_FACE('',(#3466),#2059,.F.) ;
#31946=ADVANCED_FACE('',(#3467),#2060,.F.) ;
#31947=ADVANCED_FACE('',(#3468),#2061,.F.) ;
#31948=ADVANCED_FACE('',(#3469),#2062,.F.) ;
#31949=ADVANCED_FACE('',(#3470),#2063,.F.) ;
#31950=ADVANCED_FACE('',(#3471),#2064,.F.) ;
#31951=ADVANCED_FACE('',(#3472),#2065,.F.) ;
#31952=ADVANCED_FACE('',(#3473),#2066,.F.) ;
#31953=ADVANCED_FACE('',(#3474),#2067,.F.) ;
#31954=ADVANCED_FACE('',(#3475),#2068,.F.) ;
#31955=ADVANCED_FACE('',(#3476),#2069,.F.) ;
#31956=ADVANCED_FACE('',(#3477),#2070,.F.) ;
#31957=ADVANCED_FACE('',(#3478),#2071,.F.) ;
#31958=ADVANCED_FACE('',(#3479),#2072,.F.) ;
#31959=ADVANCED_FACE('',(#3480),#2073,.F.) ;
#31960=ADVANCED_FACE('',(#3481),#2074,.F.) ;
#31961=ADVANCED_FACE('',(#3482),#2075,.F.) ;
#31962=ADVANCED_FACE('',(#3483),#30496,.T.) ;
#31963=ADVANCED_FACE('',(#3484),#2076,.T.) ;
#31964=ADVANCED_FACE('',(#3485),#30497,.T.) ;
#31965=ADVANCED_FACE('',(#3486),#30498,.T.) ;
#31966=ADVANCED_FACE('',(#3487),#30499,.T.) ;
#31967=ADVANCED_FACE('',(#3488),#30500,.T.) ;
#31968=ADVANCED_FACE('',(#3489),#30501,.T.) ;
#31969=ADVANCED_FACE('',(#3490),#30502,.T.) ;
#31970=ADVANCED_FACE('',(#3491),#30503,.T.) ;
#31971=ADVANCED_FACE('',(#3492),#30504,.T.) ;
#31972=ADVANCED_FACE('',(#3493),#2077,.T.) ;
#31973=ADVANCED_FACE('',(#3494),#30505,.T.) ;
#31974=ADVANCED_FACE('',(#3495),#2078,.T.) ;
#31975=ADVANCED_FACE('',(#3496),#2079,.T.) ;
#31976=ADVANCED_FACE('',(#3497),#2080,.T.) ;
#31977=ADVANCED_FACE('',(#3498),#2081,.T.) ;
#31978=ADVANCED_FACE('',(#3499),#2082,.T.) ;
#31979=ADVANCED_FACE('',(#3500),#2083,.T.) ;
#31980=ADVANCED_FACE('',(#3501),#2084,.T.) ;
#31981=ADVANCED_FACE('',(#3502),#2085,.T.) ;
#31982=ADVANCED_FACE('',(#3503),#2086,.T.) ;
#31983=ADVANCED_FACE('',(#3504),#2087,.T.) ;
#31984=ADVANCED_FACE('',(#3505),#2088,.T.) ;
#31985=ADVANCED_FACE('',(#3506),#2089,.T.) ;
#31986=ADVANCED_FACE('',(#3507),#2090,.T.) ;
#31987=ADVANCED_FACE('',(#3508),#2091,.T.) ;
#31988=ADVANCED_FACE('',(#3509),#2092,.T.) ;
#31989=ADVANCED_FACE('',(#3510),#2093,.T.) ;
#31990=ADVANCED_FACE('',(#3511),#2094,.T.) ;
#31991=ADVANCED_FACE('',(#3512),#2095,.F.) ;
#31992=ADVANCED_FACE('',(#3513),#2096,.F.) ;
#31993=ADVANCED_FACE('',(#3514),#2097,.F.) ;
#31994=ADVANCED_FACE('',(#3515),#2098,.F.) ;
#31995=ADVANCED_FACE('',(#3516),#2099,.F.) ;
#31996=ADVANCED_FACE('',(#3517),#2100,.F.) ;
#31997=ADVANCED_FACE('',(#3518),#2101,.F.) ;
#31998=ADVANCED_FACE('',(#3519),#2102,.F.) ;
#31999=ADVANCED_FACE('',(#3520),#2103,.F.) ;
#32000=ADVANCED_FACE('',(#3521),#2104,.F.) ;
#32001=ADVANCED_FACE('',(#3522),#2105,.T.) ;
#32002=ADVANCED_FACE('',(#3523),#2106,.F.) ;
#32003=ADVANCED_FACE('',(#3524),#2107,.F.) ;
#32004=ADVANCED_FACE('',(#3525),#2108,.F.) ;
#32005=ADVANCED_FACE('',(#3526),#2109,.F.) ;
#32006=ADVANCED_FACE('',(#3527),#2110,.F.) ;
#32007=ADVANCED_FACE('',(#3528),#2111,.F.) ;
#32008=ADVANCED_FACE('',(#3529),#2112,.F.) ;
#32009=ADVANCED_FACE('',(#3530),#2113,.F.) ;
#32010=ADVANCED_FACE('',(#3531,#1145,#1146,#1147),#2114,.T.) ;
#32011=ADVANCED_FACE('',(#3532),#392,.T.) ;
#32012=ADVANCED_FACE('',(#3533),#30506,.F.) ;
#32013=ADVANCED_FACE('',(#3534),#393,.F.) ;
#32014=ADVANCED_FACE('',(#3535),#2115,.F.) ;
#32015=ADVANCED_FACE('',(#3536),#30507,.F.) ;
#32016=ADVANCED_FACE('',(#3537,#1148,#1149,#1150),#2116,.T.) ;
#32017=ADVANCED_FACE('',(#3538),#394,.T.) ;
#32018=ADVANCED_FACE('',(#3539),#30508,.F.) ;
#32019=ADVANCED_FACE('',(#3540),#395,.F.) ;
#32020=ADVANCED_FACE('',(#3541),#2117,.F.) ;
#32021=ADVANCED_FACE('',(#3542),#30509,.F.) ;
#32022=ADVANCED_FACE('',(#3543,#1151,#1152,#1153),#2118,.T.) ;
#32023=ADVANCED_FACE('',(#3544),#396,.T.) ;
#32024=ADVANCED_FACE('',(#3545),#30510,.F.) ;
#32025=ADVANCED_FACE('',(#3546),#397,.F.) ;
#32026=ADVANCED_FACE('',(#3547),#2119,.F.) ;
#32027=ADVANCED_FACE('',(#3548),#30511,.F.) ;
#32028=ADVANCED_FACE('',(#3549,#1154,#1155,#1156),#2120,.T.) ;
#32029=ADVANCED_FACE('',(#3550),#398,.T.) ;
#32030=ADVANCED_FACE('',(#3551),#30512,.F.) ;
#32031=ADVANCED_FACE('',(#3552),#399,.F.) ;
#32032=ADVANCED_FACE('',(#3553),#2121,.F.) ;
#32033=ADVANCED_FACE('',(#3554),#30513,.F.) ;
#32034=ADVANCED_FACE('',(#3555,#1157,#1158,#1159),#2122,.T.) ;
#32035=ADVANCED_FACE('',(#3556),#400,.T.) ;
#32036=ADVANCED_FACE('',(#3557),#30514,.F.) ;
#32037=ADVANCED_FACE('',(#3558),#401,.F.) ;
#32038=ADVANCED_FACE('',(#3559),#2123,.F.) ;
#32039=ADVANCED_FACE('',(#3560),#30515,.F.) ;
#32040=ADVANCED_FACE('',(#3561,#1160,#1161,#1162),#2124,.T.) ;
#32041=ADVANCED_FACE('',(#3562),#402,.T.) ;
#32042=ADVANCED_FACE('',(#3563),#30516,.F.) ;
#32043=ADVANCED_FACE('',(#3564),#403,.F.) ;
#32044=ADVANCED_FACE('',(#3565),#2125,.F.) ;
#32045=ADVANCED_FACE('',(#3566),#30517,.F.) ;
#32046=ADVANCED_FACE('',(#3567,#1163,#1164,#1165),#2126,.T.) ;
#32047=ADVANCED_FACE('',(#3568),#404,.T.) ;
#32048=ADVANCED_FACE('',(#3569),#30518,.F.) ;
#32049=ADVANCED_FACE('',(#3570),#405,.F.) ;
#32050=ADVANCED_FACE('',(#3571),#2127,.F.) ;
#32051=ADVANCED_FACE('',(#3572),#30519,.F.) ;
#32052=ADVANCED_FACE('',(#3573,#1166,#1167,#1168),#2128,.T.) ;
#32053=ADVANCED_FACE('',(#3574),#406,.T.) ;
#32054=ADVANCED_FACE('',(#3575),#30520,.F.) ;
#32055=ADVANCED_FACE('',(#3576),#407,.F.) ;
#32056=ADVANCED_FACE('',(#3577),#2129,.F.) ;
#32057=ADVANCED_FACE('',(#3578),#30521,.F.) ;
#32058=ADVANCED_FACE('',(#3579),#408,.T.) ;
#32059=ADVANCED_FACE('',(#3580),#30522,.F.) ;
#32060=ADVANCED_FACE('',(#3581),#409,.F.) ;
#32061=ADVANCED_FACE('',(#3582),#2130,.F.) ;
#32062=ADVANCED_FACE('',(#3583),#2131,.T.) ;
#32063=ADVANCED_FACE('',(#3584),#30523,.F.) ;
#32064=ADVANCED_FACE('',(#3585),#2132,.F.) ;
#32065=ADVANCED_FACE('',(#3586),#30524,.F.) ;
#32066=ADVANCED_FACE('',(#3587),#2133,.F.) ;
#32067=ADVANCED_FACE('',(#3588),#30525,.F.) ;
#32068=ADVANCED_FACE('',(#3589),#30526,.F.) ;
#32069=ADVANCED_FACE('',(#3590),#2134,.F.) ;
#32070=ADVANCED_FACE('',(#3591),#30527,.F.) ;
#32071=ADVANCED_FACE('',(#3592),#2135,.F.) ;
#32072=ADVANCED_FACE('',(#3593),#30528,.F.) ;
#32073=ADVANCED_FACE('',(#3594),#30529,.F.) ;
#32074=ADVANCED_FACE('',(#3595),#2136,.F.) ;
#32075=ADVANCED_FACE('',(#3596),#30530,.F.) ;
#32076=ADVANCED_FACE('',(#3597),#2137,.F.) ;
#32077=ADVANCED_FACE('',(#3598),#30531,.F.) ;
#32078=ADVANCED_FACE('',(#3599),#30532,.F.) ;
#32079=ADVANCED_FACE('',(#3600),#2138,.F.) ;
#32080=ADVANCED_FACE('',(#3601),#30533,.F.) ;
#32081=ADVANCED_FACE('',(#3602),#2139,.F.) ;
#32082=ADVANCED_FACE('',(#3603),#30534,.F.) ;
#32083=ADVANCED_FACE('',(#3604),#30535,.F.) ;
#32084=ADVANCED_FACE('',(#3605),#2140,.F.) ;
#32085=ADVANCED_FACE('',(#3606),#30536,.F.) ;
#32086=ADVANCED_FACE('',(#3607),#2141,.F.) ;
#32087=ADVANCED_FACE('',(#3608),#30537,.F.) ;
#32088=ADVANCED_FACE('',(#3609),#30538,.F.) ;
#32089=ADVANCED_FACE('',(#3610),#2142,.F.) ;
#32090=ADVANCED_FACE('',(#3611),#30539,.F.) ;
#32091=ADVANCED_FACE('',(#3612),#2143,.F.) ;
#32092=ADVANCED_FACE('',(#3613),#30540,.F.) ;
#32093=ADVANCED_FACE('',(#3614),#30541,.F.) ;
#32094=ADVANCED_FACE('',(#3615),#2144,.F.) ;
#32095=ADVANCED_FACE('',(#3616),#30542,.F.) ;
#32096=ADVANCED_FACE('',(#3617),#2145,.F.) ;
#32097=ADVANCED_FACE('',(#3618),#30543,.F.) ;
#32098=ADVANCED_FACE('',(#3619),#30544,.F.) ;
#32099=ADVANCED_FACE('',(#3620),#2146,.F.) ;
#32100=ADVANCED_FACE('',(#3621),#30545,.F.) ;
#32101=ADVANCED_FACE('',(#3622),#2147,.F.) ;
#32102=ADVANCED_FACE('',(#3623),#30546,.F.) ;
#32641=CLOSED_SHELL('',(#31259,#31260,#31261,#31262,#31263,#31264,#31265,
#31266,#31267,#31268,#31269,#31270,#31271,#31272,#31273,#31274,#31275,#31276,
#31277,#31278,#31279,#31280,#31281,#31282,#31283,#31284,#31285,#31286,#31287,
#31288,#31289,#31290,#31291,#31292,#31293,#31294,#31295,#31296,#31297,#31298,
#31299,#31300,#31301,#31302,#31303,#31304,#31305,#31306,#31307,#31308,#31309,
#31310,#31311,#31312,#31313,#31314,#31315,#31316,#31317,#31318,#31319,#31320,
#31321,#31322,#31323,#31324,#31325,#31326,#31327,#31328,#31329,#31330,#31331,
#31332,#31333,#31334,#31335,#31336,#31337,#31338,#31339,#31340,#31341,#31342,
#31343,#31344,#31345,#31346,#31347,#31348,#31349,#31350,#31351,#31352,#31353,
#31354,#31355,#31356,#31357,#31358,#31359,#31360,#31361,#31362,#31363,#31364,
#31365,#31366,#31367,#31368,#31369,#31370,#31371,#31372,#31373,#31374,#31375,
#31376,#31377,#31378,#31379,#31380,#31381,#31382,#31383,#31384,#31385,#31386,
#31387,#31388,#31389,#31390,#31391,#31392,#31393,#31394,#31395,#31396,#31397,
#31398,#31399,#31400,#31401,#31402,#31403,#31404,#31405,#31406,#31407,#31408,
#31409,#31410,#31411,#31412,#31413,#31414,#31415,#31416,#31417,#31418,#31419,
#31420,#31421,#31422,#31423,#31424,#31425,#31426,#31427,#31428,#31429,#31430,
#31431,#31432,#31433,#31434,#31435,#31436,#31437,#31438,#31439,#31440,#31441,
#31442,#31443,#31444,#31445,#31446,#31447,#31448,#31449,#31450,#31451,#31452,
#31453,#31454,#31455,#31456,#31457,#31458,#31459,#31460,#31461,#31462,#31463,
#31464,#31465,#31466,#31467,#31468,#31469,#31470,#31471,#31472,#31473,#31474,
#31475,#31476,#31477,#31478,#31479,#31480,#31481,#31482,#31483,#31484,#31485,
#31486,#31487,#31488,#31489,#31490,#31491,#31492,#31493,#31494,#31495,#31496,
#31497,#31498,#31499,#31500,#31501,#31502,#31503,#31504,#31505,#31506,#31507,
#31508,#31509,#31510,#31511,#31512,#31513,#31514,#31515,#31516,#31517,#31518,
#31519,#31520,#31521,#31522,#31523,#31524,#31525,#31526,#31527,#31528,#31529,
#31530,#31531,#31532,#31533,#31534,#31535,#31536,#31537,#31538,#31539,#31540,
#31541,#31542,#31543,#31544,#31545,#31546,#31547,#31548,#31549,#31550,#31551,
#31552,#31553,#31554,#31555,#31556,#31557,#31558,#31559,#31560,#31561,#31562,
#31563,#31564,#31565,#31566,#31567,#31568,#31569,#31570,#31571,#31572,#31573,
#31574,#31575,#31576,#31577,#31578,#31579,#31580,#31581,#31582,#31583,#31584,
#31585,#31586,#31587,#31588,#31589,#31590,#31591,#31592,#31593,#31594,#31595,
#31596,#31597,#31598,#31599,#31600,#31601,#31602,#31603,#31604,#31605,#31606,
#31607,#31608,#31609,#31610,#31611,#31612,#31613,#31614,#31615,#31616,#31617,
#31618,#31619,#31620,#31621,#31622,#31623,#31624,#31625,#31626,#31627,#31628,
#31629,#31630,#31631,#31632,#31633,#31634,#31635,#31636,#31637,#31638,#31639,
#31640,#31641,#31642,#31643,#31644,#31645,#31646,#31647,#31648,#31649,#31650,
#31651,#31652,#31653,#31654,#31655,#31656,#31657,#31658,#31659,#31660,#31661,
#31662,#31663,#31664,#31665,#31666,#31667,#31668,#31669,#31670,#31671,#31672,
#31673,#31674,#31675,#31676,#31677,#31678,#31679,#31680,#31681,#31682,#31683,
#31684,#31685,#31686,#31687,#31688,#31689,#31690,#31691,#31692,#31693,#31694,
#31695,#31696,#31697,#31698,#31699,#31700,#31701,#31702,#31703,#31704,#31705,
#31706,#31707,#31708,#31709,#31710,#31711,#31712,#31713,#31714,#31715,#31716,
#31717,#31718,#31719,#31720,#31721,#31722,#31723,#31724,#31725,#31726,#31727,
#31728,#31729,#31730,#31731,#31732,#31733,#31734,#31735,#31736,#31737,#31738,
#31739,#31740,#31741,#31742,#31743,#31744,#31745,#31746,#31747,#31748,#31749,
#31750,#31751,#31752,#31753,#31754,#31755,#31756,#31757,#31758,#31759,#31760,
#31761,#31762,#31763,#31764,#31765,#31766,#31767,#31768,#31769,#31770,#31771,
#31772,#31773,#31774,#31775,#31776,#31777,#31778,#31779,#31780,#31781,#31782,
#31783,#31784,#31785,#31786,#31787,#31788,#31789,#31790,#31791,#31792,#31793,
#31794,#31795,#31796,#31797,#31798,#31799,#31800,#31801,#31802,#31803,#31804,
#31805,#31806,#31807,#31808,#31809,#31810,#31811,#31812,#31813,#31814,#31815,
#31816,#31817,#31818,#31819,#31820,#31821,#31822,#31823,#31824,#31825,#31826,
#31827,#31828,#31829,#31830,#31831,#31832,#31833,#31834,#31835,#31836,#31837,
#31838,#31839,#31840,#31841,#31842,#31843,#31844,#31845,#31846,#31847,#31848,
#31849,#31850,#31851,#31852,#31853,#31854,#31855,#31856,#31857,#31858,#31859,
#31860,#31861,#31862,#31863,#31864,#31865,#31866,#31867,#31868,#31869,#31870,
#31871,#31872,#31873,#31874,#31875,#31876,#31877,#31878,#31879,#31880,#31881,
#31882,#31883,#31884,#31885,#31886,#31887,#31888,#31889,#31890,#31891,#31892,
#31893,#31894,#31895,#31896,#31897,#31898,#31899,#31900,#31901,#31902,#31903,
#31904,#31905,#31906,#31907,#31908,#31909,#31910,#31911,#31912,#31913,#31914,
#31915,#31916,#31917,#31918,#31919,#31920,#31921,#31922,#31923,#31924,#31925,
#31926,#31927,#31928,#31929,#31930,#31931,#31932,#31933,#31934,#31935,#31936,
#31937,#31938,#31939,#31940,#31941,#31942,#31943,#31944,#31945,#31946,#31947,
#31948,#31949,#31950,#31951,#31952,#31953,#31954,#31955,#31956,#31957,#31958,
#31959,#31960,#31961,#31962,#31963,#31964,#31965,#31966,#31967,#31968,#31969,
#31970,#31971,#31972,#31973,#31974,#31975,#31976,#31977,#31978,#31979,#31980,
#31981,#31982,#31983,#31984,#31985,#31986,#31987,#31988,#31989,#31990,#31991,
#31992,#31993,#31994,#31995,#31996,#31997,#31998,#31999,#32000,#32001,#32002,
#32003,#32004,#32005,#32006,#32007,#32008,#32009,#32010,#32011,#32012,#32013,
#32014,#32015,#32016,#32017,#32018,#32019,#32020,#32021,#32022,#32023,#32024,
#32025,#32026,#32027,#32028,#32029,#32030,#32031,#32032,#32033,#32034,#32035,
#32036,#32037,#32038,#32039,#32040,#32041,#32042,#32043,#32044,#32045,#32046,
#32047,#32048,#32049,#32050,#32051,#32052,#32053,#32054,#32055,#32056,#32057,
#32058,#32059,#32060,#32061,#32062,#32063,#32064,#32065,#32066,#32067,#32068,
#32069,#32070,#32071,#32072,#32073,#32074,#32075,#32076,#32077,#32078,#32079,
#32080,#32081,#32082,#32083,#32084,#32085,#32086,#32087,#32088,#32089,#32090,
#32091,#32092,#32093,#32094,#32095,#32096,#32097,#32098,#32099,#32100,#32101,
#32102)) ;
#33718=AXIS2_PLACEMENT_3D('',#69339,#39204,#39205) ;
#33719=AXIS2_PLACEMENT_3D('',#69340,#39206,#39207) ;
#33720=AXIS2_PLACEMENT_3D('',#69349,#39212,#39213) ;
#33721=AXIS2_PLACEMENT_3D('',#69355,#39217,#39218) ;
#33722=AXIS2_PLACEMENT_3D('',#69361,#39222,#39223) ;
#33723=AXIS2_PLACEMENT_3D('',#69363,#39225,#39226) ;
#33724=AXIS2_PLACEMENT_3D('',#69372,#39231,#39232) ;
#33725=AXIS2_PLACEMENT_3D('',#69378,#39236,#39237) ;
#33726=AXIS2_PLACEMENT_3D('',#69384,#39241,#39242) ;
#33727=AXIS2_PLACEMENT_3D('',#69386,#39244,#39245) ;
#33728=AXIS2_PLACEMENT_3D('',#69395,#39250,#39251) ;
#33729=AXIS2_PLACEMENT_3D('',#69401,#39255,#39256) ;
#33730=AXIS2_PLACEMENT_3D('',#69407,#39260,#39261) ;
#33731=AXIS2_PLACEMENT_3D('',#69409,#39263,#39264) ;
#33732=AXIS2_PLACEMENT_3D('',#69418,#39269,#39270) ;
#33733=AXIS2_PLACEMENT_3D('',#69424,#39274,#39275) ;
#33734=AXIS2_PLACEMENT_3D('',#69430,#39279,#39280) ;
#33735=AXIS2_PLACEMENT_3D('',#69432,#39282,#39283) ;
#33736=AXIS2_PLACEMENT_3D('',#69441,#39288,#39289) ;
#33737=AXIS2_PLACEMENT_3D('',#69447,#39293,#39294) ;
#33738=AXIS2_PLACEMENT_3D('',#69453,#39298,#39299) ;
#33739=AXIS2_PLACEMENT_3D('',#69455,#39301,#39302) ;
#33740=AXIS2_PLACEMENT_3D('',#69464,#39307,#39308) ;
#33741=AXIS2_PLACEMENT_3D('',#69470,#39312,#39313) ;
#33742=AXIS2_PLACEMENT_3D('',#69476,#39317,#39318) ;
#33743=AXIS2_PLACEMENT_3D('',#69478,#39320,#39321) ;
#33744=AXIS2_PLACEMENT_3D('',#69487,#39326,#39327) ;
#33745=AXIS2_PLACEMENT_3D('',#69493,#39331,#39332) ;
#33746=AXIS2_PLACEMENT_3D('',#69499,#39336,#39337) ;
#33747=AXIS2_PLACEMENT_3D('',#69501,#39339,#39340) ;
#33748=AXIS2_PLACEMENT_3D('',#69510,#39345,#39346) ;
#33749=AXIS2_PLACEMENT_3D('',#69516,#39350,#39351) ;
#33750=AXIS2_PLACEMENT_3D('',#69522,#39355,#39356) ;
#33751=AXIS2_PLACEMENT_3D('',#69524,#39358,#39359) ;
#33752=AXIS2_PLACEMENT_3D('',#69533,#39364,#39365) ;
#33753=AXIS2_PLACEMENT_3D('',#69539,#39369,#39370) ;
#33754=AXIS2_PLACEMENT_3D('',#69545,#39374,#39375) ;
#33755=AXIS2_PLACEMENT_3D('',#69547,#39377,#39378) ;
#33756=AXIS2_PLACEMENT_3D('',#69637,#39428,#39429) ;
#33757=AXIS2_PLACEMENT_3D('',#69639,#39430,#39431) ;
#33758=AXIS2_PLACEMENT_3D('',#69641,#39432,#39433) ;
#33759=AXIS2_PLACEMENT_3D('',#69642,#39434,#39435) ;
#33760=AXIS2_PLACEMENT_3D('',#69643,#39436,#39437) ;
#33761=AXIS2_PLACEMENT_3D('',#69645,#39438,#39439) ;
#33762=AXIS2_PLACEMENT_3D('',#69647,#39441,#39442) ;
#33763=AXIS2_PLACEMENT_3D('',#69660,#39448,#39449) ;
#33764=AXIS2_PLACEMENT_3D('',#69664,#39451,#39452) ;
#33765=AXIS2_PLACEMENT_3D('',#69668,#39454,#39455) ;
#33766=AXIS2_PLACEMENT_3D('',#69671,#39457,#39458) ;
#33767=AXIS2_PLACEMENT_3D('',#69672,#39459,#39460) ;
#33768=AXIS2_PLACEMENT_3D('',#69674,#39461,#39462) ;
#33769=AXIS2_PLACEMENT_3D('',#69676,#39463,#39464) ;
#33770=AXIS2_PLACEMENT_3D('',#69677,#39465,#39466) ;
#33771=AXIS2_PLACEMENT_3D('',#69678,#39467,#39468) ;
#33772=AXIS2_PLACEMENT_3D('',#69680,#39469,#39470) ;
#33773=AXIS2_PLACEMENT_3D('',#69682,#39472,#39473) ;
#33774=AXIS2_PLACEMENT_3D('',#69695,#39479,#39480) ;
#33775=AXIS2_PLACEMENT_3D('',#69699,#39482,#39483) ;
#33776=AXIS2_PLACEMENT_3D('',#69703,#39485,#39486) ;
#33777=AXIS2_PLACEMENT_3D('',#69706,#39488,#39489) ;
#33778=AXIS2_PLACEMENT_3D('',#69707,#39490,#39491) ;
#33779=AXIS2_PLACEMENT_3D('',#69709,#39492,#39493) ;
#33780=AXIS2_PLACEMENT_3D('',#69711,#39494,#39495) ;
#33781=AXIS2_PLACEMENT_3D('',#69712,#39496,#39497) ;
#33782=AXIS2_PLACEMENT_3D('',#69713,#39498,#39499) ;
#33783=AXIS2_PLACEMENT_3D('',#69715,#39500,#39501) ;
#33784=AXIS2_PLACEMENT_3D('',#69717,#39503,#39504) ;
#33785=AXIS2_PLACEMENT_3D('',#69730,#39510,#39511) ;
#33786=AXIS2_PLACEMENT_3D('',#69734,#39513,#39514) ;
#33787=AXIS2_PLACEMENT_3D('',#69738,#39516,#39517) ;
#33788=AXIS2_PLACEMENT_3D('',#69741,#39519,#39520) ;
#33789=AXIS2_PLACEMENT_3D('',#69742,#39521,#39522) ;
#33790=AXIS2_PLACEMENT_3D('',#69744,#39523,#39524) ;
#33791=AXIS2_PLACEMENT_3D('',#69746,#39525,#39526) ;
#33792=AXIS2_PLACEMENT_3D('',#69747,#39527,#39528) ;
#33793=AXIS2_PLACEMENT_3D('',#69748,#39529,#39530) ;
#33794=AXIS2_PLACEMENT_3D('',#69750,#39531,#39532) ;
#33795=AXIS2_PLACEMENT_3D('',#69752,#39534,#39535) ;
#33796=AXIS2_PLACEMENT_3D('',#69765,#39541,#39542) ;
#33797=AXIS2_PLACEMENT_3D('',#69769,#39544,#39545) ;
#33798=AXIS2_PLACEMENT_3D('',#69773,#39547,#39548) ;
#33799=AXIS2_PLACEMENT_3D('',#69776,#39550,#39551) ;
#33800=AXIS2_PLACEMENT_3D('',#69777,#39552,#39553) ;
#33801=AXIS2_PLACEMENT_3D('',#69779,#39554,#39555) ;
#33802=AXIS2_PLACEMENT_3D('',#69781,#39556,#39557) ;
#33803=AXIS2_PLACEMENT_3D('',#69782,#39558,#39559) ;
#33804=AXIS2_PLACEMENT_3D('',#69783,#39560,#39561) ;
#33805=AXIS2_PLACEMENT_3D('',#69785,#39562,#39563) ;
#33806=AXIS2_PLACEMENT_3D('',#69787,#39565,#39566) ;
#33807=AXIS2_PLACEMENT_3D('',#69800,#39572,#39573) ;
#33808=AXIS2_PLACEMENT_3D('',#69804,#39575,#39576) ;
#33809=AXIS2_PLACEMENT_3D('',#69808,#39578,#39579) ;
#33810=AXIS2_PLACEMENT_3D('',#69811,#39581,#39582) ;
#33811=AXIS2_PLACEMENT_3D('',#69812,#39583,#39584) ;
#33812=AXIS2_PLACEMENT_3D('',#69814,#39585,#39586) ;
#33813=AXIS2_PLACEMENT_3D('',#69816,#39587,#39588) ;
#33814=AXIS2_PLACEMENT_3D('',#69817,#39589,#39590) ;
#33815=AXIS2_PLACEMENT_3D('',#69818,#39591,#39592) ;
#33816=AXIS2_PLACEMENT_3D('',#69820,#39593,#39594) ;
#33817=AXIS2_PLACEMENT_3D('',#69822,#39596,#39597) ;
#33818=AXIS2_PLACEMENT_3D('',#69835,#39603,#39604) ;
#33819=AXIS2_PLACEMENT_3D('',#69839,#39606,#39607) ;
#33820=AXIS2_PLACEMENT_3D('',#69843,#39609,#39610) ;
#33821=AXIS2_PLACEMENT_3D('',#69846,#39612,#39613) ;
#33822=AXIS2_PLACEMENT_3D('',#69847,#39614,#39615) ;
#33823=AXIS2_PLACEMENT_3D('',#69849,#39616,#39617) ;
#33824=AXIS2_PLACEMENT_3D('',#69851,#39618,#39619) ;
#33825=AXIS2_PLACEMENT_3D('',#69852,#39620,#39621) ;
#33826=AXIS2_PLACEMENT_3D('',#69853,#39622,#39623) ;
#33827=AXIS2_PLACEMENT_3D('',#69855,#39624,#39625) ;
#33828=AXIS2_PLACEMENT_3D('',#69857,#39627,#39628) ;
#33829=AXIS2_PLACEMENT_3D('',#69870,#39634,#39635) ;
#33830=AXIS2_PLACEMENT_3D('',#69874,#39637,#39638) ;
#33831=AXIS2_PLACEMENT_3D('',#69878,#39640,#39641) ;
#33832=AXIS2_PLACEMENT_3D('',#69881,#39643,#39644) ;
#33833=AXIS2_PLACEMENT_3D('',#69882,#39645,#39646) ;
#33834=AXIS2_PLACEMENT_3D('',#69884,#39647,#39648) ;
#33835=AXIS2_PLACEMENT_3D('',#69886,#39649,#39650) ;
#33836=AXIS2_PLACEMENT_3D('',#69887,#39651,#39652) ;
#33837=AXIS2_PLACEMENT_3D('',#69888,#39653,#39654) ;
#33838=AXIS2_PLACEMENT_3D('',#69890,#39655,#39656) ;
#33839=AXIS2_PLACEMENT_3D('',#69892,#39658,#39659) ;
#33840=AXIS2_PLACEMENT_3D('',#69905,#39665,#39666) ;
#33841=AXIS2_PLACEMENT_3D('',#69909,#39668,#39669) ;
#33842=AXIS2_PLACEMENT_3D('',#69913,#39671,#39672) ;
#33843=AXIS2_PLACEMENT_3D('',#69916,#39674,#39675) ;
#33844=AXIS2_PLACEMENT_3D('',#69917,#39676,#39677) ;
#33845=AXIS2_PLACEMENT_3D('',#69919,#39678,#39679) ;
#33846=AXIS2_PLACEMENT_3D('',#69921,#39680,#39681) ;
#33847=AXIS2_PLACEMENT_3D('',#69922,#39682,#39683) ;
#33848=AXIS2_PLACEMENT_3D('',#69923,#39684,#39685) ;
#33849=AXIS2_PLACEMENT_3D('',#69936,#39691,#39692) ;
#33850=AXIS2_PLACEMENT_3D('',#69940,#39694,#39695) ;
#33851=AXIS2_PLACEMENT_3D('',#69944,#39697,#39698) ;
#33852=AXIS2_PLACEMENT_3D('',#69947,#39700,#39701) ;
#33853=AXIS2_PLACEMENT_3D('',#69948,#39702,#39703) ;
#33854=AXIS2_PLACEMENT_3D('',#69950,#39704,#39705) ;
#33855=AXIS2_PLACEMENT_3D('',#69952,#39707,#39708) ;
#33856=AXIS2_PLACEMENT_3D('',#69954,#39709,#39710) ;
#33857=AXIS2_PLACEMENT_3D('',#69955,#39711,#39712) ;
#33858=AXIS2_PLACEMENT_3D('',#69957,#39713,#39714) ;
#33859=AXIS2_PLACEMENT_3D('',#69958,#39715,#39716) ;
#33860=AXIS2_PLACEMENT_3D('',#69960,#39717,#39718) ;
#33861=AXIS2_PLACEMENT_3D('',#69961,#39719,#39720) ;
#33862=AXIS2_PLACEMENT_3D('',#69963,#39721,#39722) ;
#33863=AXIS2_PLACEMENT_3D('',#69964,#39723,#39724) ;
#33864=AXIS2_PLACEMENT_3D('',#69966,#39725,#39726) ;
#33865=AXIS2_PLACEMENT_3D('',#69967,#39727,#39728) ;
#33866=AXIS2_PLACEMENT_3D('',#69969,#39729,#39730) ;
#33867=AXIS2_PLACEMENT_3D('',#69970,#39731,#39732) ;
#33868=AXIS2_PLACEMENT_3D('',#69972,#39733,#39734) ;
#33869=AXIS2_PLACEMENT_3D('',#69973,#39735,#39736) ;
#33870=AXIS2_PLACEMENT_3D('',#69975,#39737,#39738) ;
#33871=AXIS2_PLACEMENT_3D('',#69976,#39739,#39740) ;
#33872=AXIS2_PLACEMENT_3D('',#69978,#39741,#39742) ;
#33873=AXIS2_PLACEMENT_3D('',#69981,#39744,#39745) ;
#33874=AXIS2_PLACEMENT_3D('',#69982,#39746,#39747) ;
#33875=AXIS2_PLACEMENT_3D('',#69984,#39748,#39749) ;
#33876=AXIS2_PLACEMENT_3D('',#69985,#39750,#39751) ;
#33877=AXIS2_PLACEMENT_3D('',#69986,#39752,#39753) ;
#33878=AXIS2_PLACEMENT_3D('',#69988,#39754,#39755) ;
#33879=AXIS2_PLACEMENT_3D('',#69990,#39757,#39758) ;
#33880=AXIS2_PLACEMENT_3D('',#69992,#39759,#39760) ;
#33881=AXIS2_PLACEMENT_3D('',#69993,#39761,#39762) ;
#33882=AXIS2_PLACEMENT_3D('',#69994,#39763,#39764) ;
#33883=AXIS2_PLACEMENT_3D('',#69996,#39765,#39766) ;
#33884=AXIS2_PLACEMENT_3D('',#69998,#39768,#39769) ;
#33885=AXIS2_PLACEMENT_3D('',#70000,#39770,#39771) ;
#33886=AXIS2_PLACEMENT_3D('',#70001,#39772,#39773) ;
#33887=AXIS2_PLACEMENT_3D('',#70002,#39774,#39775) ;
#33888=AXIS2_PLACEMENT_3D('',#70004,#39776,#39777) ;
#33889=AXIS2_PLACEMENT_3D('',#70006,#39779,#39780) ;
#33890=AXIS2_PLACEMENT_3D('',#70007,#39781,#39782) ;
#33891=AXIS2_PLACEMENT_3D('',#70008,#39783,#39784) ;
#33892=AXIS2_PLACEMENT_3D('',#70012,#39786,#39787) ;
#33893=AXIS2_PLACEMENT_3D('',#70014,#39789,#39790) ;
#33894=AXIS2_PLACEMENT_3D('',#70018,#39792,#39793) ;
#33895=AXIS2_PLACEMENT_3D('',#70029,#39799,#39800) ;
#33896=AXIS2_PLACEMENT_3D('',#70030,#39801,#39802) ;
#33897=AXIS2_PLACEMENT_3D('',#70033,#39804,#39805) ;
#33898=AXIS2_PLACEMENT_3D('',#70034,#39806,#39807) ;
#33899=AXIS2_PLACEMENT_3D('',#70038,#39810,#39811) ;
#33900=AXIS2_PLACEMENT_3D('',#70040,#39812,#39813) ;
#33901=AXIS2_PLACEMENT_3D('',#70043,#39815,#39816) ;
#33902=AXIS2_PLACEMENT_3D('',#70044,#39817,#39818) ;
#33903=AXIS2_PLACEMENT_3D('',#70046,#39819,#39820) ;
#33904=AXIS2_PLACEMENT_3D('',#70047,#39821,#39822) ;
#33905=AXIS2_PLACEMENT_3D('',#70048,#39823,#39824) ;
#33906=AXIS2_PLACEMENT_3D('',#70050,#39825,#39826) ;
#33907=AXIS2_PLACEMENT_3D('',#70052,#39828,#39829) ;
#33908=AXIS2_PLACEMENT_3D('',#70054,#39830,#39831) ;
#33909=AXIS2_PLACEMENT_3D('',#70055,#39832,#39833) ;
#33910=AXIS2_PLACEMENT_3D('',#70056,#39834,#39835) ;
#33911=AXIS2_PLACEMENT_3D('',#70058,#39836,#39837) ;
#33912=AXIS2_PLACEMENT_3D('',#70060,#39839,#39840) ;
#33913=AXIS2_PLACEMENT_3D('',#70062,#39841,#39842) ;
#33914=AXIS2_PLACEMENT_3D('',#70063,#39843,#39844) ;
#33915=AXIS2_PLACEMENT_3D('',#70064,#39845,#39846) ;
#33916=AXIS2_PLACEMENT_3D('',#70066,#39847,#39848) ;
#33917=AXIS2_PLACEMENT_3D('',#70068,#39850,#39851) ;
#33918=AXIS2_PLACEMENT_3D('',#70069,#39852,#39853) ;
#33919=AXIS2_PLACEMENT_3D('',#70070,#39854,#39855) ;
#33920=AXIS2_PLACEMENT_3D('',#70074,#39857,#39858) ;
#33921=AXIS2_PLACEMENT_3D('',#70076,#39860,#39861) ;
#33922=AXIS2_PLACEMENT_3D('',#70080,#39863,#39864) ;
#33923=AXIS2_PLACEMENT_3D('',#70091,#39870,#39871) ;
#33924=AXIS2_PLACEMENT_3D('',#70092,#39872,#39873) ;
#33925=AXIS2_PLACEMENT_3D('',#70095,#39875,#39876) ;
#33926=AXIS2_PLACEMENT_3D('',#70096,#39877,#39878) ;
#33927=AXIS2_PLACEMENT_3D('',#70100,#39881,#39882) ;
#33928=AXIS2_PLACEMENT_3D('',#70102,#39883,#39884) ;
#33929=AXIS2_PLACEMENT_3D('',#70105,#39886,#39887) ;
#33930=AXIS2_PLACEMENT_3D('',#70106,#39888,#39889) ;
#33931=AXIS2_PLACEMENT_3D('',#70108,#39890,#39891) ;
#33932=AXIS2_PLACEMENT_3D('',#70109,#39892,#39893) ;
#33933=AXIS2_PLACEMENT_3D('',#70110,#39894,#39895) ;
#33934=AXIS2_PLACEMENT_3D('',#70112,#39896,#39897) ;
#33935=AXIS2_PLACEMENT_3D('',#70114,#39899,#39900) ;
#33936=AXIS2_PLACEMENT_3D('',#70116,#39901,#39902) ;
#33937=AXIS2_PLACEMENT_3D('',#70117,#39903,#39904) ;
#33938=AXIS2_PLACEMENT_3D('',#70118,#39905,#39906) ;
#33939=AXIS2_PLACEMENT_3D('',#70120,#39907,#39908) ;
#33940=AXIS2_PLACEMENT_3D('',#70122,#39910,#39911) ;
#33941=AXIS2_PLACEMENT_3D('',#70124,#39912,#39913) ;
#33942=AXIS2_PLACEMENT_3D('',#70125,#39914,#39915) ;
#33943=AXIS2_PLACEMENT_3D('',#70126,#39916,#39917) ;
#33944=AXIS2_PLACEMENT_3D('',#70128,#39918,#39919) ;
#33945=AXIS2_PLACEMENT_3D('',#70130,#39921,#39922) ;
#33946=AXIS2_PLACEMENT_3D('',#70131,#39923,#39924) ;
#33947=AXIS2_PLACEMENT_3D('',#70132,#39925,#39926) ;
#33948=AXIS2_PLACEMENT_3D('',#70136,#39928,#39929) ;
#33949=AXIS2_PLACEMENT_3D('',#70138,#39931,#39932) ;
#33950=AXIS2_PLACEMENT_3D('',#70142,#39934,#39935) ;
#33951=AXIS2_PLACEMENT_3D('',#70153,#39941,#39942) ;
#33952=AXIS2_PLACEMENT_3D('',#70154,#39943,#39944) ;
#33953=AXIS2_PLACEMENT_3D('',#70157,#39946,#39947) ;
#33954=AXIS2_PLACEMENT_3D('',#70158,#39948,#39949) ;
#33955=AXIS2_PLACEMENT_3D('',#70162,#39952,#39953) ;
#33956=AXIS2_PLACEMENT_3D('',#70164,#39954,#39955) ;
#33957=AXIS2_PLACEMENT_3D('',#70167,#39957,#39958) ;
#33958=AXIS2_PLACEMENT_3D('',#70168,#39959,#39960) ;
#33959=AXIS2_PLACEMENT_3D('',#70170,#39961,#39962) ;
#33960=AXIS2_PLACEMENT_3D('',#70171,#39963,#39964) ;
#33961=AXIS2_PLACEMENT_3D('',#70172,#39965,#39966) ;
#33962=AXIS2_PLACEMENT_3D('',#70174,#39967,#39968) ;
#33963=AXIS2_PLACEMENT_3D('',#70176,#39970,#39971) ;
#33964=AXIS2_PLACEMENT_3D('',#70178,#39972,#39973) ;
#33965=AXIS2_PLACEMENT_3D('',#70179,#39974,#39975) ;
#33966=AXIS2_PLACEMENT_3D('',#70180,#39976,#39977) ;
#33967=AXIS2_PLACEMENT_3D('',#70182,#39978,#39979) ;
#33968=AXIS2_PLACEMENT_3D('',#70184,#39981,#39982) ;
#33969=AXIS2_PLACEMENT_3D('',#70186,#39983,#39984) ;
#33970=AXIS2_PLACEMENT_3D('',#70187,#39985,#39986) ;
#33971=AXIS2_PLACEMENT_3D('',#70188,#39987,#39988) ;
#33972=AXIS2_PLACEMENT_3D('',#70190,#39989,#39990) ;
#33973=AXIS2_PLACEMENT_3D('',#70192,#39992,#39993) ;
#33974=AXIS2_PLACEMENT_3D('',#70193,#39994,#39995) ;
#33975=AXIS2_PLACEMENT_3D('',#70194,#39996,#39997) ;
#33976=AXIS2_PLACEMENT_3D('',#70198,#39999,#40000) ;
#33977=AXIS2_PLACEMENT_3D('',#70200,#40002,#40003) ;
#33978=AXIS2_PLACEMENT_3D('',#70204,#40005,#40006) ;
#33979=AXIS2_PLACEMENT_3D('',#70215,#40012,#40013) ;
#33980=AXIS2_PLACEMENT_3D('',#70216,#40014,#40015) ;
#33981=AXIS2_PLACEMENT_3D('',#70219,#40017,#40018) ;
#33982=AXIS2_PLACEMENT_3D('',#70220,#40019,#40020) ;
#33983=AXIS2_PLACEMENT_3D('',#70224,#40023,#40024) ;
#33984=AXIS2_PLACEMENT_3D('',#70226,#40025,#40026) ;
#33985=AXIS2_PLACEMENT_3D('',#70229,#40028,#40029) ;
#33986=AXIS2_PLACEMENT_3D('',#70230,#40030,#40031) ;
#33987=AXIS2_PLACEMENT_3D('',#70232,#40032,#40033) ;
#33988=AXIS2_PLACEMENT_3D('',#70233,#40034,#40035) ;
#33989=AXIS2_PLACEMENT_3D('',#70234,#40036,#40037) ;
#33990=AXIS2_PLACEMENT_3D('',#70236,#40038,#40039) ;
#33991=AXIS2_PLACEMENT_3D('',#70238,#40041,#40042) ;
#33992=AXIS2_PLACEMENT_3D('',#70240,#40043,#40044) ;
#33993=AXIS2_PLACEMENT_3D('',#70241,#40045,#40046) ;
#33994=AXIS2_PLACEMENT_3D('',#70242,#40047,#40048) ;
#33995=AXIS2_PLACEMENT_3D('',#70244,#40049,#40050) ;
#33996=AXIS2_PLACEMENT_3D('',#70246,#40052,#40053) ;
#33997=AXIS2_PLACEMENT_3D('',#70248,#40054,#40055) ;
#33998=AXIS2_PLACEMENT_3D('',#70249,#40056,#40057) ;
#33999=AXIS2_PLACEMENT_3D('',#70250,#40058,#40059) ;
#34000=AXIS2_PLACEMENT_3D('',#70252,#40060,#40061) ;
#34001=AXIS2_PLACEMENT_3D('',#70254,#40063,#40064) ;
#34002=AXIS2_PLACEMENT_3D('',#70255,#40065,#40066) ;
#34003=AXIS2_PLACEMENT_3D('',#70256,#40067,#40068) ;
#34004=AXIS2_PLACEMENT_3D('',#70260,#40070,#40071) ;
#34005=AXIS2_PLACEMENT_3D('',#70262,#40073,#40074) ;
#34006=AXIS2_PLACEMENT_3D('',#70266,#40076,#40077) ;
#34007=AXIS2_PLACEMENT_3D('',#70277,#40083,#40084) ;
#34008=AXIS2_PLACEMENT_3D('',#70278,#40085,#40086) ;
#34009=AXIS2_PLACEMENT_3D('',#70281,#40088,#40089) ;
#34010=AXIS2_PLACEMENT_3D('',#70282,#40090,#40091) ;
#34011=AXIS2_PLACEMENT_3D('',#70286,#40094,#40095) ;
#34012=AXIS2_PLACEMENT_3D('',#70288,#40096,#40097) ;
#34013=AXIS2_PLACEMENT_3D('',#70291,#40099,#40100) ;
#34014=AXIS2_PLACEMENT_3D('',#70292,#40101,#40102) ;
#34015=AXIS2_PLACEMENT_3D('',#70294,#40103,#40104) ;
#34016=AXIS2_PLACEMENT_3D('',#70295,#40105,#40106) ;
#34017=AXIS2_PLACEMENT_3D('',#70296,#40107,#40108) ;
#34018=AXIS2_PLACEMENT_3D('',#70298,#40109,#40110) ;
#34019=AXIS2_PLACEMENT_3D('',#70300,#40112,#40113) ;
#34020=AXIS2_PLACEMENT_3D('',#70302,#40114,#40115) ;
#34021=AXIS2_PLACEMENT_3D('',#70303,#40116,#40117) ;
#34022=AXIS2_PLACEMENT_3D('',#70304,#40118,#40119) ;
#34023=AXIS2_PLACEMENT_3D('',#70306,#40120,#40121) ;
#34024=AXIS2_PLACEMENT_3D('',#70308,#40123,#40124) ;
#34025=AXIS2_PLACEMENT_3D('',#70310,#40125,#40126) ;
#34026=AXIS2_PLACEMENT_3D('',#70311,#40127,#40128) ;
#34027=AXIS2_PLACEMENT_3D('',#70312,#40129,#40130) ;
#34028=AXIS2_PLACEMENT_3D('',#70314,#40131,#40132) ;
#34029=AXIS2_PLACEMENT_3D('',#70316,#40134,#40135) ;
#34030=AXIS2_PLACEMENT_3D('',#70317,#40136,#40137) ;
#34031=AXIS2_PLACEMENT_3D('',#70318,#40138,#40139) ;
#34032=AXIS2_PLACEMENT_3D('',#70322,#40141,#40142) ;
#34033=AXIS2_PLACEMENT_3D('',#70324,#40144,#40145) ;
#34034=AXIS2_PLACEMENT_3D('',#70328,#40147,#40148) ;
#34035=AXIS2_PLACEMENT_3D('',#70339,#40154,#40155) ;
#34036=AXIS2_PLACEMENT_3D('',#70340,#40156,#40157) ;
#34037=AXIS2_PLACEMENT_3D('',#70343,#40159,#40160) ;
#34038=AXIS2_PLACEMENT_3D('',#70344,#40161,#40162) ;
#34039=AXIS2_PLACEMENT_3D('',#70348,#40165,#40166) ;
#34040=AXIS2_PLACEMENT_3D('',#70350,#40167,#40168) ;
#34041=AXIS2_PLACEMENT_3D('',#70353,#40170,#40171) ;
#34042=AXIS2_PLACEMENT_3D('',#70354,#40172,#40173) ;
#34043=AXIS2_PLACEMENT_3D('',#70356,#40174,#40175) ;
#34044=AXIS2_PLACEMENT_3D('',#70357,#40176,#40177) ;
#34045=AXIS2_PLACEMENT_3D('',#70358,#40178,#40179) ;
#34046=AXIS2_PLACEMENT_3D('',#70360,#40180,#40181) ;
#34047=AXIS2_PLACEMENT_3D('',#70362,#40183,#40184) ;
#34048=AXIS2_PLACEMENT_3D('',#70364,#40185,#40186) ;
#34049=AXIS2_PLACEMENT_3D('',#70365,#40187,#40188) ;
#34050=AXIS2_PLACEMENT_3D('',#70366,#40189,#40190) ;
#34051=AXIS2_PLACEMENT_3D('',#70368,#40191,#40192) ;
#34052=AXIS2_PLACEMENT_3D('',#70370,#40194,#40195) ;
#34053=AXIS2_PLACEMENT_3D('',#70372,#40196,#40197) ;
#34054=AXIS2_PLACEMENT_3D('',#70373,#40198,#40199) ;
#34055=AXIS2_PLACEMENT_3D('',#70374,#40200,#40201) ;
#34056=AXIS2_PLACEMENT_3D('',#70376,#40202,#40203) ;
#34057=AXIS2_PLACEMENT_3D('',#70378,#40205,#40206) ;
#34058=AXIS2_PLACEMENT_3D('',#70379,#40207,#40208) ;
#34059=AXIS2_PLACEMENT_3D('',#70380,#40209,#40210) ;
#34060=AXIS2_PLACEMENT_3D('',#70384,#40212,#40213) ;
#34061=AXIS2_PLACEMENT_3D('',#70386,#40215,#40216) ;
#34062=AXIS2_PLACEMENT_3D('',#70390,#40218,#40219) ;
#34063=AXIS2_PLACEMENT_3D('',#70401,#40225,#40226) ;
#34064=AXIS2_PLACEMENT_3D('',#70402,#40227,#40228) ;
#34065=AXIS2_PLACEMENT_3D('',#70405,#40230,#40231) ;
#34066=AXIS2_PLACEMENT_3D('',#70406,#40232,#40233) ;
#34067=AXIS2_PLACEMENT_3D('',#70410,#40236,#40237) ;
#34068=AXIS2_PLACEMENT_3D('',#70412,#40238,#40239) ;
#34069=AXIS2_PLACEMENT_3D('',#70415,#40241,#40242) ;
#34070=AXIS2_PLACEMENT_3D('',#70416,#40243,#40244) ;
#34071=AXIS2_PLACEMENT_3D('',#70418,#40245,#40246) ;
#34072=AXIS2_PLACEMENT_3D('',#70419,#40247,#40248) ;
#34073=AXIS2_PLACEMENT_3D('',#70420,#40249,#40250) ;
#34074=AXIS2_PLACEMENT_3D('',#70422,#40251,#40252) ;
#34075=AXIS2_PLACEMENT_3D('',#70424,#40254,#40255) ;
#34076=AXIS2_PLACEMENT_3D('',#70426,#40256,#40257) ;
#34077=AXIS2_PLACEMENT_3D('',#70427,#40258,#40259) ;
#34078=AXIS2_PLACEMENT_3D('',#70428,#40260,#40261) ;
#34079=AXIS2_PLACEMENT_3D('',#70430,#40262,#40263) ;
#34080=AXIS2_PLACEMENT_3D('',#70432,#40265,#40266) ;
#34081=AXIS2_PLACEMENT_3D('',#70434,#40267,#40268) ;
#34082=AXIS2_PLACEMENT_3D('',#70435,#40269,#40270) ;
#34083=AXIS2_PLACEMENT_3D('',#70436,#40271,#40272) ;
#34084=AXIS2_PLACEMENT_3D('',#70438,#40273,#40274) ;
#34085=AXIS2_PLACEMENT_3D('',#70440,#40276,#40277) ;
#34086=AXIS2_PLACEMENT_3D('',#70441,#40278,#40279) ;
#34087=AXIS2_PLACEMENT_3D('',#70442,#40280,#40281) ;
#34088=AXIS2_PLACEMENT_3D('',#70446,#40283,#40284) ;
#34089=AXIS2_PLACEMENT_3D('',#70448,#40286,#40287) ;
#34090=AXIS2_PLACEMENT_3D('',#70452,#40289,#40290) ;
#34091=AXIS2_PLACEMENT_3D('',#70463,#40296,#40297) ;
#34092=AXIS2_PLACEMENT_3D('',#70464,#40298,#40299) ;
#34093=AXIS2_PLACEMENT_3D('',#70467,#40301,#40302) ;
#34094=AXIS2_PLACEMENT_3D('',#70468,#40303,#40304) ;
#34095=AXIS2_PLACEMENT_3D('',#70472,#40307,#40308) ;
#34096=AXIS2_PLACEMENT_3D('',#70474,#40309,#40310) ;
#34097=AXIS2_PLACEMENT_3D('',#70477,#40312,#40313) ;
#34098=AXIS2_PLACEMENT_3D('',#70478,#40314,#40315) ;
#34099=AXIS2_PLACEMENT_3D('',#70480,#40316,#40317) ;
#34100=AXIS2_PLACEMENT_3D('',#70481,#40318,#40319) ;
#34101=AXIS2_PLACEMENT_3D('',#70482,#40320,#40321) ;
#34102=AXIS2_PLACEMENT_3D('',#70484,#40322,#40323) ;
#34103=AXIS2_PLACEMENT_3D('',#70486,#40325,#40326) ;
#34104=AXIS2_PLACEMENT_3D('',#70488,#40327,#40328) ;
#34105=AXIS2_PLACEMENT_3D('',#70489,#40329,#40330) ;
#34106=AXIS2_PLACEMENT_3D('',#70490,#40331,#40332) ;
#34107=AXIS2_PLACEMENT_3D('',#70492,#40333,#40334) ;
#34108=AXIS2_PLACEMENT_3D('',#70494,#40336,#40337) ;
#34109=AXIS2_PLACEMENT_3D('',#70496,#40338,#40339) ;
#34110=AXIS2_PLACEMENT_3D('',#70497,#40340,#40341) ;
#34111=AXIS2_PLACEMENT_3D('',#70498,#40342,#40343) ;
#34112=AXIS2_PLACEMENT_3D('',#70500,#40344,#40345) ;
#34113=AXIS2_PLACEMENT_3D('',#70502,#40347,#40348) ;
#34114=AXIS2_PLACEMENT_3D('',#70503,#40349,#40350) ;
#34115=AXIS2_PLACEMENT_3D('',#70504,#40351,#40352) ;
#34116=AXIS2_PLACEMENT_3D('',#70508,#40354,#40355) ;
#34117=AXIS2_PLACEMENT_3D('',#70510,#40357,#40358) ;
#34118=AXIS2_PLACEMENT_3D('',#70518,#40362,#40363) ;
#34119=AXIS2_PLACEMENT_3D('',#70522,#40365,#40366) ;
#34120=AXIS2_PLACEMENT_3D('',#70526,#40369,#40370) ;
#34121=AXIS2_PLACEMENT_3D('',#70529,#40372,#40373) ;
#34122=AXIS2_PLACEMENT_3D('',#70530,#40374,#40375) ;
#34123=AXIS2_PLACEMENT_3D('',#70534,#40378,#40379) ;
#34124=AXIS2_PLACEMENT_3D('',#70537,#40380,#40381) ;
#34125=AXIS2_PLACEMENT_3D('',#70541,#40383,#40384) ;
#34126=AXIS2_PLACEMENT_3D('',#70543,#40386,#40387) ;
#34127=AXIS2_PLACEMENT_3D('',#70546,#40388,#40389) ;
#34128=AXIS2_PLACEMENT_3D('',#70547,#40390,#40391) ;
#34129=AXIS2_PLACEMENT_3D('',#70548,#40392,#40393) ;
#34130=AXIS2_PLACEMENT_3D('',#70549,#40394,#40395) ;
#34131=AXIS2_PLACEMENT_3D('',#70552,#40396,#40397) ;
#34132=AXIS2_PLACEMENT_3D('',#70555,#40400,#40401) ;
#34133=AXIS2_PLACEMENT_3D('',#70558,#40402,#40403) ;
#34134=AXIS2_PLACEMENT_3D('',#70559,#40404,#40405) ;
#34135=AXIS2_PLACEMENT_3D('',#70560,#40406,#40407) ;
#34136=AXIS2_PLACEMENT_3D('',#70561,#40408,#40409) ;
#34137=AXIS2_PLACEMENT_3D('',#70564,#40410,#40411) ;
#34138=AXIS2_PLACEMENT_3D('',#70567,#40414,#40415) ;
#34139=AXIS2_PLACEMENT_3D('',#70570,#40416,#40417) ;
#34140=AXIS2_PLACEMENT_3D('',#70571,#40418,#40419) ;
#34141=AXIS2_PLACEMENT_3D('',#70572,#40420,#40421) ;
#34142=AXIS2_PLACEMENT_3D('',#70573,#40422,#40423) ;
#34143=AXIS2_PLACEMENT_3D('',#70576,#40424,#40425) ;
#34144=AXIS2_PLACEMENT_3D('',#70579,#40428,#40429) ;
#34145=AXIS2_PLACEMENT_3D('',#70580,#40430,#40431) ;
#34146=AXIS2_PLACEMENT_3D('',#70581,#40432,#40433) ;
#34147=AXIS2_PLACEMENT_3D('',#70582,#40434,#40435) ;
#34148=AXIS2_PLACEMENT_3D('',#70586,#40437,#40438) ;
#34149=AXIS2_PLACEMENT_3D('',#70588,#40440,#40441) ;
#34150=AXIS2_PLACEMENT_3D('',#70592,#40444,#40445) ;
#34151=AXIS2_PLACEMENT_3D('',#70595,#40447,#40448) ;
#34152=AXIS2_PLACEMENT_3D('',#70596,#40449,#40450) ;
#34153=AXIS2_PLACEMENT_3D('',#70600,#40453,#40454) ;
#34154=AXIS2_PLACEMENT_3D('',#70603,#40455,#40456) ;
#34155=AXIS2_PLACEMENT_3D('',#70607,#40458,#40459) ;
#34156=AXIS2_PLACEMENT_3D('',#70609,#40461,#40462) ;
#34157=AXIS2_PLACEMENT_3D('',#70612,#40463,#40464) ;
#34158=AXIS2_PLACEMENT_3D('',#70613,#40465,#40466) ;
#34159=AXIS2_PLACEMENT_3D('',#70614,#40467,#40468) ;
#34160=AXIS2_PLACEMENT_3D('',#70615,#40469,#40470) ;
#34161=AXIS2_PLACEMENT_3D('',#70618,#40471,#40472) ;
#34162=AXIS2_PLACEMENT_3D('',#70621,#40475,#40476) ;
#34163=AXIS2_PLACEMENT_3D('',#70624,#40477,#40478) ;
#34164=AXIS2_PLACEMENT_3D('',#70625,#40479,#40480) ;
#34165=AXIS2_PLACEMENT_3D('',#70626,#40481,#40482) ;
#34166=AXIS2_PLACEMENT_3D('',#70627,#40483,#40484) ;
#34167=AXIS2_PLACEMENT_3D('',#70630,#40485,#40486) ;
#34168=AXIS2_PLACEMENT_3D('',#70633,#40489,#40490) ;
#34169=AXIS2_PLACEMENT_3D('',#70636,#40491,#40492) ;
#34170=AXIS2_PLACEMENT_3D('',#70637,#40493,#40494) ;
#34171=AXIS2_PLACEMENT_3D('',#70638,#40495,#40496) ;
#34172=AXIS2_PLACEMENT_3D('',#70639,#40497,#40498) ;
#34173=AXIS2_PLACEMENT_3D('',#70642,#40499,#40500) ;
#34174=AXIS2_PLACEMENT_3D('',#70645,#40503,#40504) ;
#34175=AXIS2_PLACEMENT_3D('',#70646,#40505,#40506) ;
#34176=AXIS2_PLACEMENT_3D('',#70647,#40507,#40508) ;
#34177=AXIS2_PLACEMENT_3D('',#70648,#40509,#40510) ;
#34178=AXIS2_PLACEMENT_3D('',#70652,#40512,#40513) ;
#34179=AXIS2_PLACEMENT_3D('',#70654,#40515,#40516) ;
#34180=AXIS2_PLACEMENT_3D('',#70658,#40519,#40520) ;
#34181=AXIS2_PLACEMENT_3D('',#70661,#40522,#40523) ;
#34182=AXIS2_PLACEMENT_3D('',#70662,#40524,#40525) ;
#34183=AXIS2_PLACEMENT_3D('',#70666,#40528,#40529) ;
#34184=AXIS2_PLACEMENT_3D('',#70669,#40530,#40531) ;
#34185=AXIS2_PLACEMENT_3D('',#70673,#40533,#40534) ;
#34186=AXIS2_PLACEMENT_3D('',#70675,#40536,#40537) ;
#34187=AXIS2_PLACEMENT_3D('',#70678,#40538,#40539) ;
#34188=AXIS2_PLACEMENT_3D('',#70679,#40540,#40541) ;
#34189=AXIS2_PLACEMENT_3D('',#70680,#40542,#40543) ;
#34190=AXIS2_PLACEMENT_3D('',#70681,#40544,#40545) ;
#34191=AXIS2_PLACEMENT_3D('',#70684,#40546,#40547) ;
#34192=AXIS2_PLACEMENT_3D('',#70687,#40550,#40551) ;
#34193=AXIS2_PLACEMENT_3D('',#70690,#40552,#40553) ;
#34194=AXIS2_PLACEMENT_3D('',#70691,#40554,#40555) ;
#34195=AXIS2_PLACEMENT_3D('',#70692,#40556,#40557) ;
#34196=AXIS2_PLACEMENT_3D('',#70693,#40558,#40559) ;
#34197=AXIS2_PLACEMENT_3D('',#70696,#40560,#40561) ;
#34198=AXIS2_PLACEMENT_3D('',#70699,#40564,#40565) ;
#34199=AXIS2_PLACEMENT_3D('',#70702,#40566,#40567) ;
#34200=AXIS2_PLACEMENT_3D('',#70703,#40568,#40569) ;
#34201=AXIS2_PLACEMENT_3D('',#70704,#40570,#40571) ;
#34202=AXIS2_PLACEMENT_3D('',#70705,#40572,#40573) ;
#34203=AXIS2_PLACEMENT_3D('',#70708,#40574,#40575) ;
#34204=AXIS2_PLACEMENT_3D('',#70711,#40578,#40579) ;
#34205=AXIS2_PLACEMENT_3D('',#70712,#40580,#40581) ;
#34206=AXIS2_PLACEMENT_3D('',#70713,#40582,#40583) ;
#34207=AXIS2_PLACEMENT_3D('',#70714,#40584,#40585) ;
#34208=AXIS2_PLACEMENT_3D('',#70718,#40587,#40588) ;
#34209=AXIS2_PLACEMENT_3D('',#70720,#40590,#40591) ;
#34210=AXIS2_PLACEMENT_3D('',#70724,#40594,#40595) ;
#34211=AXIS2_PLACEMENT_3D('',#70727,#40597,#40598) ;
#34212=AXIS2_PLACEMENT_3D('',#70728,#40599,#40600) ;
#34213=AXIS2_PLACEMENT_3D('',#70732,#40603,#40604) ;
#34214=AXIS2_PLACEMENT_3D('',#70735,#40605,#40606) ;
#34215=AXIS2_PLACEMENT_3D('',#70739,#40608,#40609) ;
#34216=AXIS2_PLACEMENT_3D('',#70741,#40611,#40612) ;
#34217=AXIS2_PLACEMENT_3D('',#70744,#40613,#40614) ;
#34218=AXIS2_PLACEMENT_3D('',#70745,#40615,#40616) ;
#34219=AXIS2_PLACEMENT_3D('',#70746,#40617,#40618) ;
#34220=AXIS2_PLACEMENT_3D('',#70747,#40619,#40620) ;
#34221=AXIS2_PLACEMENT_3D('',#70750,#40621,#40622) ;
#34222=AXIS2_PLACEMENT_3D('',#70753,#40625,#40626) ;
#34223=AXIS2_PLACEMENT_3D('',#70756,#40627,#40628) ;
#34224=AXIS2_PLACEMENT_3D('',#70757,#40629,#40630) ;
#34225=AXIS2_PLACEMENT_3D('',#70758,#40631,#40632) ;
#34226=AXIS2_PLACEMENT_3D('',#70759,#40633,#40634) ;
#34227=AXIS2_PLACEMENT_3D('',#70762,#40635,#40636) ;
#34228=AXIS2_PLACEMENT_3D('',#70765,#40639,#40640) ;
#34229=AXIS2_PLACEMENT_3D('',#70768,#40641,#40642) ;
#34230=AXIS2_PLACEMENT_3D('',#70769,#40643,#40644) ;
#34231=AXIS2_PLACEMENT_3D('',#70770,#40645,#40646) ;
#34232=AXIS2_PLACEMENT_3D('',#70771,#40647,#40648) ;
#34233=AXIS2_PLACEMENT_3D('',#70774,#40649,#40650) ;
#34234=AXIS2_PLACEMENT_3D('',#70777,#40653,#40654) ;
#34235=AXIS2_PLACEMENT_3D('',#70778,#40655,#40656) ;
#34236=AXIS2_PLACEMENT_3D('',#70779,#40657,#40658) ;
#34237=AXIS2_PLACEMENT_3D('',#70780,#40659,#40660) ;
#34238=AXIS2_PLACEMENT_3D('',#70784,#40662,#40663) ;
#34239=AXIS2_PLACEMENT_3D('',#70786,#40665,#40666) ;
#34240=AXIS2_PLACEMENT_3D('',#70790,#40669,#40670) ;
#34241=AXIS2_PLACEMENT_3D('',#70793,#40672,#40673) ;
#34242=AXIS2_PLACEMENT_3D('',#70794,#40674,#40675) ;
#34243=AXIS2_PLACEMENT_3D('',#70798,#40678,#40679) ;
#34244=AXIS2_PLACEMENT_3D('',#70801,#40680,#40681) ;
#34245=AXIS2_PLACEMENT_3D('',#70805,#40683,#40684) ;
#34246=AXIS2_PLACEMENT_3D('',#70807,#40686,#40687) ;
#34247=AXIS2_PLACEMENT_3D('',#70810,#40688,#40689) ;
#34248=AXIS2_PLACEMENT_3D('',#70811,#40690,#40691) ;
#34249=AXIS2_PLACEMENT_3D('',#70812,#40692,#40693) ;
#34250=AXIS2_PLACEMENT_3D('',#70813,#40694,#40695) ;
#34251=AXIS2_PLACEMENT_3D('',#70816,#40696,#40697) ;
#34252=AXIS2_PLACEMENT_3D('',#70819,#40700,#40701) ;
#34253=AXIS2_PLACEMENT_3D('',#70822,#40702,#40703) ;
#34254=AXIS2_PLACEMENT_3D('',#70823,#40704,#40705) ;
#34255=AXIS2_PLACEMENT_3D('',#70824,#40706,#40707) ;
#34256=AXIS2_PLACEMENT_3D('',#70825,#40708,#40709) ;
#34257=AXIS2_PLACEMENT_3D('',#70828,#40710,#40711) ;
#34258=AXIS2_PLACEMENT_3D('',#70831,#40714,#40715) ;
#34259=AXIS2_PLACEMENT_3D('',#70834,#40716,#40717) ;
#34260=AXIS2_PLACEMENT_3D('',#70835,#40718,#40719) ;
#34261=AXIS2_PLACEMENT_3D('',#70836,#40720,#40721) ;
#34262=AXIS2_PLACEMENT_3D('',#70837,#40722,#40723) ;
#34263=AXIS2_PLACEMENT_3D('',#70840,#40724,#40725) ;
#34264=AXIS2_PLACEMENT_3D('',#70843,#40728,#40729) ;
#34265=AXIS2_PLACEMENT_3D('',#70844,#40730,#40731) ;
#34266=AXIS2_PLACEMENT_3D('',#70845,#40732,#40733) ;
#34267=AXIS2_PLACEMENT_3D('',#70846,#40734,#40735) ;
#34268=AXIS2_PLACEMENT_3D('',#70850,#40737,#40738) ;
#34269=AXIS2_PLACEMENT_3D('',#70852,#40740,#40741) ;
#34270=AXIS2_PLACEMENT_3D('',#70856,#40744,#40745) ;
#34271=AXIS2_PLACEMENT_3D('',#70859,#40747,#40748) ;
#34272=AXIS2_PLACEMENT_3D('',#70860,#40749,#40750) ;
#34273=AXIS2_PLACEMENT_3D('',#70864,#40753,#40754) ;
#34274=AXIS2_PLACEMENT_3D('',#70867,#40755,#40756) ;
#34275=AXIS2_PLACEMENT_3D('',#70871,#40758,#40759) ;
#34276=AXIS2_PLACEMENT_3D('',#70873,#40761,#40762) ;
#34277=AXIS2_PLACEMENT_3D('',#70876,#40763,#40764) ;
#34278=AXIS2_PLACEMENT_3D('',#70877,#40765,#40766) ;
#34279=AXIS2_PLACEMENT_3D('',#70878,#40767,#40768) ;
#34280=AXIS2_PLACEMENT_3D('',#70879,#40769,#40770) ;
#34281=AXIS2_PLACEMENT_3D('',#70882,#40771,#40772) ;
#34282=AXIS2_PLACEMENT_3D('',#70885,#40775,#40776) ;
#34283=AXIS2_PLACEMENT_3D('',#70888,#40777,#40778) ;
#34284=AXIS2_PLACEMENT_3D('',#70889,#40779,#40780) ;
#34285=AXIS2_PLACEMENT_3D('',#70890,#40781,#40782) ;
#34286=AXIS2_PLACEMENT_3D('',#70891,#40783,#40784) ;
#34287=AXIS2_PLACEMENT_3D('',#70894,#40785,#40786) ;
#34288=AXIS2_PLACEMENT_3D('',#70897,#40789,#40790) ;
#34289=AXIS2_PLACEMENT_3D('',#70900,#40791,#40792) ;
#34290=AXIS2_PLACEMENT_3D('',#70901,#40793,#40794) ;
#34291=AXIS2_PLACEMENT_3D('',#70902,#40795,#40796) ;
#34292=AXIS2_PLACEMENT_3D('',#70903,#40797,#40798) ;
#34293=AXIS2_PLACEMENT_3D('',#70906,#40799,#40800) ;
#34294=AXIS2_PLACEMENT_3D('',#70909,#40803,#40804) ;
#34295=AXIS2_PLACEMENT_3D('',#70910,#40805,#40806) ;
#34296=AXIS2_PLACEMENT_3D('',#70911,#40807,#40808) ;
#34297=AXIS2_PLACEMENT_3D('',#70912,#40809,#40810) ;
#34298=AXIS2_PLACEMENT_3D('',#70916,#40812,#40813) ;
#34299=AXIS2_PLACEMENT_3D('',#70918,#40815,#40816) ;
#34300=AXIS2_PLACEMENT_3D('',#70922,#40819,#40820) ;
#34301=AXIS2_PLACEMENT_3D('',#70925,#40822,#40823) ;
#34302=AXIS2_PLACEMENT_3D('',#70926,#40824,#40825) ;
#34303=AXIS2_PLACEMENT_3D('',#70930,#40828,#40829) ;
#34304=AXIS2_PLACEMENT_3D('',#70933,#40830,#40831) ;
#34305=AXIS2_PLACEMENT_3D('',#70937,#40833,#40834) ;
#34306=AXIS2_PLACEMENT_3D('',#70939,#40836,#40837) ;
#34307=AXIS2_PLACEMENT_3D('',#70942,#40838,#40839) ;
#34308=AXIS2_PLACEMENT_3D('',#70943,#40840,#40841) ;
#34309=AXIS2_PLACEMENT_3D('',#70944,#40842,#40843) ;
#34310=AXIS2_PLACEMENT_3D('',#70945,#40844,#40845) ;
#34311=AXIS2_PLACEMENT_3D('',#70948,#40846,#40847) ;
#34312=AXIS2_PLACEMENT_3D('',#70951,#40850,#40851) ;
#34313=AXIS2_PLACEMENT_3D('',#70954,#40852,#40853) ;
#34314=AXIS2_PLACEMENT_3D('',#70955,#40854,#40855) ;
#34315=AXIS2_PLACEMENT_3D('',#70956,#40856,#40857) ;
#34316=AXIS2_PLACEMENT_3D('',#70957,#40858,#40859) ;
#34317=AXIS2_PLACEMENT_3D('',#70960,#40860,#40861) ;
#34318=AXIS2_PLACEMENT_3D('',#70963,#40864,#40865) ;
#34319=AXIS2_PLACEMENT_3D('',#70966,#40866,#40867) ;
#34320=AXIS2_PLACEMENT_3D('',#70967,#40868,#40869) ;
#34321=AXIS2_PLACEMENT_3D('',#70968,#40870,#40871) ;
#34322=AXIS2_PLACEMENT_3D('',#70969,#40872,#40873) ;
#34323=AXIS2_PLACEMENT_3D('',#70972,#40874,#40875) ;
#34324=AXIS2_PLACEMENT_3D('',#70975,#40878,#40879) ;
#34325=AXIS2_PLACEMENT_3D('',#70976,#40880,#40881) ;
#34326=AXIS2_PLACEMENT_3D('',#70977,#40882,#40883) ;
#34327=AXIS2_PLACEMENT_3D('',#70978,#40884,#40885) ;
#34328=AXIS2_PLACEMENT_3D('',#70982,#40887,#40888) ;
#34329=AXIS2_PLACEMENT_3D('',#70984,#40890,#40891) ;
#34330=AXIS2_PLACEMENT_3D('',#70988,#40894,#40895) ;
#34331=AXIS2_PLACEMENT_3D('',#70991,#40897,#40898) ;
#34332=AXIS2_PLACEMENT_3D('',#70992,#40899,#40900) ;
#34333=AXIS2_PLACEMENT_3D('',#70996,#40903,#40904) ;
#34334=AXIS2_PLACEMENT_3D('',#70999,#40905,#40906) ;
#34335=AXIS2_PLACEMENT_3D('',#71003,#40908,#40909) ;
#34336=AXIS2_PLACEMENT_3D('',#71005,#40911,#40912) ;
#34337=AXIS2_PLACEMENT_3D('',#71008,#40913,#40914) ;
#34338=AXIS2_PLACEMENT_3D('',#71009,#40915,#40916) ;
#34339=AXIS2_PLACEMENT_3D('',#71010,#40917,#40918) ;
#34340=AXIS2_PLACEMENT_3D('',#71011,#40919,#40920) ;
#34341=AXIS2_PLACEMENT_3D('',#71014,#40921,#40922) ;
#34342=AXIS2_PLACEMENT_3D('',#71017,#40925,#40926) ;
#34343=AXIS2_PLACEMENT_3D('',#71020,#40927,#40928) ;
#34344=AXIS2_PLACEMENT_3D('',#71021,#40929,#40930) ;
#34345=AXIS2_PLACEMENT_3D('',#71022,#40931,#40932) ;
#34346=AXIS2_PLACEMENT_3D('',#71023,#40933,#40934) ;
#34347=AXIS2_PLACEMENT_3D('',#71026,#40935,#40936) ;
#34348=AXIS2_PLACEMENT_3D('',#71029,#40939,#40940) ;
#34349=AXIS2_PLACEMENT_3D('',#71032,#40941,#40942) ;
#34350=AXIS2_PLACEMENT_3D('',#71033,#40943,#40944) ;
#34351=AXIS2_PLACEMENT_3D('',#71034,#40945,#40946) ;
#34352=AXIS2_PLACEMENT_3D('',#71035,#40947,#40948) ;
#34353=AXIS2_PLACEMENT_3D('',#71038,#40949,#40950) ;
#34354=AXIS2_PLACEMENT_3D('',#71041,#40953,#40954) ;
#34355=AXIS2_PLACEMENT_3D('',#71042,#40955,#40956) ;
#34356=AXIS2_PLACEMENT_3D('',#71043,#40957,#40958) ;
#34357=AXIS2_PLACEMENT_3D('',#71044,#40959,#40960) ;
#34358=AXIS2_PLACEMENT_3D('',#71048,#40962,#40963) ;
#34359=AXIS2_PLACEMENT_3D('',#71050,#40965,#40966) ;
#34360=AXIS2_PLACEMENT_3D('',#71054,#40969,#40970) ;
#34361=AXIS2_PLACEMENT_3D('',#71057,#40972,#40973) ;
#34362=AXIS2_PLACEMENT_3D('',#71058,#40974,#40975) ;
#34363=AXIS2_PLACEMENT_3D('',#71062,#40978,#40979) ;
#34364=AXIS2_PLACEMENT_3D('',#71065,#40980,#40981) ;
#34365=AXIS2_PLACEMENT_3D('',#71069,#40983,#40984) ;
#34366=AXIS2_PLACEMENT_3D('',#71071,#40986,#40987) ;
#34367=AXIS2_PLACEMENT_3D('',#71074,#40988,#40989) ;
#34368=AXIS2_PLACEMENT_3D('',#71075,#40990,#40991) ;
#34369=AXIS2_PLACEMENT_3D('',#71076,#40992,#40993) ;
#34370=AXIS2_PLACEMENT_3D('',#71077,#40994,#40995) ;
#34371=AXIS2_PLACEMENT_3D('',#71080,#40996,#40997) ;
#34372=AXIS2_PLACEMENT_3D('',#71083,#41000,#41001) ;
#34373=AXIS2_PLACEMENT_3D('',#71086,#41002,#41003) ;
#34374=AXIS2_PLACEMENT_3D('',#71087,#41004,#41005) ;
#34375=AXIS2_PLACEMENT_3D('',#71088,#41006,#41007) ;
#34376=AXIS2_PLACEMENT_3D('',#71089,#41008,#41009) ;
#34377=AXIS2_PLACEMENT_3D('',#71092,#41010,#41011) ;
#34378=AXIS2_PLACEMENT_3D('',#71095,#41014,#41015) ;
#34379=AXIS2_PLACEMENT_3D('',#71097,#41016,#41017) ;
#34380=AXIS2_PLACEMENT_3D('',#71098,#41018,#41019) ;
#34381=AXIS2_PLACEMENT_3D('',#71099,#41020,#41021) ;
#34382=AXIS2_PLACEMENT_3D('',#71100,#41022,#41023) ;
#34383=AXIS2_PLACEMENT_3D('',#71102,#41024,#41025) ;
#34384=AXIS2_PLACEMENT_3D('',#71104,#41027,#41028) ;
#34385=AXIS2_PLACEMENT_3D('',#71105,#41029,#41030) ;
#34386=AXIS2_PLACEMENT_3D('',#71106,#41031,#41032) ;
#34387=AXIS2_PLACEMENT_3D('',#71107,#41033,#41034) ;
#34388=AXIS2_PLACEMENT_3D('',#71111,#41036,#41037) ;
#34389=AXIS2_PLACEMENT_3D('',#71113,#41039,#41040) ;
#34390=AXIS2_PLACEMENT_3D('',#71117,#41042,#41043) ;
#34391=AXIS2_PLACEMENT_3D('',#71124,#41047,#41048) ;
#34392=AXIS2_PLACEMENT_3D('',#71126,#41050,#41051) ;
#34393=AXIS2_PLACEMENT_3D('',#71129,#41053,#41054) ;
#34394=AXIS2_PLACEMENT_3D('',#71130,#41055,#41056) ;
#34395=AXIS2_PLACEMENT_3D('',#71134,#41059,#41060) ;
#34396=AXIS2_PLACEMENT_3D('',#71137,#41061,#41062) ;
#34397=AXIS2_PLACEMENT_3D('',#71141,#41064,#41065) ;
#34398=AXIS2_PLACEMENT_3D('',#71143,#41067,#41068) ;
#34399=AXIS2_PLACEMENT_3D('',#71146,#41069,#41070) ;
#34400=AXIS2_PLACEMENT_3D('',#71147,#41071,#41072) ;
#34401=AXIS2_PLACEMENT_3D('',#71148,#41073,#41074) ;
#34402=AXIS2_PLACEMENT_3D('',#71149,#41075,#41076) ;
#34403=AXIS2_PLACEMENT_3D('',#71152,#41077,#41078) ;
#34404=AXIS2_PLACEMENT_3D('',#71155,#41081,#41082) ;
#34405=AXIS2_PLACEMENT_3D('',#71158,#41083,#41084) ;
#34406=AXIS2_PLACEMENT_3D('',#71159,#41085,#41086) ;
#34407=AXIS2_PLACEMENT_3D('',#71160,#41087,#41088) ;
#34408=AXIS2_PLACEMENT_3D('',#71161,#41089,#41090) ;
#34409=AXIS2_PLACEMENT_3D('',#71164,#41091,#41092) ;
#34410=AXIS2_PLACEMENT_3D('',#71167,#41095,#41096) ;
#34411=AXIS2_PLACEMENT_3D('',#71169,#41097,#41098) ;
#34412=AXIS2_PLACEMENT_3D('',#71170,#41099,#41100) ;
#34413=AXIS2_PLACEMENT_3D('',#71171,#41101,#41102) ;
#34414=AXIS2_PLACEMENT_3D('',#71172,#41103,#41104) ;
#34415=AXIS2_PLACEMENT_3D('',#71174,#41105,#41106) ;
#34416=AXIS2_PLACEMENT_3D('',#71176,#41108,#41109) ;
#34417=AXIS2_PLACEMENT_3D('',#71177,#41110,#41111) ;
#34418=AXIS2_PLACEMENT_3D('',#71178,#41112,#41113) ;
#34419=AXIS2_PLACEMENT_3D('',#71179,#41114,#41115) ;
#34420=AXIS2_PLACEMENT_3D('',#71183,#41117,#41118) ;
#34421=AXIS2_PLACEMENT_3D('',#71185,#41120,#41121) ;
#34422=AXIS2_PLACEMENT_3D('',#71189,#41123,#41124) ;
#34423=AXIS2_PLACEMENT_3D('',#71196,#41128,#41129) ;
#34424=AXIS2_PLACEMENT_3D('',#71198,#41131,#41132) ;
#34425=AXIS2_PLACEMENT_3D('',#71201,#41134,#41135) ;
#34426=AXIS2_PLACEMENT_3D('',#71202,#41136,#41137) ;
#34427=AXIS2_PLACEMENT_3D('',#71206,#41140,#41141) ;
#34428=AXIS2_PLACEMENT_3D('',#71209,#41142,#41143) ;
#34429=AXIS2_PLACEMENT_3D('',#71213,#41145,#41146) ;
#34430=AXIS2_PLACEMENT_3D('',#71215,#41148,#41149) ;
#34431=AXIS2_PLACEMENT_3D('',#71218,#41150,#41151) ;
#34432=AXIS2_PLACEMENT_3D('',#71219,#41152,#41153) ;
#34433=AXIS2_PLACEMENT_3D('',#71220,#41154,#41155) ;
#34434=AXIS2_PLACEMENT_3D('',#71221,#41156,#41157) ;
#34435=AXIS2_PLACEMENT_3D('',#71224,#41158,#41159) ;
#34436=AXIS2_PLACEMENT_3D('',#71227,#41162,#41163) ;
#34437=AXIS2_PLACEMENT_3D('',#71230,#41164,#41165) ;
#34438=AXIS2_PLACEMENT_3D('',#71231,#41166,#41167) ;
#34439=AXIS2_PLACEMENT_3D('',#71232,#41168,#41169) ;
#34440=AXIS2_PLACEMENT_3D('',#71233,#41170,#41171) ;
#34441=AXIS2_PLACEMENT_3D('',#71236,#41172,#41173) ;
#34442=AXIS2_PLACEMENT_3D('',#71239,#41176,#41177) ;
#34443=AXIS2_PLACEMENT_3D('',#71241,#41178,#41179) ;
#34444=AXIS2_PLACEMENT_3D('',#71242,#41180,#41181) ;
#34445=AXIS2_PLACEMENT_3D('',#71243,#41182,#41183) ;
#34446=AXIS2_PLACEMENT_3D('',#71244,#41184,#41185) ;
#34447=AXIS2_PLACEMENT_3D('',#71246,#41186,#41187) ;
#34448=AXIS2_PLACEMENT_3D('',#71248,#41189,#41190) ;
#34449=AXIS2_PLACEMENT_3D('',#71249,#41191,#41192) ;
#34450=AXIS2_PLACEMENT_3D('',#71250,#41193,#41194) ;
#34451=AXIS2_PLACEMENT_3D('',#71251,#41195,#41196) ;
#34452=AXIS2_PLACEMENT_3D('',#71255,#41198,#41199) ;
#34453=AXIS2_PLACEMENT_3D('',#71257,#41201,#41202) ;
#34454=AXIS2_PLACEMENT_3D('',#71261,#41204,#41205) ;
#34455=AXIS2_PLACEMENT_3D('',#71268,#41209,#41210) ;
#34456=AXIS2_PLACEMENT_3D('',#71270,#41212,#41213) ;
#34457=AXIS2_PLACEMENT_3D('',#71273,#41215,#41216) ;
#34458=AXIS2_PLACEMENT_3D('',#71274,#41217,#41218) ;
#34459=AXIS2_PLACEMENT_3D('',#71278,#41221,#41222) ;
#34460=AXIS2_PLACEMENT_3D('',#71281,#41223,#41224) ;
#34461=AXIS2_PLACEMENT_3D('',#71285,#41226,#41227) ;
#34462=AXIS2_PLACEMENT_3D('',#71287,#41229,#41230) ;
#34463=AXIS2_PLACEMENT_3D('',#71290,#41231,#41232) ;
#34464=AXIS2_PLACEMENT_3D('',#71291,#41233,#41234) ;
#34465=AXIS2_PLACEMENT_3D('',#71292,#41235,#41236) ;
#34466=AXIS2_PLACEMENT_3D('',#71293,#41237,#41238) ;
#34467=AXIS2_PLACEMENT_3D('',#71296,#41239,#41240) ;
#34468=AXIS2_PLACEMENT_3D('',#71299,#41243,#41244) ;
#34469=AXIS2_PLACEMENT_3D('',#71302,#41245,#41246) ;
#34470=AXIS2_PLACEMENT_3D('',#71303,#41247,#41248) ;
#34471=AXIS2_PLACEMENT_3D('',#71304,#41249,#41250) ;
#34472=AXIS2_PLACEMENT_3D('',#71305,#41251,#41252) ;
#34473=AXIS2_PLACEMENT_3D('',#71308,#41253,#41254) ;
#34474=AXIS2_PLACEMENT_3D('',#71311,#41257,#41258) ;
#34475=AXIS2_PLACEMENT_3D('',#71313,#41259,#41260) ;
#34476=AXIS2_PLACEMENT_3D('',#71314,#41261,#41262) ;
#34477=AXIS2_PLACEMENT_3D('',#71315,#41263,#41264) ;
#34478=AXIS2_PLACEMENT_3D('',#71316,#41265,#41266) ;
#34479=AXIS2_PLACEMENT_3D('',#71318,#41267,#41268) ;
#34480=AXIS2_PLACEMENT_3D('',#71320,#41270,#41271) ;
#34481=AXIS2_PLACEMENT_3D('',#71321,#41272,#41273) ;
#34482=AXIS2_PLACEMENT_3D('',#71322,#41274,#41275) ;
#34483=AXIS2_PLACEMENT_3D('',#71323,#41276,#41277) ;
#34484=AXIS2_PLACEMENT_3D('',#71327,#41279,#41280) ;
#34485=AXIS2_PLACEMENT_3D('',#71329,#41282,#41283) ;
#34486=AXIS2_PLACEMENT_3D('',#71333,#41285,#41286) ;
#34487=AXIS2_PLACEMENT_3D('',#71340,#41290,#41291) ;
#34488=AXIS2_PLACEMENT_3D('',#71342,#41293,#41294) ;
#34489=AXIS2_PLACEMENT_3D('',#71345,#41296,#41297) ;
#34490=AXIS2_PLACEMENT_3D('',#71346,#41298,#41299) ;
#34491=AXIS2_PLACEMENT_3D('',#71350,#41302,#41303) ;
#34492=AXIS2_PLACEMENT_3D('',#71353,#41304,#41305) ;
#34493=AXIS2_PLACEMENT_3D('',#71357,#41307,#41308) ;
#34494=AXIS2_PLACEMENT_3D('',#71359,#41310,#41311) ;
#34495=AXIS2_PLACEMENT_3D('',#71362,#41312,#41313) ;
#34496=AXIS2_PLACEMENT_3D('',#71363,#41314,#41315) ;
#34497=AXIS2_PLACEMENT_3D('',#71364,#41316,#41317) ;
#34498=AXIS2_PLACEMENT_3D('',#71365,#41318,#41319) ;
#34499=AXIS2_PLACEMENT_3D('',#71368,#41320,#41321) ;
#34500=AXIS2_PLACEMENT_3D('',#71371,#41324,#41325) ;
#34501=AXIS2_PLACEMENT_3D('',#71374,#41326,#41327) ;
#34502=AXIS2_PLACEMENT_3D('',#71375,#41328,#41329) ;
#34503=AXIS2_PLACEMENT_3D('',#71376,#41330,#41331) ;
#34504=AXIS2_PLACEMENT_3D('',#71377,#41332,#41333) ;
#34505=AXIS2_PLACEMENT_3D('',#71380,#41334,#41335) ;
#34506=AXIS2_PLACEMENT_3D('',#71383,#41338,#41339) ;
#34507=AXIS2_PLACEMENT_3D('',#71385,#41340,#41341) ;
#34508=AXIS2_PLACEMENT_3D('',#71386,#41342,#41343) ;
#34509=AXIS2_PLACEMENT_3D('',#71387,#41344,#41345) ;
#34510=AXIS2_PLACEMENT_3D('',#71388,#41346,#41347) ;
#34511=AXIS2_PLACEMENT_3D('',#71390,#41348,#41349) ;
#34512=AXIS2_PLACEMENT_3D('',#71392,#41351,#41352) ;
#34513=AXIS2_PLACEMENT_3D('',#71393,#41353,#41354) ;
#34514=AXIS2_PLACEMENT_3D('',#71394,#41355,#41356) ;
#34515=AXIS2_PLACEMENT_3D('',#71395,#41357,#41358) ;
#34516=AXIS2_PLACEMENT_3D('',#71399,#41360,#41361) ;
#34517=AXIS2_PLACEMENT_3D('',#71401,#41363,#41364) ;
#34518=AXIS2_PLACEMENT_3D('',#71405,#41366,#41367) ;
#34519=AXIS2_PLACEMENT_3D('',#71412,#41371,#41372) ;
#34520=AXIS2_PLACEMENT_3D('',#71414,#41374,#41375) ;
#34521=AXIS2_PLACEMENT_3D('',#71417,#41377,#41378) ;
#34522=AXIS2_PLACEMENT_3D('',#71418,#41379,#41380) ;
#34523=AXIS2_PLACEMENT_3D('',#71422,#41383,#41384) ;
#34524=AXIS2_PLACEMENT_3D('',#71425,#41385,#41386) ;
#34525=AXIS2_PLACEMENT_3D('',#71429,#41388,#41389) ;
#34526=AXIS2_PLACEMENT_3D('',#71431,#41391,#41392) ;
#34527=AXIS2_PLACEMENT_3D('',#71434,#41393,#41394) ;
#34528=AXIS2_PLACEMENT_3D('',#71435,#41395,#41396) ;
#34529=AXIS2_PLACEMENT_3D('',#71436,#41397,#41398) ;
#34530=AXIS2_PLACEMENT_3D('',#71437,#41399,#41400) ;
#34531=AXIS2_PLACEMENT_3D('',#71440,#41401,#41402) ;
#34532=AXIS2_PLACEMENT_3D('',#71443,#41405,#41406) ;
#34533=AXIS2_PLACEMENT_3D('',#71446,#41407,#41408) ;
#34534=AXIS2_PLACEMENT_3D('',#71447,#41409,#41410) ;
#34535=AXIS2_PLACEMENT_3D('',#71448,#41411,#41412) ;
#34536=AXIS2_PLACEMENT_3D('',#71449,#41413,#41414) ;
#34537=AXIS2_PLACEMENT_3D('',#71452,#41415,#41416) ;
#34538=AXIS2_PLACEMENT_3D('',#71455,#41419,#41420) ;
#34539=AXIS2_PLACEMENT_3D('',#71457,#41421,#41422) ;
#34540=AXIS2_PLACEMENT_3D('',#71458,#41423,#41424) ;
#34541=AXIS2_PLACEMENT_3D('',#71459,#41425,#41426) ;
#34542=AXIS2_PLACEMENT_3D('',#71460,#41427,#41428) ;
#34543=AXIS2_PLACEMENT_3D('',#71462,#41429,#41430) ;
#34544=AXIS2_PLACEMENT_3D('',#71464,#41432,#41433) ;
#34545=AXIS2_PLACEMENT_3D('',#71465,#41434,#41435) ;
#34546=AXIS2_PLACEMENT_3D('',#71466,#41436,#41437) ;
#34547=AXIS2_PLACEMENT_3D('',#71467,#41438,#41439) ;
#34548=AXIS2_PLACEMENT_3D('',#71471,#41441,#41442) ;
#34549=AXIS2_PLACEMENT_3D('',#71473,#41444,#41445) ;
#34550=AXIS2_PLACEMENT_3D('',#71477,#41447,#41448) ;
#34551=AXIS2_PLACEMENT_3D('',#71484,#41452,#41453) ;
#34552=AXIS2_PLACEMENT_3D('',#71486,#41455,#41456) ;
#34553=AXIS2_PLACEMENT_3D('',#71489,#41458,#41459) ;
#34554=AXIS2_PLACEMENT_3D('',#71490,#41460,#41461) ;
#34555=AXIS2_PLACEMENT_3D('',#71494,#41464,#41465) ;
#34556=AXIS2_PLACEMENT_3D('',#71497,#41466,#41467) ;
#34557=AXIS2_PLACEMENT_3D('',#71501,#41469,#41470) ;
#34558=AXIS2_PLACEMENT_3D('',#71503,#41472,#41473) ;
#34559=AXIS2_PLACEMENT_3D('',#71506,#41474,#41475) ;
#34560=AXIS2_PLACEMENT_3D('',#71507,#41476,#41477) ;
#34561=AXIS2_PLACEMENT_3D('',#71508,#41478,#41479) ;
#34562=AXIS2_PLACEMENT_3D('',#71509,#41480,#41481) ;
#34563=AXIS2_PLACEMENT_3D('',#71512,#41482,#41483) ;
#34564=AXIS2_PLACEMENT_3D('',#71515,#41486,#41487) ;
#34565=AXIS2_PLACEMENT_3D('',#71518,#41488,#41489) ;
#34566=AXIS2_PLACEMENT_3D('',#71519,#41490,#41491) ;
#34567=AXIS2_PLACEMENT_3D('',#71520,#41492,#41493) ;
#34568=AXIS2_PLACEMENT_3D('',#71521,#41494,#41495) ;
#34569=AXIS2_PLACEMENT_3D('',#71524,#41496,#41497) ;
#34570=AXIS2_PLACEMENT_3D('',#71527,#41500,#41501) ;
#34571=AXIS2_PLACEMENT_3D('',#71529,#41502,#41503) ;
#34572=AXIS2_PLACEMENT_3D('',#71530,#41504,#41505) ;
#34573=AXIS2_PLACEMENT_3D('',#71531,#41506,#41507) ;
#34574=AXIS2_PLACEMENT_3D('',#71532,#41508,#41509) ;
#34575=AXIS2_PLACEMENT_3D('',#71534,#41510,#41511) ;
#34576=AXIS2_PLACEMENT_3D('',#71536,#41513,#41514) ;
#34577=AXIS2_PLACEMENT_3D('',#71537,#41515,#41516) ;
#34578=AXIS2_PLACEMENT_3D('',#71538,#41517,#41518) ;
#34579=AXIS2_PLACEMENT_3D('',#71539,#41519,#41520) ;
#34580=AXIS2_PLACEMENT_3D('',#71543,#41522,#41523) ;
#34581=AXIS2_PLACEMENT_3D('',#71545,#41525,#41526) ;
#34582=AXIS2_PLACEMENT_3D('',#71549,#41528,#41529) ;
#34583=AXIS2_PLACEMENT_3D('',#71556,#41533,#41534) ;
#34584=AXIS2_PLACEMENT_3D('',#71558,#41536,#41537) ;
#34585=AXIS2_PLACEMENT_3D('',#71561,#41539,#41540) ;
#34586=AXIS2_PLACEMENT_3D('',#71562,#41541,#41542) ;
#34587=AXIS2_PLACEMENT_3D('',#71566,#41545,#41546) ;
#34588=AXIS2_PLACEMENT_3D('',#71569,#41547,#41548) ;
#34589=AXIS2_PLACEMENT_3D('',#71573,#41550,#41551) ;
#34590=AXIS2_PLACEMENT_3D('',#71575,#41553,#41554) ;
#34591=AXIS2_PLACEMENT_3D('',#71578,#41555,#41556) ;
#34592=AXIS2_PLACEMENT_3D('',#71579,#41557,#41558) ;
#34593=AXIS2_PLACEMENT_3D('',#71580,#41559,#41560) ;
#34594=AXIS2_PLACEMENT_3D('',#71581,#41561,#41562) ;
#34595=AXIS2_PLACEMENT_3D('',#71584,#41563,#41564) ;
#34596=AXIS2_PLACEMENT_3D('',#71587,#41567,#41568) ;
#34597=AXIS2_PLACEMENT_3D('',#71590,#41569,#41570) ;
#34598=AXIS2_PLACEMENT_3D('',#71591,#41571,#41572) ;
#34599=AXIS2_PLACEMENT_3D('',#71592,#41573,#41574) ;
#34600=AXIS2_PLACEMENT_3D('',#71593,#41575,#41576) ;
#34601=AXIS2_PLACEMENT_3D('',#71596,#41577,#41578) ;
#34602=AXIS2_PLACEMENT_3D('',#71599,#41581,#41582) ;
#34603=AXIS2_PLACEMENT_3D('',#71601,#41583,#41584) ;
#34604=AXIS2_PLACEMENT_3D('',#71602,#41585,#41586) ;
#34605=AXIS2_PLACEMENT_3D('',#71603,#41587,#41588) ;
#34606=AXIS2_PLACEMENT_3D('',#71604,#41589,#41590) ;
#34607=AXIS2_PLACEMENT_3D('',#71606,#41591,#41592) ;
#34608=AXIS2_PLACEMENT_3D('',#71608,#41594,#41595) ;
#34609=AXIS2_PLACEMENT_3D('',#71609,#41596,#41597) ;
#34610=AXIS2_PLACEMENT_3D('',#71610,#41598,#41599) ;
#34611=AXIS2_PLACEMENT_3D('',#71611,#41600,#41601) ;
#34612=AXIS2_PLACEMENT_3D('',#71615,#41603,#41604) ;
#34613=AXIS2_PLACEMENT_3D('',#71617,#41606,#41607) ;
#34614=AXIS2_PLACEMENT_3D('',#71621,#41609,#41610) ;
#34615=AXIS2_PLACEMENT_3D('',#71628,#41614,#41615) ;
#34616=AXIS2_PLACEMENT_3D('',#71630,#41617,#41618) ;
#34617=AXIS2_PLACEMENT_3D('',#71633,#41620,#41621) ;
#34618=AXIS2_PLACEMENT_3D('',#71634,#41622,#41623) ;
#34619=AXIS2_PLACEMENT_3D('',#71638,#41626,#41627) ;
#34620=AXIS2_PLACEMENT_3D('',#71641,#41628,#41629) ;
#34621=AXIS2_PLACEMENT_3D('',#71645,#41631,#41632) ;
#34622=AXIS2_PLACEMENT_3D('',#71647,#41634,#41635) ;
#34623=AXIS2_PLACEMENT_3D('',#71650,#41636,#41637) ;
#34624=AXIS2_PLACEMENT_3D('',#71651,#41638,#41639) ;
#34625=AXIS2_PLACEMENT_3D('',#71652,#41640,#41641) ;
#34626=AXIS2_PLACEMENT_3D('',#71653,#41642,#41643) ;
#34627=AXIS2_PLACEMENT_3D('',#71656,#41644,#41645) ;
#34628=AXIS2_PLACEMENT_3D('',#71659,#41648,#41649) ;
#34629=AXIS2_PLACEMENT_3D('',#71662,#41650,#41651) ;
#34630=AXIS2_PLACEMENT_3D('',#71663,#41652,#41653) ;
#34631=AXIS2_PLACEMENT_3D('',#71664,#41654,#41655) ;
#34632=AXIS2_PLACEMENT_3D('',#71665,#41656,#41657) ;
#34633=AXIS2_PLACEMENT_3D('',#71668,#41658,#41659) ;
#34634=AXIS2_PLACEMENT_3D('',#71671,#41662,#41663) ;
#34635=AXIS2_PLACEMENT_3D('',#71674,#41664,#41665) ;
#34636=AXIS2_PLACEMENT_3D('',#71675,#41666,#41667) ;
#34637=AXIS2_PLACEMENT_3D('',#71676,#41668,#41669) ;
#34638=AXIS2_PLACEMENT_3D('',#71677,#41670,#41671) ;
#34639=AXIS2_PLACEMENT_3D('',#71680,#41672,#41673) ;
#34640=AXIS2_PLACEMENT_3D('',#71683,#41676,#41677) ;
#34641=AXIS2_PLACEMENT_3D('',#71684,#41678,#41679) ;
#34642=AXIS2_PLACEMENT_3D('',#71685,#41680,#41681) ;
#34643=AXIS2_PLACEMENT_3D('',#71686,#41682,#41683) ;
#34644=AXIS2_PLACEMENT_3D('',#71690,#41685,#41686) ;
#34645=AXIS2_PLACEMENT_3D('',#71692,#41688,#41689) ;
#34646=AXIS2_PLACEMENT_3D('',#71696,#41692,#41693) ;
#34647=AXIS2_PLACEMENT_3D('',#71699,#41695,#41696) ;
#34648=AXIS2_PLACEMENT_3D('',#71700,#41697,#41698) ;
#34649=AXIS2_PLACEMENT_3D('',#71704,#41701,#41702) ;
#34650=AXIS2_PLACEMENT_3D('',#71717,#41708,#41709) ;
#34651=AXIS2_PLACEMENT_3D('',#71721,#41711,#41712) ;
#34652=AXIS2_PLACEMENT_3D('',#71725,#41714,#41715) ;
#34653=AXIS2_PLACEMENT_3D('',#71728,#41717,#41718) ;
#34654=AXIS2_PLACEMENT_3D('',#71730,#41719,#41720) ;
#34655=AXIS2_PLACEMENT_3D('',#71731,#41721,#41722) ;
#34656=AXIS2_PLACEMENT_3D('',#71733,#41723,#41724) ;
#34657=AXIS2_PLACEMENT_3D('',#71736,#41726,#41727) ;
#34658=AXIS2_PLACEMENT_3D('',#71737,#41728,#41729) ;
#34659=AXIS2_PLACEMENT_3D('',#71739,#41730,#41731) ;
#34660=AXIS2_PLACEMENT_3D('',#71740,#41732,#41733) ;
#34661=AXIS2_PLACEMENT_3D('',#71741,#41734,#41735) ;
#34662=AXIS2_PLACEMENT_3D('',#71743,#41736,#41737) ;
#34663=AXIS2_PLACEMENT_3D('',#71745,#41739,#41740) ;
#34664=AXIS2_PLACEMENT_3D('',#71747,#41741,#41742) ;
#34665=AXIS2_PLACEMENT_3D('',#71748,#41743,#41744) ;
#34666=AXIS2_PLACEMENT_3D('',#71749,#41745,#41746) ;
#34667=AXIS2_PLACEMENT_3D('',#71751,#41747,#41748) ;
#34668=AXIS2_PLACEMENT_3D('',#71753,#41750,#41751) ;
#34669=AXIS2_PLACEMENT_3D('',#71754,#41752,#41753) ;
#34670=AXIS2_PLACEMENT_3D('',#71755,#41754,#41755) ;
#34671=AXIS2_PLACEMENT_3D('',#71756,#41756,#41757) ;
#34672=AXIS2_PLACEMENT_3D('',#71757,#41758,#41759) ;
#34673=AXIS2_PLACEMENT_3D('',#71758,#41760,#41761) ;
#34674=AXIS2_PLACEMENT_3D('',#71759,#41762,#41763) ;
#34675=AXIS2_PLACEMENT_3D('',#71760,#41764,#41765) ;
#34676=AXIS2_PLACEMENT_3D('',#71764,#41767,#41768) ;
#34677=AXIS2_PLACEMENT_3D('',#71766,#41770,#41771) ;
#34678=AXIS2_PLACEMENT_3D('',#71772,#41774,#41775) ;
#34679=AXIS2_PLACEMENT_3D('',#71777,#41778,#41779) ;
#34680=AXIS2_PLACEMENT_3D('',#71779,#41781,#41782) ;
#34681=AXIS2_PLACEMENT_3D('',#71782,#41784,#41785) ;
#34682=AXIS2_PLACEMENT_3D('',#71783,#41786,#41787) ;
#34683=AXIS2_PLACEMENT_3D('',#71787,#41790,#41791) ;
#34684=AXIS2_PLACEMENT_3D('',#71791,#41794,#41795) ;
#34685=AXIS2_PLACEMENT_3D('',#71792,#41796,#41797) ;
#34686=AXIS2_PLACEMENT_3D('',#71793,#41798,#41799) ;
#34687=AXIS2_PLACEMENT_3D('',#71794,#41800,#41801) ;
#34688=AXIS2_PLACEMENT_3D('',#71795,#41802,#41803) ;
#34689=AXIS2_PLACEMENT_3D('',#71799,#41806,#41807) ;
#34690=AXIS2_PLACEMENT_3D('',#71801,#41808,#41809) ;
#34691=AXIS2_PLACEMENT_3D('',#71803,#41811,#41812) ;
#34692=AXIS2_PLACEMENT_3D('',#71806,#41814,#41815) ;
#34693=AXIS2_PLACEMENT_3D('',#71807,#41816,#41817) ;
#34694=AXIS2_PLACEMENT_3D('',#71809,#41819,#41820) ;
#34695=AXIS2_PLACEMENT_3D('',#71811,#41821,#41822) ;
#34696=AXIS2_PLACEMENT_3D('',#71812,#41823,#41824) ;
#34697=AXIS2_PLACEMENT_3D('',#71813,#41825,#41826) ;
#34698=AXIS2_PLACEMENT_3D('',#71814,#41827,#41828) ;
#34699=AXIS2_PLACEMENT_3D('',#71816,#41829,#41830) ;
#34700=AXIS2_PLACEMENT_3D('',#71818,#41831,#41832) ;
#34701=AXIS2_PLACEMENT_3D('',#71820,#41834,#41835) ;
#34702=AXIS2_PLACEMENT_3D('',#71822,#41836,#41837) ;
#34703=AXIS2_PLACEMENT_3D('',#71823,#41838,#41839) ;
#34704=AXIS2_PLACEMENT_3D('',#71824,#41840,#41841) ;
#34705=AXIS2_PLACEMENT_3D('',#71826,#41842,#41843) ;
#34706=AXIS2_PLACEMENT_3D('',#71828,#41845,#41846) ;
#34707=AXIS2_PLACEMENT_3D('',#71830,#41847,#41848) ;
#34708=AXIS2_PLACEMENT_3D('',#71831,#41849,#41850) ;
#34709=AXIS2_PLACEMENT_3D('',#71832,#41851,#41852) ;
#34710=AXIS2_PLACEMENT_3D('',#71835,#41853,#41854) ;
#34711=AXIS2_PLACEMENT_3D('',#71836,#41855,#41856) ;
#34712=AXIS2_PLACEMENT_3D('',#71837,#41857,#41858) ;
#34713=AXIS2_PLACEMENT_3D('',#71838,#41859,#41860) ;
#34714=AXIS2_PLACEMENT_3D('',#71840,#41862,#41863) ;
#34715=AXIS2_PLACEMENT_3D('',#71841,#41864,#41865) ;
#34716=AXIS2_PLACEMENT_3D('',#71843,#41867,#41868) ;
#34717=AXIS2_PLACEMENT_3D('',#71845,#41869,#41870) ;
#34718=AXIS2_PLACEMENT_3D('',#71846,#41871,#41872) ;
#34719=AXIS2_PLACEMENT_3D('',#71847,#41873,#41874) ;
#34720=AXIS2_PLACEMENT_3D('',#71848,#41875,#41876) ;
#34721=AXIS2_PLACEMENT_3D('',#71850,#41878,#41879) ;
#34722=AXIS2_PLACEMENT_3D('',#71853,#41882,#41883) ;
#34723=AXIS2_PLACEMENT_3D('',#71855,#41884,#41885) ;
#34724=AXIS2_PLACEMENT_3D('',#71857,#41887,#41888) ;
#34725=AXIS2_PLACEMENT_3D('',#71859,#41890,#41891) ;
#34726=AXIS2_PLACEMENT_3D('',#71860,#41892,#41893) ;
#34727=AXIS2_PLACEMENT_3D('',#71861,#41894,#41895) ;
#34728=AXIS2_PLACEMENT_3D('',#71862,#41896,#41897) ;
#34729=AXIS2_PLACEMENT_3D('',#71864,#41899,#41900) ;
#34730=AXIS2_PLACEMENT_3D('',#71865,#41901,#41902) ;
#34731=AXIS2_PLACEMENT_3D('',#71866,#41903,#41904) ;
#34732=AXIS2_PLACEMENT_3D('',#71867,#41905,#41906) ;
#34733=AXIS2_PLACEMENT_3D('',#71868,#41907,#41908) ;
#34734=AXIS2_PLACEMENT_3D('',#71869,#41909,#41910) ;
#34735=AXIS2_PLACEMENT_3D('',#71870,#41911,#41912) ;
#34736=AXIS2_PLACEMENT_3D('',#71879,#41917,#41918) ;
#34737=AXIS2_PLACEMENT_3D('',#71880,#41919,#41920) ;
#34738=AXIS2_PLACEMENT_3D('',#71881,#41921,#41922) ;
#34739=AXIS2_PLACEMENT_3D('',#71882,#41923,#41924) ;
#34740=AXIS2_PLACEMENT_3D('',#71883,#41925,#41926) ;
#34741=AXIS2_PLACEMENT_3D('',#71884,#41927,#41928) ;
#34742=AXIS2_PLACEMENT_3D('',#71885,#41929,#41930) ;
#34743=AXIS2_PLACEMENT_3D('',#71886,#41931,#41932) ;
#34744=AXIS2_PLACEMENT_3D('',#71887,#41933,#41934) ;
#34745=AXIS2_PLACEMENT_3D('',#71888,#41935,#41936) ;
#34746=AXIS2_PLACEMENT_3D('',#71889,#41937,#41938) ;
#34747=AXIS2_PLACEMENT_3D('',#71890,#41939,#41940) ;
#34748=AXIS2_PLACEMENT_3D('',#71891,#41941,#41942) ;
#34749=AXIS2_PLACEMENT_3D('',#71892,#41943,#41944) ;
#34750=AXIS2_PLACEMENT_3D('',#71893,#41945,#41946) ;
#34751=AXIS2_PLACEMENT_3D('',#71894,#41947,#41948) ;
#34752=AXIS2_PLACEMENT_3D('',#71895,#41949,#41950) ;
#34753=AXIS2_PLACEMENT_3D('',#71896,#41951,#41952) ;
#34754=AXIS2_PLACEMENT_3D('',#71897,#41953,#41954) ;
#34755=AXIS2_PLACEMENT_3D('',#71900,#41955,#41956) ;
#34756=AXIS2_PLACEMENT_3D('',#71903,#41958,#41959) ;
#34757=AXIS2_PLACEMENT_3D('',#71905,#41961,#41962) ;
#34758=AXIS2_PLACEMENT_3D('',#71907,#41963,#41964) ;
#34759=AXIS2_PLACEMENT_3D('',#71908,#41965,#41966) ;
#34760=AXIS2_PLACEMENT_3D('',#71909,#41967,#41968) ;
#34761=AXIS2_PLACEMENT_3D('',#71911,#41969,#41970) ;
#34762=AXIS2_PLACEMENT_3D('',#71913,#41972,#41973) ;
#34763=AXIS2_PLACEMENT_3D('',#71915,#41974,#41975) ;
#34764=AXIS2_PLACEMENT_3D('',#71916,#41976,#41977) ;
#34765=AXIS2_PLACEMENT_3D('',#71917,#41978,#41979) ;
#34766=AXIS2_PLACEMENT_3D('',#71920,#41980,#41981) ;
#34767=AXIS2_PLACEMENT_3D('',#71921,#41982,#41983) ;
#34768=AXIS2_PLACEMENT_3D('',#71922,#41984,#41985) ;
#34769=AXIS2_PLACEMENT_3D('',#71923,#41986,#41987) ;
#34770=AXIS2_PLACEMENT_3D('',#71925,#41989,#41990) ;
#34771=AXIS2_PLACEMENT_3D('',#71926,#41991,#41992) ;
#34772=AXIS2_PLACEMENT_3D('',#71928,#41994,#41995) ;
#34773=AXIS2_PLACEMENT_3D('',#71930,#41996,#41997) ;
#34774=AXIS2_PLACEMENT_3D('',#71931,#41998,#41999) ;
#34775=AXIS2_PLACEMENT_3D('',#71932,#42000,#42001) ;
#34776=AXIS2_PLACEMENT_3D('',#71933,#42002,#42003) ;
#34777=AXIS2_PLACEMENT_3D('',#71935,#42005,#42006) ;
#34778=AXIS2_PLACEMENT_3D('',#71938,#42009,#42010) ;
#34779=AXIS2_PLACEMENT_3D('',#71940,#42011,#42012) ;
#34780=AXIS2_PLACEMENT_3D('',#71942,#42014,#42015) ;
#34781=AXIS2_PLACEMENT_3D('',#71944,#42017,#42018) ;
#34782=AXIS2_PLACEMENT_3D('',#71945,#42019,#42020) ;
#34783=AXIS2_PLACEMENT_3D('',#71946,#42021,#42022) ;
#34784=AXIS2_PLACEMENT_3D('',#71947,#42023,#42024) ;
#34785=AXIS2_PLACEMENT_3D('',#71948,#42025,#42026) ;
#34786=AXIS2_PLACEMENT_3D('',#71950,#42028,#42029) ;
#34787=AXIS2_PLACEMENT_3D('',#71951,#42030,#42031) ;
#34788=AXIS2_PLACEMENT_3D('',#71952,#42032,#42033) ;
#34789=AXIS2_PLACEMENT_3D('',#71953,#42034,#42035) ;
#34790=AXIS2_PLACEMENT_3D('',#71954,#42036,#42037) ;
#34791=AXIS2_PLACEMENT_3D('',#71955,#42038,#42039) ;
#34792=AXIS2_PLACEMENT_3D('',#71956,#42040,#42041) ;
#34793=AXIS2_PLACEMENT_3D('',#71957,#42042,#42043) ;
#34794=AXIS2_PLACEMENT_3D('',#71966,#42048,#42049) ;
#34795=AXIS2_PLACEMENT_3D('',#71968,#42050,#42051) ;
#34796=AXIS2_PLACEMENT_3D('',#71970,#42052,#42053) ;
#34797=AXIS2_PLACEMENT_3D('',#71971,#42054,#42055) ;
#34798=AXIS2_PLACEMENT_3D('',#71972,#42056,#42057) ;
#34799=AXIS2_PLACEMENT_3D('',#71974,#42058,#42059) ;
#34800=AXIS2_PLACEMENT_3D('',#71975,#42060,#42061) ;
#34801=AXIS2_PLACEMENT_3D('',#71976,#42062,#42063) ;
#34802=AXIS2_PLACEMENT_3D('',#71977,#42064,#42065) ;
#34803=AXIS2_PLACEMENT_3D('',#71979,#42067,#42068) ;
#34804=AXIS2_PLACEMENT_3D('',#71980,#42069,#42070) ;
#34805=AXIS2_PLACEMENT_3D('',#71981,#42071,#42072) ;
#34806=AXIS2_PLACEMENT_3D('',#71983,#42074,#42075) ;
#34807=AXIS2_PLACEMENT_3D('',#71984,#42076,#42077) ;
#34808=AXIS2_PLACEMENT_3D('',#71985,#42078,#42079) ;
#34809=AXIS2_PLACEMENT_3D('',#71986,#42080,#42081) ;
#34810=AXIS2_PLACEMENT_3D('',#71987,#42082,#42083) ;
#34811=AXIS2_PLACEMENT_3D('',#71988,#42084,#42085) ;
#34812=AXIS2_PLACEMENT_3D('',#71989,#42086,#42087) ;
#34813=AXIS2_PLACEMENT_3D('',#71990,#42088,#42089) ;
#34814=AXIS2_PLACEMENT_3D('',#71991,#42090,#42091) ;
#34815=AXIS2_PLACEMENT_3D('',#71994,#42092,#42093) ;
#34816=AXIS2_PLACEMENT_3D('',#71997,#42095,#42096) ;
#34817=AXIS2_PLACEMENT_3D('',#71999,#42098,#42099) ;
#34818=AXIS2_PLACEMENT_3D('',#72001,#42100,#42101) ;
#34819=AXIS2_PLACEMENT_3D('',#72002,#42102,#42103) ;
#34820=AXIS2_PLACEMENT_3D('',#72003,#42104,#42105) ;
#34821=AXIS2_PLACEMENT_3D('',#72005,#42106,#42107) ;
#34822=AXIS2_PLACEMENT_3D('',#72007,#42109,#42110) ;
#34823=AXIS2_PLACEMENT_3D('',#72009,#42111,#42112) ;
#34824=AXIS2_PLACEMENT_3D('',#72010,#42113,#42114) ;
#34825=AXIS2_PLACEMENT_3D('',#72011,#42115,#42116) ;
#34826=AXIS2_PLACEMENT_3D('',#72014,#42117,#42118) ;
#34827=AXIS2_PLACEMENT_3D('',#72015,#42119,#42120) ;
#34828=AXIS2_PLACEMENT_3D('',#72016,#42121,#42122) ;
#34829=AXIS2_PLACEMENT_3D('',#72017,#42123,#42124) ;
#34830=AXIS2_PLACEMENT_3D('',#72019,#42126,#42127) ;
#34831=AXIS2_PLACEMENT_3D('',#72020,#42128,#42129) ;
#34832=AXIS2_PLACEMENT_3D('',#72022,#42131,#42132) ;
#34833=AXIS2_PLACEMENT_3D('',#72024,#42133,#42134) ;
#34834=AXIS2_PLACEMENT_3D('',#72025,#42135,#42136) ;
#34835=AXIS2_PLACEMENT_3D('',#72026,#42137,#42138) ;
#34836=AXIS2_PLACEMENT_3D('',#72027,#42139,#42140) ;
#34837=AXIS2_PLACEMENT_3D('',#72029,#42142,#42143) ;
#34838=AXIS2_PLACEMENT_3D('',#72032,#42146,#42147) ;
#34839=AXIS2_PLACEMENT_3D('',#72034,#42148,#42149) ;
#34840=AXIS2_PLACEMENT_3D('',#72036,#42151,#42152) ;
#34841=AXIS2_PLACEMENT_3D('',#72038,#42154,#42155) ;
#34842=AXIS2_PLACEMENT_3D('',#72039,#42156,#42157) ;
#34843=AXIS2_PLACEMENT_3D('',#72040,#42158,#42159) ;
#34844=AXIS2_PLACEMENT_3D('',#72041,#42160,#42161) ;
#34845=AXIS2_PLACEMENT_3D('',#72042,#42162,#42163) ;
#34846=AXIS2_PLACEMENT_3D('',#72044,#42165,#42166) ;
#34847=AXIS2_PLACEMENT_3D('',#72045,#42167,#42168) ;
#34848=AXIS2_PLACEMENT_3D('',#72046,#42169,#42170) ;
#34849=AXIS2_PLACEMENT_3D('',#72047,#42171,#42172) ;
#34850=AXIS2_PLACEMENT_3D('',#72048,#42173,#42174) ;
#34851=AXIS2_PLACEMENT_3D('',#72049,#42175,#42176) ;
#34852=AXIS2_PLACEMENT_3D('',#72050,#42177,#42178) ;
#34853=AXIS2_PLACEMENT_3D('',#72051,#42179,#42180) ;
#34854=AXIS2_PLACEMENT_3D('',#72060,#42185,#42186) ;
#34855=AXIS2_PLACEMENT_3D('',#72062,#42187,#42188) ;
#34856=AXIS2_PLACEMENT_3D('',#72064,#42189,#42190) ;
#34857=AXIS2_PLACEMENT_3D('',#72065,#42191,#42192) ;
#34858=AXIS2_PLACEMENT_3D('',#72066,#42193,#42194) ;
#34859=AXIS2_PLACEMENT_3D('',#72068,#42195,#42196) ;
#34860=AXIS2_PLACEMENT_3D('',#72069,#42197,#42198) ;
#34861=AXIS2_PLACEMENT_3D('',#72070,#42199,#42200) ;
#34862=AXIS2_PLACEMENT_3D('',#72071,#42201,#42202) ;
#34863=AXIS2_PLACEMENT_3D('',#72073,#42204,#42205) ;
#34864=AXIS2_PLACEMENT_3D('',#72074,#42206,#42207) ;
#34865=AXIS2_PLACEMENT_3D('',#72075,#42208,#42209) ;
#34866=AXIS2_PLACEMENT_3D('',#72077,#42211,#42212) ;
#34867=AXIS2_PLACEMENT_3D('',#72078,#42213,#42214) ;
#34868=AXIS2_PLACEMENT_3D('',#72079,#42215,#42216) ;
#34869=AXIS2_PLACEMENT_3D('',#72080,#42217,#42218) ;
#34870=AXIS2_PLACEMENT_3D('',#72081,#42219,#42220) ;
#34871=AXIS2_PLACEMENT_3D('',#72082,#42221,#42222) ;
#34872=AXIS2_PLACEMENT_3D('',#72083,#42223,#42224) ;
#34873=AXIS2_PLACEMENT_3D('',#72084,#42225,#42226) ;
#34874=AXIS2_PLACEMENT_3D('',#72085,#42227,#42228) ;
#34875=AXIS2_PLACEMENT_3D('',#72088,#42229,#42230) ;
#34876=AXIS2_PLACEMENT_3D('',#72091,#42232,#42233) ;
#34877=AXIS2_PLACEMENT_3D('',#72093,#42235,#42236) ;
#34878=AXIS2_PLACEMENT_3D('',#72095,#42237,#42238) ;
#34879=AXIS2_PLACEMENT_3D('',#72096,#42239,#42240) ;
#34880=AXIS2_PLACEMENT_3D('',#72097,#42241,#42242) ;
#34881=AXIS2_PLACEMENT_3D('',#72099,#42243,#42244) ;
#34882=AXIS2_PLACEMENT_3D('',#72101,#42246,#42247) ;
#34883=AXIS2_PLACEMENT_3D('',#72103,#42248,#42249) ;
#34884=AXIS2_PLACEMENT_3D('',#72104,#42250,#42251) ;
#34885=AXIS2_PLACEMENT_3D('',#72105,#42252,#42253) ;
#34886=AXIS2_PLACEMENT_3D('',#72108,#42254,#42255) ;
#34887=AXIS2_PLACEMENT_3D('',#72109,#42256,#42257) ;
#34888=AXIS2_PLACEMENT_3D('',#72110,#42258,#42259) ;
#34889=AXIS2_PLACEMENT_3D('',#72111,#42260,#42261) ;
#34890=AXIS2_PLACEMENT_3D('',#72113,#42263,#42264) ;
#34891=AXIS2_PLACEMENT_3D('',#72114,#42265,#42266) ;
#34892=AXIS2_PLACEMENT_3D('',#72116,#42268,#42269) ;
#34893=AXIS2_PLACEMENT_3D('',#72118,#42270,#42271) ;
#34894=AXIS2_PLACEMENT_3D('',#72119,#42272,#42273) ;
#34895=AXIS2_PLACEMENT_3D('',#72120,#42274,#42275) ;
#34896=AXIS2_PLACEMENT_3D('',#72121,#42276,#42277) ;
#34897=AXIS2_PLACEMENT_3D('',#72123,#42279,#42280) ;
#34898=AXIS2_PLACEMENT_3D('',#72126,#42283,#42284) ;
#34899=AXIS2_PLACEMENT_3D('',#72128,#42285,#42286) ;
#34900=AXIS2_PLACEMENT_3D('',#72130,#42288,#42289) ;
#34901=AXIS2_PLACEMENT_3D('',#72132,#42291,#42292) ;
#34902=AXIS2_PLACEMENT_3D('',#72133,#42293,#42294) ;
#34903=AXIS2_PLACEMENT_3D('',#72134,#42295,#42296) ;
#34904=AXIS2_PLACEMENT_3D('',#72135,#42297,#42298) ;
#34905=AXIS2_PLACEMENT_3D('',#72136,#42299,#42300) ;
#34906=AXIS2_PLACEMENT_3D('',#72138,#42302,#42303) ;
#34907=AXIS2_PLACEMENT_3D('',#72139,#42304,#42305) ;
#34908=AXIS2_PLACEMENT_3D('',#72140,#42306,#42307) ;
#34909=AXIS2_PLACEMENT_3D('',#72141,#42308,#42309) ;
#34910=AXIS2_PLACEMENT_3D('',#72142,#42310,#42311) ;
#34911=AXIS2_PLACEMENT_3D('',#72143,#42312,#42313) ;
#34912=AXIS2_PLACEMENT_3D('',#72144,#42314,#42315) ;
#34913=AXIS2_PLACEMENT_3D('',#72145,#42316,#42317) ;
#34914=AXIS2_PLACEMENT_3D('',#72154,#42322,#42323) ;
#34915=AXIS2_PLACEMENT_3D('',#72156,#42324,#42325) ;
#34916=AXIS2_PLACEMENT_3D('',#72158,#42326,#42327) ;
#34917=AXIS2_PLACEMENT_3D('',#72159,#42328,#42329) ;
#34918=AXIS2_PLACEMENT_3D('',#72160,#42330,#42331) ;
#34919=AXIS2_PLACEMENT_3D('',#72162,#42332,#42333) ;
#34920=AXIS2_PLACEMENT_3D('',#72163,#42334,#42335) ;
#34921=AXIS2_PLACEMENT_3D('',#72164,#42336,#42337) ;
#34922=AXIS2_PLACEMENT_3D('',#72165,#42338,#42339) ;
#34923=AXIS2_PLACEMENT_3D('',#72167,#42341,#42342) ;
#34924=AXIS2_PLACEMENT_3D('',#72168,#42343,#42344) ;
#34925=AXIS2_PLACEMENT_3D('',#72169,#42345,#42346) ;
#34926=AXIS2_PLACEMENT_3D('',#72171,#42348,#42349) ;
#34927=AXIS2_PLACEMENT_3D('',#72172,#42350,#42351) ;
#34928=AXIS2_PLACEMENT_3D('',#72173,#42352,#42353) ;
#34929=AXIS2_PLACEMENT_3D('',#72174,#42354,#42355) ;
#34930=AXIS2_PLACEMENT_3D('',#72175,#42356,#42357) ;
#34931=AXIS2_PLACEMENT_3D('',#72176,#42358,#42359) ;
#34932=AXIS2_PLACEMENT_3D('',#72177,#42360,#42361) ;
#34933=AXIS2_PLACEMENT_3D('',#72178,#42362,#42363) ;
#34934=AXIS2_PLACEMENT_3D('',#72179,#42364,#42365) ;
#34935=AXIS2_PLACEMENT_3D('',#72182,#42366,#42367) ;
#34936=AXIS2_PLACEMENT_3D('',#72185,#42369,#42370) ;
#34937=AXIS2_PLACEMENT_3D('',#72187,#42372,#42373) ;
#34938=AXIS2_PLACEMENT_3D('',#72189,#42374,#42375) ;
#34939=AXIS2_PLACEMENT_3D('',#72190,#42376,#42377) ;
#34940=AXIS2_PLACEMENT_3D('',#72191,#42378,#42379) ;
#34941=AXIS2_PLACEMENT_3D('',#72193,#42380,#42381) ;
#34942=AXIS2_PLACEMENT_3D('',#72195,#42383,#42384) ;
#34943=AXIS2_PLACEMENT_3D('',#72197,#42385,#42386) ;
#34944=AXIS2_PLACEMENT_3D('',#72198,#42387,#42388) ;
#34945=AXIS2_PLACEMENT_3D('',#72199,#42389,#42390) ;
#34946=AXIS2_PLACEMENT_3D('',#72202,#42391,#42392) ;
#34947=AXIS2_PLACEMENT_3D('',#72203,#42393,#42394) ;
#34948=AXIS2_PLACEMENT_3D('',#72204,#42395,#42396) ;
#34949=AXIS2_PLACEMENT_3D('',#72205,#42397,#42398) ;
#34950=AXIS2_PLACEMENT_3D('',#72207,#42400,#42401) ;
#34951=AXIS2_PLACEMENT_3D('',#72208,#42402,#42403) ;
#34952=AXIS2_PLACEMENT_3D('',#72210,#42405,#42406) ;
#34953=AXIS2_PLACEMENT_3D('',#72212,#42407,#42408) ;
#34954=AXIS2_PLACEMENT_3D('',#72213,#42409,#42410) ;
#34955=AXIS2_PLACEMENT_3D('',#72214,#42411,#42412) ;
#34956=AXIS2_PLACEMENT_3D('',#72215,#42413,#42414) ;
#34957=AXIS2_PLACEMENT_3D('',#72217,#42416,#42417) ;
#34958=AXIS2_PLACEMENT_3D('',#72220,#42420,#42421) ;
#34959=AXIS2_PLACEMENT_3D('',#72222,#42422,#42423) ;
#34960=AXIS2_PLACEMENT_3D('',#72224,#42425,#42426) ;
#34961=AXIS2_PLACEMENT_3D('',#72226,#42428,#42429) ;
#34962=AXIS2_PLACEMENT_3D('',#72227,#42430,#42431) ;
#34963=AXIS2_PLACEMENT_3D('',#72228,#42432,#42433) ;
#34964=AXIS2_PLACEMENT_3D('',#72229,#42434,#42435) ;
#34965=AXIS2_PLACEMENT_3D('',#72230,#42436,#42437) ;
#34966=AXIS2_PLACEMENT_3D('',#72232,#42439,#42440) ;
#34967=AXIS2_PLACEMENT_3D('',#72233,#42441,#42442) ;
#34968=AXIS2_PLACEMENT_3D('',#72234,#42443,#42444) ;
#34969=AXIS2_PLACEMENT_3D('',#72235,#42445,#42446) ;
#34970=AXIS2_PLACEMENT_3D('',#72236,#42447,#42448) ;
#34971=AXIS2_PLACEMENT_3D('',#72237,#42449,#42450) ;
#34972=AXIS2_PLACEMENT_3D('',#72238,#42451,#42452) ;
#34973=AXIS2_PLACEMENT_3D('',#72239,#42453,#42454) ;
#34974=AXIS2_PLACEMENT_3D('',#72248,#42459,#42460) ;
#34975=AXIS2_PLACEMENT_3D('',#72250,#42461,#42462) ;
#34976=AXIS2_PLACEMENT_3D('',#72252,#42463,#42464) ;
#34977=AXIS2_PLACEMENT_3D('',#72253,#42465,#42466) ;
#34978=AXIS2_PLACEMENT_3D('',#72254,#42467,#42468) ;
#34979=AXIS2_PLACEMENT_3D('',#72256,#42469,#42470) ;
#34980=AXIS2_PLACEMENT_3D('',#72257,#42471,#42472) ;
#34981=AXIS2_PLACEMENT_3D('',#72258,#42473,#42474) ;
#34982=AXIS2_PLACEMENT_3D('',#72259,#42475,#42476) ;
#34983=AXIS2_PLACEMENT_3D('',#72261,#42478,#42479) ;
#34984=AXIS2_PLACEMENT_3D('',#72262,#42480,#42481) ;
#34985=AXIS2_PLACEMENT_3D('',#72263,#42482,#42483) ;
#34986=AXIS2_PLACEMENT_3D('',#72265,#42485,#42486) ;
#34987=AXIS2_PLACEMENT_3D('',#72266,#42487,#42488) ;
#34988=AXIS2_PLACEMENT_3D('',#72267,#42489,#42490) ;
#34989=AXIS2_PLACEMENT_3D('',#72268,#42491,#42492) ;
#34990=AXIS2_PLACEMENT_3D('',#72269,#42493,#42494) ;
#34991=AXIS2_PLACEMENT_3D('',#72270,#42495,#42496) ;
#34992=AXIS2_PLACEMENT_3D('',#72271,#42497,#42498) ;
#34993=AXIS2_PLACEMENT_3D('',#72272,#42499,#42500) ;
#34994=AXIS2_PLACEMENT_3D('',#72273,#42501,#42502) ;
#34995=AXIS2_PLACEMENT_3D('',#72276,#42503,#42504) ;
#34996=AXIS2_PLACEMENT_3D('',#72279,#42506,#42507) ;
#34997=AXIS2_PLACEMENT_3D('',#72281,#42509,#42510) ;
#34998=AXIS2_PLACEMENT_3D('',#72283,#42511,#42512) ;
#34999=AXIS2_PLACEMENT_3D('',#72284,#42513,#42514) ;
#35000=AXIS2_PLACEMENT_3D('',#72285,#42515,#42516) ;
#35001=AXIS2_PLACEMENT_3D('',#72287,#42517,#42518) ;
#35002=AXIS2_PLACEMENT_3D('',#72289,#42520,#42521) ;
#35003=AXIS2_PLACEMENT_3D('',#72291,#42522,#42523) ;
#35004=AXIS2_PLACEMENT_3D('',#72292,#42524,#42525) ;
#35005=AXIS2_PLACEMENT_3D('',#72293,#42526,#42527) ;
#35006=AXIS2_PLACEMENT_3D('',#72296,#42528,#42529) ;
#35007=AXIS2_PLACEMENT_3D('',#72297,#42530,#42531) ;
#35008=AXIS2_PLACEMENT_3D('',#72298,#42532,#42533) ;
#35009=AXIS2_PLACEMENT_3D('',#72299,#42534,#42535) ;
#35010=AXIS2_PLACEMENT_3D('',#72301,#42537,#42538) ;
#35011=AXIS2_PLACEMENT_3D('',#72302,#42539,#42540) ;
#35012=AXIS2_PLACEMENT_3D('',#72304,#42542,#42543) ;
#35013=AXIS2_PLACEMENT_3D('',#72306,#42544,#42545) ;
#35014=AXIS2_PLACEMENT_3D('',#72307,#42546,#42547) ;
#35015=AXIS2_PLACEMENT_3D('',#72308,#42548,#42549) ;
#35016=AXIS2_PLACEMENT_3D('',#72309,#42550,#42551) ;
#35017=AXIS2_PLACEMENT_3D('',#72311,#42553,#42554) ;
#35018=AXIS2_PLACEMENT_3D('',#72314,#42557,#42558) ;
#35019=AXIS2_PLACEMENT_3D('',#72316,#42559,#42560) ;
#35020=AXIS2_PLACEMENT_3D('',#72318,#42562,#42563) ;
#35021=AXIS2_PLACEMENT_3D('',#72320,#42565,#42566) ;
#35022=AXIS2_PLACEMENT_3D('',#72321,#42567,#42568) ;
#35023=AXIS2_PLACEMENT_3D('',#72322,#42569,#42570) ;
#35024=AXIS2_PLACEMENT_3D('',#72323,#42571,#42572) ;
#35025=AXIS2_PLACEMENT_3D('',#72324,#42573,#42574) ;
#35026=AXIS2_PLACEMENT_3D('',#72326,#42576,#42577) ;
#35027=AXIS2_PLACEMENT_3D('',#72327,#42578,#42579) ;
#35028=AXIS2_PLACEMENT_3D('',#72328,#42580,#42581) ;
#35029=AXIS2_PLACEMENT_3D('',#72329,#42582,#42583) ;
#35030=AXIS2_PLACEMENT_3D('',#72330,#42584,#42585) ;
#35031=AXIS2_PLACEMENT_3D('',#72331,#42586,#42587) ;
#35032=AXIS2_PLACEMENT_3D('',#72332,#42588,#42589) ;
#35033=AXIS2_PLACEMENT_3D('',#72333,#42590,#42591) ;
#35034=AXIS2_PLACEMENT_3D('',#72342,#42596,#42597) ;
#35035=AXIS2_PLACEMENT_3D('',#72344,#42598,#42599) ;
#35036=AXIS2_PLACEMENT_3D('',#72346,#42600,#42601) ;
#35037=AXIS2_PLACEMENT_3D('',#72347,#42602,#42603) ;
#35038=AXIS2_PLACEMENT_3D('',#72348,#42604,#42605) ;
#35039=AXIS2_PLACEMENT_3D('',#72350,#42606,#42607) ;
#35040=AXIS2_PLACEMENT_3D('',#72351,#42608,#42609) ;
#35041=AXIS2_PLACEMENT_3D('',#72352,#42610,#42611) ;
#35042=AXIS2_PLACEMENT_3D('',#72353,#42612,#42613) ;
#35043=AXIS2_PLACEMENT_3D('',#72355,#42615,#42616) ;
#35044=AXIS2_PLACEMENT_3D('',#72356,#42617,#42618) ;
#35045=AXIS2_PLACEMENT_3D('',#72357,#42619,#42620) ;
#35046=AXIS2_PLACEMENT_3D('',#72359,#42622,#42623) ;
#35047=AXIS2_PLACEMENT_3D('',#72360,#42624,#42625) ;
#35048=AXIS2_PLACEMENT_3D('',#72361,#42626,#42627) ;
#35049=AXIS2_PLACEMENT_3D('',#72362,#42628,#42629) ;
#35050=AXIS2_PLACEMENT_3D('',#72363,#42630,#42631) ;
#35051=AXIS2_PLACEMENT_3D('',#72364,#42632,#42633) ;
#35052=AXIS2_PLACEMENT_3D('',#72365,#42634,#42635) ;
#35053=AXIS2_PLACEMENT_3D('',#72366,#42636,#42637) ;
#35054=AXIS2_PLACEMENT_3D('',#72367,#42638,#42639) ;
#35055=AXIS2_PLACEMENT_3D('',#72370,#42640,#42641) ;
#35056=AXIS2_PLACEMENT_3D('',#72373,#42643,#42644) ;
#35057=AXIS2_PLACEMENT_3D('',#72375,#42646,#42647) ;
#35058=AXIS2_PLACEMENT_3D('',#72377,#42648,#42649) ;
#35059=AXIS2_PLACEMENT_3D('',#72378,#42650,#42651) ;
#35060=AXIS2_PLACEMENT_3D('',#72379,#42652,#42653) ;
#35061=AXIS2_PLACEMENT_3D('',#72381,#42654,#42655) ;
#35062=AXIS2_PLACEMENT_3D('',#72383,#42657,#42658) ;
#35063=AXIS2_PLACEMENT_3D('',#72385,#42659,#42660) ;
#35064=AXIS2_PLACEMENT_3D('',#72386,#42661,#42662) ;
#35065=AXIS2_PLACEMENT_3D('',#72387,#42663,#42664) ;
#35066=AXIS2_PLACEMENT_3D('',#72390,#42665,#42666) ;
#35067=AXIS2_PLACEMENT_3D('',#72391,#42667,#42668) ;
#35068=AXIS2_PLACEMENT_3D('',#72392,#42669,#42670) ;
#35069=AXIS2_PLACEMENT_3D('',#72393,#42671,#42672) ;
#35070=AXIS2_PLACEMENT_3D('',#72395,#42674,#42675) ;
#35071=AXIS2_PLACEMENT_3D('',#72396,#42676,#42677) ;
#35072=AXIS2_PLACEMENT_3D('',#72398,#42679,#42680) ;
#35073=AXIS2_PLACEMENT_3D('',#72400,#42681,#42682) ;
#35074=AXIS2_PLACEMENT_3D('',#72401,#42683,#42684) ;
#35075=AXIS2_PLACEMENT_3D('',#72402,#42685,#42686) ;
#35076=AXIS2_PLACEMENT_3D('',#72403,#42687,#42688) ;
#35077=AXIS2_PLACEMENT_3D('',#72405,#42690,#42691) ;
#35078=AXIS2_PLACEMENT_3D('',#72408,#42694,#42695) ;
#35079=AXIS2_PLACEMENT_3D('',#72410,#42696,#42697) ;
#35080=AXIS2_PLACEMENT_3D('',#72412,#42699,#42700) ;
#35081=AXIS2_PLACEMENT_3D('',#72414,#42702,#42703) ;
#35082=AXIS2_PLACEMENT_3D('',#72415,#42704,#42705) ;
#35083=AXIS2_PLACEMENT_3D('',#72416,#42706,#42707) ;
#35084=AXIS2_PLACEMENT_3D('',#72417,#42708,#42709) ;
#35085=AXIS2_PLACEMENT_3D('',#72418,#42710,#42711) ;
#35086=AXIS2_PLACEMENT_3D('',#72420,#42713,#42714) ;
#35087=AXIS2_PLACEMENT_3D('',#72421,#42715,#42716) ;
#35088=AXIS2_PLACEMENT_3D('',#72422,#42717,#42718) ;
#35089=AXIS2_PLACEMENT_3D('',#72423,#42719,#42720) ;
#35090=AXIS2_PLACEMENT_3D('',#72424,#42721,#42722) ;
#35091=AXIS2_PLACEMENT_3D('',#72425,#42723,#42724) ;
#35092=AXIS2_PLACEMENT_3D('',#72426,#42725,#42726) ;
#35093=AXIS2_PLACEMENT_3D('',#72427,#42727,#42728) ;
#35094=AXIS2_PLACEMENT_3D('',#72436,#42733,#42734) ;
#35095=AXIS2_PLACEMENT_3D('',#72438,#42735,#42736) ;
#35096=AXIS2_PLACEMENT_3D('',#72440,#42737,#42738) ;
#35097=AXIS2_PLACEMENT_3D('',#72441,#42739,#42740) ;
#35098=AXIS2_PLACEMENT_3D('',#72442,#42741,#42742) ;
#35099=AXIS2_PLACEMENT_3D('',#72444,#42743,#42744) ;
#35100=AXIS2_PLACEMENT_3D('',#72445,#42745,#42746) ;
#35101=AXIS2_PLACEMENT_3D('',#72446,#42747,#42748) ;
#35102=AXIS2_PLACEMENT_3D('',#72447,#42749,#42750) ;
#35103=AXIS2_PLACEMENT_3D('',#72449,#42752,#42753) ;
#35104=AXIS2_PLACEMENT_3D('',#72450,#42754,#42755) ;
#35105=AXIS2_PLACEMENT_3D('',#72451,#42756,#42757) ;
#35106=AXIS2_PLACEMENT_3D('',#72453,#42759,#42760) ;
#35107=AXIS2_PLACEMENT_3D('',#72454,#42761,#42762) ;
#35108=AXIS2_PLACEMENT_3D('',#72455,#42763,#42764) ;
#35109=AXIS2_PLACEMENT_3D('',#72456,#42765,#42766) ;
#35110=AXIS2_PLACEMENT_3D('',#72457,#42767,#42768) ;
#35111=AXIS2_PLACEMENT_3D('',#72458,#42769,#42770) ;
#35112=AXIS2_PLACEMENT_3D('',#72459,#42771,#42772) ;
#35113=AXIS2_PLACEMENT_3D('',#72460,#42773,#42774) ;
#35114=AXIS2_PLACEMENT_3D('',#72461,#42775,#42776) ;
#35115=AXIS2_PLACEMENT_3D('',#72464,#42777,#42778) ;
#35116=AXIS2_PLACEMENT_3D('',#72467,#42780,#42781) ;
#35117=AXIS2_PLACEMENT_3D('',#72469,#42783,#42784) ;
#35118=AXIS2_PLACEMENT_3D('',#72471,#42785,#42786) ;
#35119=AXIS2_PLACEMENT_3D('',#72472,#42787,#42788) ;
#35120=AXIS2_PLACEMENT_3D('',#72473,#42789,#42790) ;
#35121=AXIS2_PLACEMENT_3D('',#72475,#42791,#42792) ;
#35122=AXIS2_PLACEMENT_3D('',#72477,#42794,#42795) ;
#35123=AXIS2_PLACEMENT_3D('',#72479,#42796,#42797) ;
#35124=AXIS2_PLACEMENT_3D('',#72480,#42798,#42799) ;
#35125=AXIS2_PLACEMENT_3D('',#72481,#42800,#42801) ;
#35126=AXIS2_PLACEMENT_3D('',#72484,#42802,#42803) ;
#35127=AXIS2_PLACEMENT_3D('',#72485,#42804,#42805) ;
#35128=AXIS2_PLACEMENT_3D('',#72486,#42806,#42807) ;
#35129=AXIS2_PLACEMENT_3D('',#72487,#42808,#42809) ;
#35130=AXIS2_PLACEMENT_3D('',#72489,#42811,#42812) ;
#35131=AXIS2_PLACEMENT_3D('',#72490,#42813,#42814) ;
#35132=AXIS2_PLACEMENT_3D('',#72492,#42816,#42817) ;
#35133=AXIS2_PLACEMENT_3D('',#72494,#42818,#42819) ;
#35134=AXIS2_PLACEMENT_3D('',#72495,#42820,#42821) ;
#35135=AXIS2_PLACEMENT_3D('',#72496,#42822,#42823) ;
#35136=AXIS2_PLACEMENT_3D('',#72497,#42824,#42825) ;
#35137=AXIS2_PLACEMENT_3D('',#72499,#42827,#42828) ;
#35138=AXIS2_PLACEMENT_3D('',#72502,#42831,#42832) ;
#35139=AXIS2_PLACEMENT_3D('',#72504,#42833,#42834) ;
#35140=AXIS2_PLACEMENT_3D('',#72506,#42836,#42837) ;
#35141=AXIS2_PLACEMENT_3D('',#72508,#42839,#42840) ;
#35142=AXIS2_PLACEMENT_3D('',#72509,#42841,#42842) ;
#35143=AXIS2_PLACEMENT_3D('',#72510,#42843,#42844) ;
#35144=AXIS2_PLACEMENT_3D('',#72511,#42845,#42846) ;
#35145=AXIS2_PLACEMENT_3D('',#72512,#42847,#42848) ;
#35146=AXIS2_PLACEMENT_3D('',#72514,#42850,#42851) ;
#35147=AXIS2_PLACEMENT_3D('',#72515,#42852,#42853) ;
#35148=AXIS2_PLACEMENT_3D('',#72516,#42854,#42855) ;
#35149=AXIS2_PLACEMENT_3D('',#72517,#42856,#42857) ;
#35150=AXIS2_PLACEMENT_3D('',#72518,#42858,#42859) ;
#35151=AXIS2_PLACEMENT_3D('',#72519,#42860,#42861) ;
#35152=AXIS2_PLACEMENT_3D('',#72520,#42862,#42863) ;
#35153=AXIS2_PLACEMENT_3D('',#72521,#42864,#42865) ;
#35154=AXIS2_PLACEMENT_3D('',#72530,#42870,#42871) ;
#35155=AXIS2_PLACEMENT_3D('',#72532,#42872,#42873) ;
#35156=AXIS2_PLACEMENT_3D('',#72534,#42874,#42875) ;
#35157=AXIS2_PLACEMENT_3D('',#72535,#42876,#42877) ;
#35158=AXIS2_PLACEMENT_3D('',#72536,#42878,#42879) ;
#35159=AXIS2_PLACEMENT_3D('',#72538,#42880,#42881) ;
#35160=AXIS2_PLACEMENT_3D('',#72539,#42882,#42883) ;
#35161=AXIS2_PLACEMENT_3D('',#72540,#42884,#42885) ;
#35162=AXIS2_PLACEMENT_3D('',#72541,#42886,#42887) ;
#35163=AXIS2_PLACEMENT_3D('',#72543,#42889,#42890) ;
#35164=AXIS2_PLACEMENT_3D('',#72544,#42891,#42892) ;
#35165=AXIS2_PLACEMENT_3D('',#72545,#42893,#42894) ;
#35166=AXIS2_PLACEMENT_3D('',#72547,#42896,#42897) ;
#35167=AXIS2_PLACEMENT_3D('',#72548,#42898,#42899) ;
#35168=AXIS2_PLACEMENT_3D('',#72549,#42900,#42901) ;
#35169=AXIS2_PLACEMENT_3D('',#72550,#42902,#42903) ;
#35170=AXIS2_PLACEMENT_3D('',#72551,#42904,#42905) ;
#35171=AXIS2_PLACEMENT_3D('',#72552,#42906,#42907) ;
#35172=AXIS2_PLACEMENT_3D('',#72553,#42908,#42909) ;
#35173=AXIS2_PLACEMENT_3D('',#72554,#42910,#42911) ;
#35174=AXIS2_PLACEMENT_3D('',#72555,#42912,#42913) ;
#35175=AXIS2_PLACEMENT_3D('',#72558,#42914,#42915) ;
#35176=AXIS2_PLACEMENT_3D('',#72561,#42917,#42918) ;
#35177=AXIS2_PLACEMENT_3D('',#72563,#42920,#42921) ;
#35178=AXIS2_PLACEMENT_3D('',#72565,#42922,#42923) ;
#35179=AXIS2_PLACEMENT_3D('',#72566,#42924,#42925) ;
#35180=AXIS2_PLACEMENT_3D('',#72567,#42926,#42927) ;
#35181=AXIS2_PLACEMENT_3D('',#72569,#42928,#42929) ;
#35182=AXIS2_PLACEMENT_3D('',#72571,#42931,#42932) ;
#35183=AXIS2_PLACEMENT_3D('',#72573,#42933,#42934) ;
#35184=AXIS2_PLACEMENT_3D('',#72574,#42935,#42936) ;
#35185=AXIS2_PLACEMENT_3D('',#72575,#42937,#42938) ;
#35186=AXIS2_PLACEMENT_3D('',#72578,#42939,#42940) ;
#35187=AXIS2_PLACEMENT_3D('',#72579,#42941,#42942) ;
#35188=AXIS2_PLACEMENT_3D('',#72580,#42943,#42944) ;
#35189=AXIS2_PLACEMENT_3D('',#72581,#42945,#42946) ;
#35190=AXIS2_PLACEMENT_3D('',#72583,#42948,#42949) ;
#35191=AXIS2_PLACEMENT_3D('',#72584,#42950,#42951) ;
#35192=AXIS2_PLACEMENT_3D('',#72586,#42953,#42954) ;
#35193=AXIS2_PLACEMENT_3D('',#72588,#42955,#42956) ;
#35194=AXIS2_PLACEMENT_3D('',#72589,#42957,#42958) ;
#35195=AXIS2_PLACEMENT_3D('',#72590,#42959,#42960) ;
#35196=AXIS2_PLACEMENT_3D('',#72591,#42961,#42962) ;
#35197=AXIS2_PLACEMENT_3D('',#72593,#42964,#42965) ;
#35198=AXIS2_PLACEMENT_3D('',#72596,#42968,#42969) ;
#35199=AXIS2_PLACEMENT_3D('',#72598,#42970,#42971) ;
#35200=AXIS2_PLACEMENT_3D('',#72600,#42973,#42974) ;
#35201=AXIS2_PLACEMENT_3D('',#72602,#42976,#42977) ;
#35202=AXIS2_PLACEMENT_3D('',#72603,#42978,#42979) ;
#35203=AXIS2_PLACEMENT_3D('',#72604,#42980,#42981) ;
#35204=AXIS2_PLACEMENT_3D('',#72605,#42982,#42983) ;
#35205=AXIS2_PLACEMENT_3D('',#72606,#42984,#42985) ;
#35206=AXIS2_PLACEMENT_3D('',#72608,#42987,#42988) ;
#35207=AXIS2_PLACEMENT_3D('',#72609,#42989,#42990) ;
#35208=AXIS2_PLACEMENT_3D('',#72610,#42991,#42992) ;
#35209=AXIS2_PLACEMENT_3D('',#72611,#42993,#42994) ;
#35210=AXIS2_PLACEMENT_3D('',#72612,#42995,#42996) ;
#35211=AXIS2_PLACEMENT_3D('',#72613,#42997,#42998) ;
#35212=AXIS2_PLACEMENT_3D('',#72614,#42999,#43000) ;
#35213=AXIS2_PLACEMENT_3D('',#72615,#43001,#43002) ;
#35214=AXIS2_PLACEMENT_3D('',#72624,#43007,#43008) ;
#35215=AXIS2_PLACEMENT_3D('',#72626,#43009,#43010) ;
#35216=AXIS2_PLACEMENT_3D('',#72628,#43011,#43012) ;
#35217=AXIS2_PLACEMENT_3D('',#72629,#43013,#43014) ;
#35218=AXIS2_PLACEMENT_3D('',#72630,#43015,#43016) ;
#35219=AXIS2_PLACEMENT_3D('',#72632,#43017,#43018) ;
#35220=AXIS2_PLACEMENT_3D('',#72633,#43019,#43020) ;
#35221=AXIS2_PLACEMENT_3D('',#72634,#43021,#43022) ;
#35222=AXIS2_PLACEMENT_3D('',#72635,#43023,#43024) ;
#35223=AXIS2_PLACEMENT_3D('',#72637,#43026,#43027) ;
#35224=AXIS2_PLACEMENT_3D('',#72638,#43028,#43029) ;
#35225=AXIS2_PLACEMENT_3D('',#72639,#43030,#43031) ;
#35226=AXIS2_PLACEMENT_3D('',#72641,#43033,#43034) ;
#35227=AXIS2_PLACEMENT_3D('',#72642,#43035,#43036) ;
#35228=AXIS2_PLACEMENT_3D('',#72643,#43037,#43038) ;
#35229=AXIS2_PLACEMENT_3D('',#72644,#43039,#43040) ;
#35230=AXIS2_PLACEMENT_3D('',#72645,#43041,#43042) ;
#35231=AXIS2_PLACEMENT_3D('',#72646,#43043,#43044) ;
#35232=AXIS2_PLACEMENT_3D('',#72647,#43045,#43046) ;
#35233=AXIS2_PLACEMENT_3D('',#72650,#43049,#43050) ;
#35234=AXIS2_PLACEMENT_3D('',#72653,#43053,#43054) ;
#35235=AXIS2_PLACEMENT_3D('',#72656,#43057,#43058) ;
#35236=AXIS2_PLACEMENT_3D('',#72659,#43061,#43062) ;
#35237=AXIS2_PLACEMENT_3D('',#72662,#43065,#43066) ;
#35238=AXIS2_PLACEMENT_3D('',#72665,#43069,#43070) ;
#35239=AXIS2_PLACEMENT_3D('',#72668,#43073,#43074) ;
#35240=AXIS2_PLACEMENT_3D('',#72671,#43077,#43078) ;
#35241=AXIS2_PLACEMENT_3D('',#72674,#43081,#43082) ;
#35242=AXIS2_PLACEMENT_3D('',#72676,#43084,#43085) ;
#35243=AXIS2_PLACEMENT_3D('',#72678,#43087,#43088) ;
#35244=AXIS2_PLACEMENT_3D('',#72680,#43090,#43091) ;
#35245=AXIS2_PLACEMENT_3D('',#72682,#43093,#43094) ;
#35246=AXIS2_PLACEMENT_3D('',#72684,#43096,#43097) ;
#35247=AXIS2_PLACEMENT_3D('',#72686,#43099,#43100) ;
#35248=AXIS2_PLACEMENT_3D('',#72688,#43102,#43103) ;
#35249=AXIS2_PLACEMENT_3D('',#72690,#43105,#43106) ;
#35250=AXIS2_PLACEMENT_3D('',#72692,#43108,#43109) ;
#35251=AXIS2_PLACEMENT_3D('',#72694,#43111,#43112) ;
#35252=AXIS2_PLACEMENT_3D('',#72696,#43114,#43115) ;
#35253=AXIS2_PLACEMENT_3D('',#72698,#43117,#43118) ;
#35254=AXIS2_PLACEMENT_3D('',#72700,#43120,#43121) ;
#35255=AXIS2_PLACEMENT_3D('',#72702,#43123,#43124) ;
#35256=AXIS2_PLACEMENT_3D('',#72704,#43126,#43127) ;
#35257=AXIS2_PLACEMENT_3D('',#72706,#43129,#43130) ;
#35258=AXIS2_PLACEMENT_3D('',#72708,#43132,#43133) ;
#35259=AXIS2_PLACEMENT_3D('',#72710,#43135,#43136) ;
#35260=AXIS2_PLACEMENT_3D('',#72791,#43177,#43178) ;
#35261=AXIS2_PLACEMENT_3D('',#72793,#43179,#43180) ;
#35262=AXIS2_PLACEMENT_3D('',#72796,#43182,#43183) ;
#35263=AXIS2_PLACEMENT_3D('',#72797,#43184,#43185) ;
#35264=AXIS2_PLACEMENT_3D('',#72802,#43189,#43190) ;
#35265=AXIS2_PLACEMENT_3D('',#72806,#43192,#43193) ;
#35266=AXIS2_PLACEMENT_3D('',#72807,#43194,#43195) ;
#35267=AXIS2_PLACEMENT_3D('',#72808,#43196,#43197) ;
#35268=AXIS2_PLACEMENT_3D('',#72810,#43198,#43199) ;
#35269=AXIS2_PLACEMENT_3D('',#72813,#43201,#43202) ;
#35270=AXIS2_PLACEMENT_3D('',#72814,#43203,#43204) ;
#35271=AXIS2_PLACEMENT_3D('',#72816,#43205,#43206) ;
#35272=AXIS2_PLACEMENT_3D('',#72819,#43208,#43209) ;
#35273=AXIS2_PLACEMENT_3D('',#72820,#43210,#43211) ;
#35274=AXIS2_PLACEMENT_3D('',#72824,#43213,#43214) ;
#35275=AXIS2_PLACEMENT_3D('',#72825,#43215,#43216) ;
#35276=AXIS2_PLACEMENT_3D('',#72826,#43217,#43218) ;
#35277=AXIS2_PLACEMENT_3D('',#72830,#43220,#43221) ;
#35278=AXIS2_PLACEMENT_3D('',#72831,#43222,#43223) ;
#35279=AXIS2_PLACEMENT_3D('',#72832,#43224,#43225) ;
#35280=AXIS2_PLACEMENT_3D('',#72836,#43227,#43228) ;
#35281=AXIS2_PLACEMENT_3D('',#72837,#43229,#43230) ;
#35282=AXIS2_PLACEMENT_3D('',#72838,#43231,#43232) ;
#35283=AXIS2_PLACEMENT_3D('',#72840,#43233,#43234) ;
#35284=AXIS2_PLACEMENT_3D('',#72843,#43236,#43237) ;
#35285=AXIS2_PLACEMENT_3D('',#72844,#43238,#43239) ;
#35286=AXIS2_PLACEMENT_3D('',#72848,#43241,#43242) ;
#35287=AXIS2_PLACEMENT_3D('',#72849,#43243,#43244) ;
#35288=AXIS2_PLACEMENT_3D('',#72850,#43245,#43246) ;
#35289=AXIS2_PLACEMENT_3D('',#72852,#43247,#43248) ;
#35290=AXIS2_PLACEMENT_3D('',#72857,#43252,#43253) ;
#35291=AXIS2_PLACEMENT_3D('',#72860,#43255,#43256) ;
#35292=AXIS2_PLACEMENT_3D('',#72861,#43257,#43258) ;
#35293=AXIS2_PLACEMENT_3D('',#72863,#43260,#43261) ;
#35294=AXIS2_PLACEMENT_3D('',#72872,#43266,#43267) ;
#35295=AXIS2_PLACEMENT_3D('',#72881,#43272,#43273) ;
#35296=AXIS2_PLACEMENT_3D('',#72890,#43278,#43279) ;
#35297=AXIS2_PLACEMENT_3D('',#72899,#43284,#43285) ;
#35298=AXIS2_PLACEMENT_3D('',#72908,#43290,#43291) ;
#35299=AXIS2_PLACEMENT_3D('',#72917,#43296,#43297) ;
#35300=AXIS2_PLACEMENT_3D('',#72926,#43302,#43303) ;
#35301=AXIS2_PLACEMENT_3D('',#72935,#43308,#43309) ;
#35302=AXIS2_PLACEMENT_3D('',#72938,#43312,#43313) ;
#35303=AXIS2_PLACEMENT_3D('',#72943,#43317,#43318) ;
#35304=AXIS2_PLACEMENT_3D('',#72948,#43322,#43323) ;
#35305=AXIS2_PLACEMENT_3D('',#72953,#43327,#43328) ;
#35306=AXIS2_PLACEMENT_3D('',#72958,#43332,#43333) ;
#35307=AXIS2_PLACEMENT_3D('',#72963,#43337,#43338) ;
#35308=AXIS2_PLACEMENT_3D('',#72968,#43342,#43343) ;
#35309=AXIS2_PLACEMENT_3D('',#72973,#43347,#43348) ;
#35310=AXIS2_PLACEMENT_3D('',#72978,#43352,#43353) ;
#35311=AXIS2_PLACEMENT_3D('',#72983,#43357,#43358) ;
#35312=AXIS2_PLACEMENT_3D('',#72988,#43362,#43363) ;
#35313=AXIS2_PLACEMENT_3D('',#72993,#43367,#43368) ;
#35314=AXIS2_PLACEMENT_3D('',#72998,#43372,#43373) ;
#35315=AXIS2_PLACEMENT_3D('',#73003,#43377,#43378) ;
#35316=AXIS2_PLACEMENT_3D('',#73008,#43382,#43383) ;
#35317=AXIS2_PLACEMENT_3D('',#73013,#43387,#43388) ;
#35318=AXIS2_PLACEMENT_3D('',#73018,#43392,#43393) ;
#35319=AXIS2_PLACEMENT_3D('',#73019,#43394,#43395) ;
#35320=AXIS2_PLACEMENT_3D('',#73021,#43397,#43398) ;
#35321=AXIS2_PLACEMENT_3D('',#73023,#43400,#43401) ;
#35322=AXIS2_PLACEMENT_3D('',#73025,#43403,#43404) ;
#35323=AXIS2_PLACEMENT_3D('',#73027,#43406,#43407) ;
#35324=AXIS2_PLACEMENT_3D('',#73029,#43409,#43410) ;
#35325=AXIS2_PLACEMENT_3D('',#73031,#43412,#43413) ;
#35326=AXIS2_PLACEMENT_3D('',#73033,#43415,#43416) ;
#35327=AXIS2_PLACEMENT_3D('',#73035,#43418,#43419) ;
#35328=AXIS2_PLACEMENT_3D('',#73037,#43421,#43422) ;
#35329=AXIS2_PLACEMENT_3D('',#73039,#43423,#43424) ;
#35330=AXIS2_PLACEMENT_3D('',#73040,#43425,#43426) ;
#35331=AXIS2_PLACEMENT_3D('',#73043,#43427,#43428) ;
#35332=AXIS2_PLACEMENT_3D('',#73044,#43429,#43430) ;
#35333=AXIS2_PLACEMENT_3D('',#73045,#43431,#43432) ;
#35334=AXIS2_PLACEMENT_3D('',#73046,#43433,#43434) ;
#35335=AXIS2_PLACEMENT_3D('',#73048,#43435,#43436) ;
#35336=AXIS2_PLACEMENT_3D('',#73050,#43438,#43439) ;
#35337=AXIS2_PLACEMENT_3D('',#73051,#43440,#43441) ;
#35338=AXIS2_PLACEMENT_3D('',#73052,#43442,#43443) ;
#35339=AXIS2_PLACEMENT_3D('',#73054,#43445,#43446) ;
#35340=AXIS2_PLACEMENT_3D('',#73055,#43447,#43448) ;
#35341=AXIS2_PLACEMENT_3D('',#73057,#43449,#43450) ;
#35342=AXIS2_PLACEMENT_3D('',#73058,#43451,#43452) ;
#35343=AXIS2_PLACEMENT_3D('',#73061,#43453,#43454) ;
#35344=AXIS2_PLACEMENT_3D('',#73062,#43455,#43456) ;
#35345=AXIS2_PLACEMENT_3D('',#73063,#43457,#43458) ;
#35346=AXIS2_PLACEMENT_3D('',#73064,#43459,#43460) ;
#35347=AXIS2_PLACEMENT_3D('',#73066,#43461,#43462) ;
#35348=AXIS2_PLACEMENT_3D('',#73068,#43464,#43465) ;
#35349=AXIS2_PLACEMENT_3D('',#73069,#43466,#43467) ;
#35350=AXIS2_PLACEMENT_3D('',#73070,#43468,#43469) ;
#35351=AXIS2_PLACEMENT_3D('',#73072,#43471,#43472) ;
#35352=AXIS2_PLACEMENT_3D('',#73073,#43473,#43474) ;
#35353=AXIS2_PLACEMENT_3D('',#73075,#43475,#43476) ;
#35354=AXIS2_PLACEMENT_3D('',#73076,#43477,#43478) ;
#35355=AXIS2_PLACEMENT_3D('',#73079,#43479,#43480) ;
#35356=AXIS2_PLACEMENT_3D('',#73080,#43481,#43482) ;
#35357=AXIS2_PLACEMENT_3D('',#73081,#43483,#43484) ;
#35358=AXIS2_PLACEMENT_3D('',#73082,#43485,#43486) ;
#35359=AXIS2_PLACEMENT_3D('',#73084,#43487,#43488) ;
#35360=AXIS2_PLACEMENT_3D('',#73086,#43490,#43491) ;
#35361=AXIS2_PLACEMENT_3D('',#73087,#43492,#43493) ;
#35362=AXIS2_PLACEMENT_3D('',#73088,#43494,#43495) ;
#35363=AXIS2_PLACEMENT_3D('',#73090,#43497,#43498) ;
#35364=AXIS2_PLACEMENT_3D('',#73091,#43499,#43500) ;
#35365=AXIS2_PLACEMENT_3D('',#73093,#43501,#43502) ;
#35366=AXIS2_PLACEMENT_3D('',#73094,#43503,#43504) ;
#35367=AXIS2_PLACEMENT_3D('',#73097,#43505,#43506) ;
#35368=AXIS2_PLACEMENT_3D('',#73098,#43507,#43508) ;
#35369=AXIS2_PLACEMENT_3D('',#73099,#43509,#43510) ;
#35370=AXIS2_PLACEMENT_3D('',#73100,#43511,#43512) ;
#35371=AXIS2_PLACEMENT_3D('',#73102,#43513,#43514) ;
#35372=AXIS2_PLACEMENT_3D('',#73104,#43516,#43517) ;
#35373=AXIS2_PLACEMENT_3D('',#73105,#43518,#43519) ;
#35374=AXIS2_PLACEMENT_3D('',#73106,#43520,#43521) ;
#35375=AXIS2_PLACEMENT_3D('',#73108,#43523,#43524) ;
#35376=AXIS2_PLACEMENT_3D('',#73109,#43525,#43526) ;
#35377=AXIS2_PLACEMENT_3D('',#73111,#43527,#43528) ;
#35378=AXIS2_PLACEMENT_3D('',#73112,#43529,#43530) ;
#35379=AXIS2_PLACEMENT_3D('',#73115,#43531,#43532) ;
#35380=AXIS2_PLACEMENT_3D('',#73116,#43533,#43534) ;
#35381=AXIS2_PLACEMENT_3D('',#73117,#43535,#43536) ;
#35382=AXIS2_PLACEMENT_3D('',#73118,#43537,#43538) ;
#35383=AXIS2_PLACEMENT_3D('',#73120,#43539,#43540) ;
#35384=AXIS2_PLACEMENT_3D('',#73122,#43542,#43543) ;
#35385=AXIS2_PLACEMENT_3D('',#73123,#43544,#43545) ;
#35386=AXIS2_PLACEMENT_3D('',#73124,#43546,#43547) ;
#35387=AXIS2_PLACEMENT_3D('',#73126,#43549,#43550) ;
#35388=AXIS2_PLACEMENT_3D('',#73127,#43551,#43552) ;
#35389=AXIS2_PLACEMENT_3D('',#73129,#43553,#43554) ;
#35390=AXIS2_PLACEMENT_3D('',#73130,#43555,#43556) ;
#35391=AXIS2_PLACEMENT_3D('',#73133,#43557,#43558) ;
#35392=AXIS2_PLACEMENT_3D('',#73134,#43559,#43560) ;
#35393=AXIS2_PLACEMENT_3D('',#73135,#43561,#43562) ;
#35394=AXIS2_PLACEMENT_3D('',#73136,#43563,#43564) ;
#35395=AXIS2_PLACEMENT_3D('',#73138,#43565,#43566) ;
#35396=AXIS2_PLACEMENT_3D('',#73140,#43568,#43569) ;
#35397=AXIS2_PLACEMENT_3D('',#73141,#43570,#43571) ;
#35398=AXIS2_PLACEMENT_3D('',#73142,#43572,#43573) ;
#35399=AXIS2_PLACEMENT_3D('',#73144,#43575,#43576) ;
#35400=AXIS2_PLACEMENT_3D('',#73145,#43577,#43578) ;
#35401=AXIS2_PLACEMENT_3D('',#73147,#43579,#43580) ;
#35402=AXIS2_PLACEMENT_3D('',#73148,#43581,#43582) ;
#35403=AXIS2_PLACEMENT_3D('',#73151,#43583,#43584) ;
#35404=AXIS2_PLACEMENT_3D('',#73152,#43585,#43586) ;
#35405=AXIS2_PLACEMENT_3D('',#73153,#43587,#43588) ;
#35406=AXIS2_PLACEMENT_3D('',#73154,#43589,#43590) ;
#35407=AXIS2_PLACEMENT_3D('',#73156,#43591,#43592) ;
#35408=AXIS2_PLACEMENT_3D('',#73158,#43594,#43595) ;
#35409=AXIS2_PLACEMENT_3D('',#73159,#43596,#43597) ;
#35410=AXIS2_PLACEMENT_3D('',#73160,#43598,#43599) ;
#35411=AXIS2_PLACEMENT_3D('',#73162,#43601,#43602) ;
#35412=AXIS2_PLACEMENT_3D('',#73163,#43603,#43604) ;
#35413=AXIS2_PLACEMENT_3D('',#73165,#43605,#43606) ;
#35414=AXIS2_PLACEMENT_3D('',#73166,#43607,#43608) ;
#35415=AXIS2_PLACEMENT_3D('',#73169,#43609,#43610) ;
#35416=AXIS2_PLACEMENT_3D('',#73170,#43611,#43612) ;
#35417=AXIS2_PLACEMENT_3D('',#73171,#43613,#43614) ;
#35418=AXIS2_PLACEMENT_3D('',#73172,#43615,#43616) ;
#35419=AXIS2_PLACEMENT_3D('',#73174,#43617,#43618) ;
#35420=AXIS2_PLACEMENT_3D('',#73176,#43620,#43621) ;
#35421=AXIS2_PLACEMENT_3D('',#73177,#43622,#43623) ;
#35422=AXIS2_PLACEMENT_3D('',#73178,#43624,#43625) ;
#35423=AXIS2_PLACEMENT_3D('',#73180,#43627,#43628) ;
#35424=AXIS2_PLACEMENT_3D('',#73181,#43629,#43630) ;
#35425=AXIS2_PLACEMENT_3D('',#73184,#43631,#43632) ;
#35426=AXIS2_PLACEMENT_3D('',#73185,#43633,#43634) ;
#35427=AXIS2_PLACEMENT_3D('',#73186,#43635,#43636) ;
#35428=AXIS2_PLACEMENT_3D('',#73187,#43637,#43638) ;
#35429=AXIS2_PLACEMENT_3D('',#73189,#43639,#43640) ;
#35430=AXIS2_PLACEMENT_3D('',#73191,#43642,#43643) ;
#35431=AXIS2_PLACEMENT_3D('',#73192,#43644,#43645) ;
#35432=AXIS2_PLACEMENT_3D('',#73193,#43646,#43647) ;
#35433=AXIS2_PLACEMENT_3D('',#73195,#43649,#43650) ;
#35434=AXIS2_PLACEMENT_3D('',#73196,#43651,#43652) ;
#35435=AXIS2_PLACEMENT_3D('',#73198,#43654,#43655) ;
#35436=AXIS2_PLACEMENT_3D('',#73200,#43657,#43658) ;
#35437=AXIS2_PLACEMENT_3D('',#73202,#43660,#43661) ;
#35438=AXIS2_PLACEMENT_3D('',#73203,#43662,#43663) ;
#35439=AXIS2_PLACEMENT_3D('',#73204,#43664,#43665) ;
#35440=AXIS2_PLACEMENT_3D('',#73206,#43667,#43668) ;
#35441=AXIS2_PLACEMENT_3D('',#73208,#43670,#43671) ;
#35442=AXIS2_PLACEMENT_3D('',#73210,#43673,#43674) ;
#35443=AXIS2_PLACEMENT_3D('',#73211,#43675,#43676) ;
#35444=AXIS2_PLACEMENT_3D('',#73212,#43677,#43678) ;
#35445=AXIS2_PLACEMENT_3D('',#73214,#43680,#43681) ;
#35446=AXIS2_PLACEMENT_3D('',#73216,#43683,#43684) ;
#35447=AXIS2_PLACEMENT_3D('',#73218,#43686,#43687) ;
#35448=AXIS2_PLACEMENT_3D('',#73219,#43688,#43689) ;
#35449=AXIS2_PLACEMENT_3D('',#73220,#43690,#43691) ;
#35450=AXIS2_PLACEMENT_3D('',#73222,#43693,#43694) ;
#35451=AXIS2_PLACEMENT_3D('',#73224,#43696,#43697) ;
#35452=AXIS2_PLACEMENT_3D('',#73226,#43699,#43700) ;
#35453=AXIS2_PLACEMENT_3D('',#73227,#43701,#43702) ;
#35454=AXIS2_PLACEMENT_3D('',#73228,#43703,#43704) ;
#35455=AXIS2_PLACEMENT_3D('',#73230,#43706,#43707) ;
#35456=AXIS2_PLACEMENT_3D('',#73232,#43709,#43710) ;
#35457=AXIS2_PLACEMENT_3D('',#73234,#43712,#43713) ;
#35458=AXIS2_PLACEMENT_3D('',#73235,#43714,#43715) ;
#35459=AXIS2_PLACEMENT_3D('',#73236,#43716,#43717) ;
#35460=AXIS2_PLACEMENT_3D('',#73238,#43719,#43720) ;
#35461=AXIS2_PLACEMENT_3D('',#73240,#43722,#43723) ;
#35462=AXIS2_PLACEMENT_3D('',#73242,#43725,#43726) ;
#35463=AXIS2_PLACEMENT_3D('',#73243,#43727,#43728) ;
#35464=AXIS2_PLACEMENT_3D('',#73244,#43729,#43730) ;
#35465=AXIS2_PLACEMENT_3D('',#73246,#43732,#43733) ;
#35466=AXIS2_PLACEMENT_3D('',#73248,#43735,#43736) ;
#35467=AXIS2_PLACEMENT_3D('',#73250,#43738,#43739) ;
#35468=AXIS2_PLACEMENT_3D('',#73251,#43740,#43741) ;
#35469=AXIS2_PLACEMENT_3D('',#73252,#43742,#43743) ;
#35470=AXIS2_PLACEMENT_3D('',#73254,#43745,#43746) ;
#35471=AXIS2_PLACEMENT_3D('',#73256,#43748,#43749) ;
#35472=AXIS2_PLACEMENT_3D('',#73258,#43751,#43752) ;
#35473=AXIS2_PLACEMENT_3D('',#73259,#43753,#43754) ;
#39204=DIRECTION('axis',(0.,0.,1.)) ;
#39205=DIRECTION('refdir',(1.,0.,0.)) ;
#39206=DIRECTION('center_axis',(4.58892183511729E-14,-7.97041684978857E-27,
1.)) ;
#39207=DIRECTION('ref_axis',(-1.73688224296914E-13,-1.,1.14794370197489E-41)) ;
#39208=DIRECTION('',(-1.73688224296914E-13,-1.,0.)) ;
#39209=DIRECTION('',(1.,-1.6579330501069E-13,-4.58892183511729E-14)) ;
#39210=DIRECTION('',(-1.73688224296914E-13,-1.,3.58732406867123E-43)) ;
#39211=DIRECTION('',(1.,-1.6579330501069E-13,-4.58892183511729E-14)) ;
#39212=DIRECTION('center_axis',(1.6579330501069E-13,1.,3.5839606558192E-28)) ;
#39213=DIRECTION('ref_axis',(4.53957858957841E-14,-7.88471344280163E-27,
1.)) ;
#39214=DIRECTION('',(4.53957858957841E-14,-7.88471344280162E-27,1.)) ;
#39215=DIRECTION('',(-1.,1.6579330501069E-13,4.54195640846217E-14)) ;
#39216=DIRECTION('',(4.53957858957841E-14,-7.88471344280162E-27,1.)) ;
#39217=DIRECTION('center_axis',(-1.6579330501069E-13,-1.,-3.43824445941423E-28)) ;
#39218=DIRECTION('ref_axis',(-4.35500900612589E-14,7.56413781071074E-27,
-1.)) ;
#39219=DIRECTION('',(-4.53957858957841E-14,7.87014182316113E-27,-1.)) ;
#39220=DIRECTION('',(-4.35500900612589E-14,7.56413781071072E-27,-1.)) ;
#39221=DIRECTION('',(1.,-1.6579330501069E-13,-4.54195640846217E-14)) ;
#39222=DIRECTION('center_axis',(1.,-1.6579330501069E-13,-4.58892183511729E-14)) ;
#39223=DIRECTION('ref_axis',(-4.58892183511729E-14,-2.00890147845606E-41,
-1.)) ;
#39224=DIRECTION('',(1.6579330501069E-13,1.,1.66321791207071E-16)) ;
#39225=DIRECTION('center_axis',(4.58892183511729E-14,-7.97041684978857E-27,
1.)) ;
#39226=DIRECTION('ref_axis',(-1.73688224296914E-13,-1.,1.14794370197489E-41)) ;
#39227=DIRECTION('',(-1.73688224296914E-13,-1.,0.)) ;
#39228=DIRECTION('',(1.,-1.6579330501069E-13,-4.58892183511729E-14)) ;
#39229=DIRECTION('',(-1.73688224296914E-13,-1.,3.58732406867123E-43)) ;
#39230=DIRECTION('',(1.,-1.6579330501069E-13,-4.58892183511729E-14)) ;
#39231=DIRECTION('center_axis',(1.6579330501069E-13,1.,3.5839606558192E-28)) ;
#39232=DIRECTION('ref_axis',(4.53957858957841E-14,-7.88471344280163E-27,
1.)) ;
#39233=DIRECTION('',(4.53957858957841E-14,-7.88471344280162E-27,1.)) ;
#39234=DIRECTION('',(-1.,1.6579330501069E-13,4.54195640846217E-14)) ;
#39235=DIRECTION('',(4.53957858957841E-14,-7.88471344280162E-27,1.)) ;
#39236=DIRECTION('center_axis',(-1.6579330501069E-13,-1.,-3.43824445941423E-28)) ;
#39237=DIRECTION('ref_axis',(-4.35500900612589E-14,7.56413781071074E-27,
-1.)) ;
#39238=DIRECTION('',(-4.53957858957841E-14,7.87014182316113E-27,-1.)) ;
#39239=DIRECTION('',(-4.35500900612589E-14,7.56413781071072E-27,-1.)) ;
#39240=DIRECTION('',(1.,-1.6579330501069E-13,-4.54195640846217E-14)) ;
#39241=DIRECTION('center_axis',(1.,-1.6579330501069E-13,-4.58892183511729E-14)) ;
#39242=DIRECTION('ref_axis',(-4.58892183511729E-14,-2.00890147845606E-41,
-1.)) ;
#39243=DIRECTION('',(1.6579330501069E-13,1.,1.66321791207071E-16)) ;
#39244=DIRECTION('center_axis',(-1.6579330501069E-13,-1.,-3.43824445941423E-28)) ;
#39245=DIRECTION('ref_axis',(-4.35500900612589E-14,7.56413781071074E-27,
-1.)) ;
#39246=DIRECTION('',(-4.53957858957841E-14,7.87014182316113E-27,-1.)) ;
#39247=DIRECTION('',(1.,-1.6579330501069E-13,-4.4408920985006E-14)) ;
#39248=DIRECTION('',(-4.35500900612589E-14,7.56413781071072E-27,-1.)) ;
#39249=DIRECTION('',(1.,-1.6579330501069E-13,-4.54195640846217E-14)) ;
#39250=DIRECTION('center_axis',(4.4408920985006E-14,-7.71330662882764E-27,
1.)) ;
#39251=DIRECTION('ref_axis',(-1.73688224296914E-13,-1.,1.29143666472175E-41)) ;
#39252=DIRECTION('',(-1.73688224296914E-13,-1.,1.43492962746861E-42)) ;
#39253=DIRECTION('',(1.,-1.6579330501069E-13,-4.4408920985006E-14)) ;
#39254=DIRECTION('',(-1.73688224296914E-13,-1.,3.58732406867123E-43)) ;
#39255=DIRECTION('center_axis',(1.6579330501069E-13,1.,3.5839606558192E-28)) ;
#39256=DIRECTION('ref_axis',(4.53957858957841E-14,-7.88471344280163E-27,
1.)) ;
#39257=DIRECTION('',(4.53957858957841E-14,-7.88471344280162E-27,1.)) ;
#39258=DIRECTION('',(-1.,1.6579330501069E-13,4.54195640846217E-14)) ;
#39259=DIRECTION('',(4.53957858957841E-14,-7.88471344280162E-27,1.)) ;
#39260=DIRECTION('center_axis',(1.,-1.6579330501069E-13,-4.4408920985006E-14)) ;
#39261=DIRECTION('ref_axis',(-4.4408920985006E-14,-2.00890147845606E-41,
-1.)) ;
#39262=DIRECTION('',(1.6579330501069E-13,1.,1.66321791207071E-16)) ;
#39263=DIRECTION('center_axis',(4.58892183511729E-14,-7.97041684978857E-27,
1.)) ;
#39264=DIRECTION('ref_axis',(-1.73688224296914E-13,-1.,1.14794370197489E-41)) ;
#39265=DIRECTION('',(-1.73688224296914E-13,-1.,0.)) ;
#39266=DIRECTION('',(1.,-1.6579330501069E-13,-4.58892183511729E-14)) ;
#39267=DIRECTION('',(-1.73688224296914E-13,-1.,3.58732406867123E-43)) ;
#39268=DIRECTION('',(1.,-1.6579330501069E-13,-4.58892183511729E-14)) ;
#39269=DIRECTION('center_axis',(1.6579330501069E-13,1.,3.5839606558192E-28)) ;
#39270=DIRECTION('ref_axis',(4.53957858957841E-14,-7.88471344280163E-27,
1.)) ;
#39271=DIRECTION('',(4.53957858957841E-14,-7.88471344280162E-27,1.)) ;
#39272=DIRECTION('',(-1.,1.6579330501069E-13,4.54195640846217E-14)) ;
#39273=DIRECTION('',(4.53957858957841E-14,-7.88471344280162E-27,1.)) ;
#39274=DIRECTION('center_axis',(-1.6579330501069E-13,-1.,-3.43824445941423E-28)) ;
#39275=DIRECTION('ref_axis',(-4.35500900612589E-14,7.56413781071074E-27,
-1.)) ;
#39276=DIRECTION('',(-4.53957858957841E-14,7.87014182316113E-27,-1.)) ;
#39277=DIRECTION('',(-4.35500900612589E-14,7.56413781071072E-27,-1.)) ;
#39278=DIRECTION('',(1.,-1.6579330501069E-13,-4.54195640846217E-14)) ;
#39279=DIRECTION('center_axis',(1.,-1.6579330501069E-13,-4.58892183511729E-14)) ;
#39280=DIRECTION('ref_axis',(-4.58892183511729E-14,-2.00890147845606E-41,
-1.)) ;
#39281=DIRECTION('',(1.6579330501069E-13,1.,1.66321791207071E-16)) ;
#39282=DIRECTION('center_axis',(4.58892183511729E-14,-7.97041684978857E-27,
1.)) ;
#39283=DIRECTION('ref_axis',(-1.73688224296914E-13,-1.,1.14794370197489E-41)) ;
#39284=DIRECTION('',(-1.73688224296914E-13,-1.,0.)) ;
#39285=DIRECTION('',(1.,-1.6579330501069E-13,-4.58892183511729E-14)) ;
#39286=DIRECTION('',(-1.73688224296914E-13,-1.,3.58732406867123E-43)) ;
#39287=DIRECTION('',(1.,-1.6579330501069E-13,-4.58892183511729E-14)) ;
#39288=DIRECTION('center_axis',(1.6579330501069E-13,1.,3.5839606558192E-28)) ;
#39289=DIRECTION('ref_axis',(4.53957858957841E-14,-7.88471344280163E-27,
1.)) ;
#39290=DIRECTION('',(4.53957858957841E-14,-7.88471344280162E-27,1.)) ;
#39291=DIRECTION('',(-1.,1.6579330501069E-13,4.54195640846217E-14)) ;
#39292=DIRECTION('',(4.53957858957841E-14,-7.88471344280162E-27,1.)) ;
#39293=DIRECTION('center_axis',(-1.6579330501069E-13,-1.,-3.43824445941423E-28)) ;
#39294=DIRECTION('ref_axis',(-4.35500900612589E-14,7.56413781071074E-27,
-1.)) ;
#39295=DIRECTION('',(-4.53957858957841E-14,7.87014182316113E-27,-1.)) ;
#39296=DIRECTION('',(-4.35500900612589E-14,7.56413781071072E-27,-1.)) ;
#39297=DIRECTION('',(1.,-1.6579330501069E-13,-4.54195640846217E-14)) ;
#39298=DIRECTION('center_axis',(1.,-1.6579330501069E-13,-4.58892183511729E-14)) ;
#39299=DIRECTION('ref_axis',(-4.58892183511729E-14,-2.00890147845606E-41,
-1.)) ;
#39300=DIRECTION('',(1.6579330501069E-13,1.,1.66321791207071E-16)) ;
#39301=DIRECTION('center_axis',(4.58892183511729E-14,-7.97041684978857E-27,
1.)) ;
#39302=DIRECTION('ref_axis',(-1.73688224296914E-13,-1.,1.14794370197489E-41)) ;
#39303=DIRECTION('',(-1.73688224296914E-13,-1.,0.)) ;
#39304=DIRECTION('',(1.,-1.6579330501069E-13,-4.58892183511729E-14)) ;
#39305=DIRECTION('',(-1.73688224296914E-13,-1.,3.58732406867123E-43)) ;
#39306=DIRECTION('',(1.,-1.6579330501069E-13,-4.58892183511729E-14)) ;
#39307=DIRECTION('center_axis',(1.6579330501069E-13,1.,3.5839606558192E-28)) ;
#39308=DIRECTION('ref_axis',(4.53957858957841E-14,-7.88471344280163E-27,
1.)) ;
#39309=DIRECTION('',(4.53957858957841E-14,-7.88471344280162E-27,1.)) ;
#39310=DIRECTION('',(-1.,1.6579330501069E-13,4.54195640846217E-14)) ;
#39311=DIRECTION('',(4.53957858957841E-14,-7.88471344280162E-27,1.)) ;
#39312=DIRECTION('center_axis',(-1.6579330501069E-13,-1.,-3.43824445941423E-28)) ;
#39313=DIRECTION('ref_axis',(-4.35500900612589E-14,7.56413781071074E-27,
-1.)) ;
#39314=DIRECTION('',(-4.53957858957841E-14,7.87014182316113E-27,-1.)) ;
#39315=DIRECTION('',(-4.35500900612589E-14,7.56413781071072E-27,-1.)) ;
#39316=DIRECTION('',(1.,-1.6579330501069E-13,-4.54195640846217E-14)) ;
#39317=DIRECTION('center_axis',(1.,-1.6579330501069E-13,-4.58892183511729E-14)) ;
#39318=DIRECTION('ref_axis',(-4.58892183511729E-14,-2.00890147845606E-41,
-1.)) ;
#39319=DIRECTION('',(1.6579330501069E-13,1.,1.66321791207071E-16)) ;
#39320=DIRECTION('center_axis',(-1.6579330501069E-13,-1.,-3.43824445941423E-28)) ;
#39321=DIRECTION('ref_axis',(-4.35500900612589E-14,7.56413781071074E-27,
-1.)) ;
#39322=DIRECTION('',(-4.53957858957841E-14,7.87014182316113E-27,-1.)) ;
#39323=DIRECTION('',(1.,-1.6579330501069E-13,-4.4408920985006E-14)) ;
#39324=DIRECTION('',(-4.35500900612589E-14,7.56413781071072E-27,-1.)) ;
#39325=DIRECTION('',(1.,-1.6579330501069E-13,-4.54195640846217E-14)) ;
#39326=DIRECTION('center_axis',(4.4408920985006E-14,-7.71330662882764E-27,
1.)) ;
#39327=DIRECTION('ref_axis',(-1.73688224296914E-13,-1.,1.29143666472175E-41)) ;
#39328=DIRECTION('',(-1.73688224296914E-13,-1.,1.43492962746861E-42)) ;
#39329=DIRECTION('',(1.,-1.6579330501069E-13,-4.4408920985006E-14)) ;
#39330=DIRECTION('',(-1.73688224296914E-13,-1.,3.58732406867123E-43)) ;
#39331=DIRECTION('center_axis',(1.6579330501069E-13,1.,3.5839606558192E-28)) ;
#39332=DIRECTION('ref_axis',(4.53957858957841E-14,-7.88471344280163E-27,
1.)) ;
#39333=DIRECTION('',(4.53957858957841E-14,-7.88471344280162E-27,1.)) ;
#39334=DIRECTION('',(-1.,1.6579330501069E-13,4.54195640846217E-14)) ;
#39335=DIRECTION('',(4.53957858957841E-14,-7.88471344280162E-27,1.)) ;
#39336=DIRECTION('center_axis',(1.,-1.6579330501069E-13,-4.4408920985006E-14)) ;
#39337=DIRECTION('ref_axis',(-4.4408920985006E-14,-2.00890147845606E-41,
-1.)) ;
#39338=DIRECTION('',(1.6579330501069E-13,1.,1.66321791207071E-16)) ;
#39339=DIRECTION('center_axis',(4.58892183511729E-14,-7.97041684978857E-27,
1.)) ;
#39340=DIRECTION('ref_axis',(-1.73688224296914E-13,-1.,1.14794370197489E-41)) ;
#39341=DIRECTION('',(-1.73688224296914E-13,-1.,0.)) ;
#39342=DIRECTION('',(1.,-1.6579330501069E-13,-4.58892183511729E-14)) ;
#39343=DIRECTION('',(-1.73688224296914E-13,-1.,3.58732406867123E-43)) ;
#39344=DIRECTION('',(1.,-1.6579330501069E-13,-4.58892183511729E-14)) ;
#39345=DIRECTION('center_axis',(1.6579330501069E-13,1.,3.5839606558192E-28)) ;
#39346=DIRECTION('ref_axis',(4.53957858957841E-14,-7.88471344280163E-27,
1.)) ;
#39347=DIRECTION('',(4.53957858957841E-14,-7.88471344280162E-27,1.)) ;
#39348=DIRECTION('',(-1.,1.6579330501069E-13,4.54195640846217E-14)) ;
#39349=DIRECTION('',(4.53957858957841E-14,-7.88471344280162E-27,1.)) ;
#39350=DIRECTION('center_axis',(-1.6579330501069E-13,-1.,-3.43824445941423E-28)) ;
#39351=DIRECTION('ref_axis',(-4.35500900612589E-14,7.56413781071074E-27,
-1.)) ;
#39352=DIRECTION('',(-4.53957858957841E-14,7.87014182316113E-27,-1.)) ;
#39353=DIRECTION('',(-4.35500900612589E-14,7.56413781071072E-27,-1.)) ;
#39354=DIRECTION('',(1.,-1.6579330501069E-13,-4.54195640846217E-14)) ;
#39355=DIRECTION('center_axis',(1.,-1.6579330501069E-13,-4.58892183511729E-14)) ;
#39356=DIRECTION('ref_axis',(-4.58892183511729E-14,-2.00890147845606E-41,
-1.)) ;
#39357=DIRECTION('',(1.6579330501069E-13,1.,1.66321791207071E-16)) ;
#39358=DIRECTION('center_axis',(4.58892183511729E-14,-7.97041684978857E-27,
1.)) ;
#39359=DIRECTION('ref_axis',(-1.73688224296914E-13,-1.,1.14794370197489E-41)) ;
#39360=DIRECTION('',(-1.73688224296914E-13,-1.,0.)) ;
#39361=DIRECTION('',(1.,-1.6579330501069E-13,-4.58892183511729E-14)) ;
#39362=DIRECTION('',(-1.73688224296914E-13,-1.,3.58732406867123E-43)) ;
#39363=DIRECTION('',(1.,-1.6579330501069E-13,-4.58892183511729E-14)) ;
#39364=DIRECTION('center_axis',(1.6579330501069E-13,1.,3.5839606558192E-28)) ;
#39365=DIRECTION('ref_axis',(4.53957858957841E-14,-7.88471344280163E-27,
1.)) ;
#39366=DIRECTION('',(4.53957858957841E-14,-7.88471344280162E-27,1.)) ;
#39367=DIRECTION('',(-1.,1.6579330501069E-13,4.54195640846217E-14)) ;
#39368=DIRECTION('',(4.53957858957841E-14,-7.88471344280162E-27,1.)) ;
#39369=DIRECTION('center_axis',(-1.6579330501069E-13,-1.,-3.43824445941423E-28)) ;
#39370=DIRECTION('ref_axis',(-4.35500900612589E-14,7.56413781071074E-27,
-1.)) ;
#39371=DIRECTION('',(-4.53957858957841E-14,7.87014182316113E-27,-1.)) ;
#39372=DIRECTION('',(-4.35500900612589E-14,7.56413781071072E-27,-1.)) ;
#39373=DIRECTION('',(1.,-1.6579330501069E-13,-4.54195640846217E-14)) ;
#39374=DIRECTION('center_axis',(1.,-1.6579330501069E-13,-4.58892183511729E-14)) ;
#39375=DIRECTION('ref_axis',(-4.58892183511729E-14,-2.00890147845606E-41,
-1.)) ;
#39376=DIRECTION('',(1.6579330501069E-13,1.,1.66321791207071E-16)) ;
#39377=DIRECTION('center_axis',(-4.54195640846217E-14,1.66321791214601E-16,
-1.)) ;
#39378=DIRECTION('ref_axis',(-1.,1.75658099177411E-13,4.54195640846217E-14)) ;
#39379=DIRECTION('',(-1.75658099177411E-13,-1.,-6.12002098060108E-16)) ;
#39380=DIRECTION('',(-1.75658099177411E-13,-1.,-6.12002098060108E-16)) ;
#39381=DIRECTION('',(-1.75658099177411E-13,-1.,-6.12002098060108E-16)) ;
#39382=DIRECTION('',(-1.75658099177411E-13,-1.,-6.12002098060108E-16)) ;
#39383=DIRECTION('',(-1.75658099177411E-13,-1.,-6.12002098060108E-16)) ;
#39384=DIRECTION('',(-1.75658099177411E-13,-1.,-6.12002098060108E-16)) ;
#39385=DIRECTION('',(-1.75658099177411E-13,-1.,-6.12002098060108E-16)) ;
#39386=DIRECTION('',(-1.,1.75658099177411E-13,4.54195640846217E-14)) ;
#39387=DIRECTION('',(-1.75658099177411E-13,-1.,-1.66321791206623E-16)) ;
#39388=DIRECTION('',(-1.,1.75658099177411E-13,4.54195640846217E-14)) ;
#39389=DIRECTION('',(-1.75658099177411E-13,-1.,-6.12002098060108E-16)) ;
#39390=DIRECTION('',(1.,-1.75658099177411E-13,-4.54195640846217E-14)) ;
#39391=DIRECTION('',(-1.75658099177411E-13,-1.,-1.66321791206623E-16)) ;
#39392=DIRECTION('',(-1.,1.75658099177411E-13,4.54195640846217E-14)) ;
#39393=DIRECTION('',(-1.75658099177411E-13,-1.,-6.12002098060108E-16)) ;
#39394=DIRECTION('',(1.,-1.75658099177411E-13,-4.54195640846217E-14)) ;
#39395=DIRECTION('',(-1.75658099177411E-13,-1.,-1.66321791206623E-16)) ;
#39396=DIRECTION('',(-1.,1.75658099177411E-13,4.54195640846217E-14)) ;
#39397=DIRECTION('',(-1.75658099177411E-13,-1.,-6.12002098060108E-16)) ;
#39398=DIRECTION('',(1.,-1.75658099177411E-13,-4.54195640846217E-14)) ;
#39399=DIRECTION('',(-1.75658099177411E-13,-1.,-1.66321791206623E-16)) ;
#39400=DIRECTION('',(-1.,1.75658099177411E-13,4.54195640846217E-14)) ;
#39401=DIRECTION('',(-1.75658099177411E-13,-1.,-6.12002098060108E-16)) ;
#39402=DIRECTION('',(1.,-1.75658099177411E-13,-4.54195640846217E-14)) ;
#39403=DIRECTION('',(-1.75658099177411E-13,-1.,-1.66321791206623E-16)) ;
#39404=DIRECTION('',(-1.,1.75658099177411E-13,4.54195640846217E-14)) ;
#39405=DIRECTION('',(-1.75658099177411E-13,-1.,-6.12002098060108E-16)) ;
#39406=DIRECTION('',(1.,-1.75658099177411E-13,-4.54195640846217E-14)) ;
#39407=DIRECTION('',(-1.75658099177411E-13,-1.,-1.66321791206623E-16)) ;
#39408=DIRECTION('',(-1.,1.75658099177411E-13,4.54195640846217E-14)) ;
#39409=DIRECTION('',(-1.75658099177411E-13,-1.,-6.12002098060108E-16)) ;
#39410=DIRECTION('',(1.,-1.75658099177411E-13,-4.54195640846217E-14)) ;
#39411=DIRECTION('',(-1.75658099177411E-13,-1.,-1.66321791206623E-16)) ;
#39412=DIRECTION('',(-1.,1.75658099177411E-13,4.54195640846217E-14)) ;
#39413=DIRECTION('',(-1.75658099177411E-13,-1.,-6.12002098060108E-16)) ;
#39414=DIRECTION('',(1.,-1.75658099177411E-13,-4.54195640846217E-14)) ;
#39415=DIRECTION('',(-1.75658099177411E-13,-1.,-1.66321791206623E-16)) ;
#39416=DIRECTION('',(-1.,1.75658099177411E-13,4.54195640846217E-14)) ;
#39417=DIRECTION('',(-1.75658099177411E-13,-1.,-6.12002098060108E-16)) ;
#39418=DIRECTION('',(1.,-1.75658099177411E-13,-4.54195640846217E-14)) ;
#39419=DIRECTION('',(-1.75658099177411E-13,-1.,-1.66321791206623E-16)) ;
#39420=DIRECTION('',(-1.,1.75658099177411E-13,4.54195640846217E-14)) ;
#39421=DIRECTION('',(-1.75658099177411E-13,-1.,-6.12002098060108E-16)) ;
#39422=DIRECTION('',(1.,-1.75658099177411E-13,-4.54195640846217E-14)) ;
#39423=DIRECTION('',(-1.75658099177411E-13,-1.,-1.66321791206623E-16)) ;
#39424=DIRECTION('',(-1.,1.73688224296914E-13,4.53957858957841E-14)) ;
#39425=DIRECTION('',(-1.75658099177411E-13,-1.,-6.12002098060108E-16)) ;
#39426=DIRECTION('',(-1.75658099177411E-13,-1.,-6.12002098060108E-16)) ;
#39427=DIRECTION('',(-1.75658099177411E-13,-1.,-6.12002098060108E-16)) ;
#39428=DIRECTION('center_axis',(-4.54195640846217E-14,1.66321791214601E-16,
-1.)) ;
#39429=DIRECTION('ref_axis',(-1.,0.,4.46626862477777E-14)) ;
#39430=DIRECTION('center_axis',(4.54195640846217E-14,-1.66321791214601E-16,
1.)) ;
#39431=DIRECTION('ref_axis',(-1.,1.8946420272009E-13,4.54195640846217E-14)) ;
#39432=DIRECTION('center_axis',(-7.59720474939486E-30,-1.,-1.66321791214601E-16)) ;
#39433=DIRECTION('ref_axis',(1.,0.,-4.56777472988634E-14)) ;
#39434=DIRECTION('center_axis',(-4.54195640846217E-14,1.66321791214601E-16,
-1.)) ;
#39435=DIRECTION('ref_axis',(-1.,1.8946420272009E-13,4.54195640846217E-14)) ;
#39436=DIRECTION('center_axis',(-4.54195640846217E-14,1.66321791214601E-16,
-1.)) ;
#39437=DIRECTION('ref_axis',(-1.,1.75658099177411E-13,4.54195640846217E-14)) ;
#39438=DIRECTION('center_axis',(-2.1716102378779E-15,3.83815143260386E-28,
1.)) ;
#39439=DIRECTION('ref_axis',(-1.,1.75658099177411E-13,-2.1716102378779E-15)) ;
#39440=DIRECTION('',(-4.54195640846217E-14,1.66321791214601E-16,-1.)) ;
#39441=DIRECTION('center_axis',(-4.54195640846217E-14,1.66321791214601E-16,
-1.)) ;
#39442=DIRECTION('ref_axis',(-1.,5.55236256206829E-46,4.54195640846217E-14)) ;
#39443=DIRECTION('',(1.75658099177411E-13,1.,1.66321791206623E-16)) ;
#39444=DIRECTION('',(1.,-1.75658099177411E-13,-4.54195640846217E-14)) ;
#39445=DIRECTION('',(-1.75658099177411E-13,-1.,-1.66321791206623E-16)) ;
#39446=DIRECTION('',(-1.,1.75658099177411E-13,4.54195640846217E-14)) ;
#39447=DIRECTION('',(-1.,3.33066907386739E-16,4.54195640846217E-14)) ;
#39448=DIRECTION('center_axis',(-4.54195640846217E-14,1.66321791214601E-16,
-1.)) ;
#39449=DIRECTION('ref_axis',(1.,-5.55236256206829E-46,-4.54195640846217E-14)) ;
#39450=DIRECTION('',(-8.32667268460786E-17,-1.,-1.66321791214597E-16)) ;
#39451=DIRECTION('center_axis',(-4.54195640846217E-14,1.66321791214601E-16,
-1.)) ;
#39452=DIRECTION('ref_axis',(1.,-5.55236256206829E-46,-4.54195640846217E-14)) ;
#39453=DIRECTION('',(1.,-3.33066907386739E-16,-4.54195640846217E-14)) ;
#39454=DIRECTION('center_axis',(-4.54195640846217E-14,1.66321791214601E-16,
-1.)) ;
#39455=DIRECTION('ref_axis',(1.,-5.55236256206829E-46,-4.54195640846217E-14)) ;
#39456=DIRECTION('',(1.66533453692965E-16,1.,1.66321791214593E-16)) ;
#39457=DIRECTION('center_axis',(-4.54195640846217E-14,1.66321791214601E-16,
-1.)) ;
#39458=DIRECTION('ref_axis',(1.,-5.55236256206829E-46,-4.54195640846217E-14)) ;
#39459=DIRECTION('center_axis',(-4.54195640846217E-14,1.66321791214601E-16,
-1.)) ;
#39460=DIRECTION('ref_axis',(-1.,0.,4.46626862477777E-14)) ;
#39461=DIRECTION('center_axis',(4.54195640846217E-14,-1.66321791214601E-16,
1.)) ;
#39462=DIRECTION('ref_axis',(-1.,1.8946420272009E-13,4.54195640846217E-14)) ;
#39463=DIRECTION('center_axis',(-7.59720474939486E-30,-1.,-1.66321791214601E-16)) ;
#39464=DIRECTION('ref_axis',(1.,0.,-4.56777472988634E-14)) ;
#39465=DIRECTION('center_axis',(-4.54195640846217E-14,1.66321791214601E-16,
-1.)) ;
#39466=DIRECTION('ref_axis',(-1.,1.8946420272009E-13,4.54195640846217E-14)) ;
#39467=DIRECTION('center_axis',(-4.54195640846217E-14,1.66321791214601E-16,
-1.)) ;
#39468=DIRECTION('ref_axis',(-1.,1.75658099177411E-13,4.54195640846217E-14)) ;
#39469=DIRECTION('center_axis',(-2.1716102378779E-15,3.83815143260386E-28,
1.)) ;
#39470=DIRECTION('ref_axis',(-1.,1.75658099177411E-13,-2.1716102378779E-15)) ;
#39471=DIRECTION('',(-4.54195640846217E-14,1.66321791214601E-16,-1.)) ;
#39472=DIRECTION('center_axis',(-4.54195640846217E-14,1.66321791214601E-16,
-1.)) ;
#39473=DIRECTION('ref_axis',(-1.,5.55236256206829E-46,4.54195640846217E-14)) ;
#39474=DIRECTION('',(1.75658099177411E-13,1.,1.66321791206623E-16)) ;
#39475=DIRECTION('',(1.,-1.75658099177411E-13,-4.54195640846217E-14)) ;
#39476=DIRECTION('',(-1.75658099177411E-13,-1.,-1.66321791206623E-16)) ;
#39477=DIRECTION('',(-1.,1.75658099177411E-13,4.54195640846217E-14)) ;
#39478=DIRECTION('',(-1.,3.33066907386739E-16,4.54195640846217E-14)) ;
#39479=DIRECTION('center_axis',(-4.54195640846217E-14,1.66321791214601E-16,
-1.)) ;
#39480=DIRECTION('ref_axis',(1.,-5.55236256206829E-46,-4.54195640846217E-14)) ;
#39481=DIRECTION('',(-8.32667268460786E-17,-1.,-1.66321791214597E-16)) ;
#39482=DIRECTION('center_axis',(-4.54195640846217E-14,1.66321791214601E-16,
-1.)) ;
#39483=DIRECTION('ref_axis',(1.,-5.55236256206829E-46,-4.54195640846217E-14)) ;
#39484=DIRECTION('',(1.,-3.33066907386739E-16,-4.54195640846217E-14)) ;
#39485=DIRECTION('center_axis',(-4.54195640846217E-14,1.66321791214601E-16,
-1.)) ;
#39486=DIRECTION('ref_axis',(1.,-5.55236256206829E-46,-4.54195640846217E-14)) ;
#39487=DIRECTION('',(1.66533453692965E-16,1.,1.66321791214593E-16)) ;
#39488=DIRECTION('center_axis',(-4.54195640846217E-14,1.66321791214601E-16,
-1.)) ;
#39489=DIRECTION('ref_axis',(1.,-5.55236256206829E-46,-4.54195640846217E-14)) ;
#39490=DIRECTION('center_axis',(-4.54195640846217E-14,1.66321791214601E-16,
-1.)) ;
#39491=DIRECTION('ref_axis',(-1.,0.,4.46626862477777E-14)) ;
#39492=DIRECTION('center_axis',(4.54195640846217E-14,-1.66321791214601E-16,
1.)) ;
#39493=DIRECTION('ref_axis',(-1.,1.8946420272009E-13,4.54195640846217E-14)) ;
#39494=DIRECTION('center_axis',(-7.59720474939486E-30,-1.,-1.66321791214601E-16)) ;
#39495=DIRECTION('ref_axis',(1.,0.,-4.56777472988634E-14)) ;
#39496=DIRECTION('center_axis',(-4.54195640846217E-14,1.66321791214601E-16,
-1.)) ;
#39497=DIRECTION('ref_axis',(-1.,1.8946420272009E-13,4.54195640846217E-14)) ;
#39498=DIRECTION('center_axis',(-4.54195640846217E-14,1.66321791214601E-16,
-1.)) ;
#39499=DIRECTION('ref_axis',(-1.,1.75658099177411E-13,4.54195640846217E-14)) ;
#39500=DIRECTION('center_axis',(-2.1716102378779E-15,3.83815143260386E-28,
1.)) ;
#39501=DIRECTION('ref_axis',(-1.,1.75658099177411E-13,-2.1716102378779E-15)) ;
#39502=DIRECTION('',(-4.54195640846217E-14,1.66321791214601E-16,-1.)) ;
#39503=DIRECTION('center_axis',(-4.54195640846217E-14,1.66321791214601E-16,
-1.)) ;
#39504=DIRECTION('ref_axis',(-1.,5.55236256206829E-46,4.54195640846217E-14)) ;
#39505=DIRECTION('',(1.75658099177411E-13,1.,1.66321791206623E-16)) ;
#39506=DIRECTION('',(1.,-1.75658099177411E-13,-4.54195640846217E-14)) ;
#39507=DIRECTION('',(-1.75658099177411E-13,-1.,-1.66321791206623E-16)) ;
#39508=DIRECTION('',(-1.,1.75658099177411E-13,4.54195640846217E-14)) ;
#39509=DIRECTION('',(-1.,3.33066907386739E-16,4.54195640846217E-14)) ;
#39510=DIRECTION('center_axis',(-4.54195640846217E-14,1.66321791214601E-16,
-1.)) ;
#39511=DIRECTION('ref_axis',(1.,-5.55236256206829E-46,-4.54195640846217E-14)) ;
#39512=DIRECTION('',(-8.32667268460786E-17,-1.,-1.66321791214597E-16)) ;
#39513=DIRECTION('center_axis',(-4.54195640846217E-14,1.66321791214601E-16,
-1.)) ;
#39514=DIRECTION('ref_axis',(1.,-5.55236256206829E-46,-4.54195640846217E-14)) ;
#39515=DIRECTION('',(1.,-3.33066907386739E-16,-4.54195640846217E-14)) ;
#39516=DIRECTION('center_axis',(-4.54195640846217E-14,1.66321791214601E-16,
-1.)) ;
#39517=DIRECTION('ref_axis',(1.,-5.55236256206829E-46,-4.54195640846217E-14)) ;
#39518=DIRECTION('',(1.66533453692965E-16,1.,1.66321791214593E-16)) ;
#39519=DIRECTION('center_axis',(-4.54195640846217E-14,1.66321791214601E-16,
-1.)) ;
#39520=DIRECTION('ref_axis',(1.,-5.55236256206829E-46,-4.54195640846217E-14)) ;
#39521=DIRECTION('center_axis',(-4.54195640846217E-14,1.66321791214601E-16,
-1.)) ;
#39522=DIRECTION('ref_axis',(-1.,0.,4.46626862477777E-14)) ;
#39523=DIRECTION('center_axis',(4.54195640846217E-14,-1.66321791214601E-16,
1.)) ;
#39524=DIRECTION('ref_axis',(-1.,1.8946420272009E-13,4.54195640846217E-14)) ;
#39525=DIRECTION('center_axis',(-7.59720474939486E-30,-1.,-1.66321791214601E-16)) ;
#39526=DIRECTION('ref_axis',(1.,0.,-4.56777472988634E-14)) ;
#39527=DIRECTION('center_axis',(-4.54195640846217E-14,1.66321791214601E-16,
-1.)) ;
#39528=DIRECTION('ref_axis',(-1.,1.8946420272009E-13,4.54195640846217E-14)) ;
#39529=DIRECTION('center_axis',(-4.54195640846217E-14,1.66321791214601E-16,
-1.)) ;
#39530=DIRECTION('ref_axis',(-1.,1.75658099177411E-13,4.54195640846217E-14)) ;
#39531=DIRECTION('center_axis',(-2.1716102378779E-15,3.83815143260386E-28,
1.)) ;
#39532=DIRECTION('ref_axis',(-1.,1.75658099177411E-13,-2.1716102378779E-15)) ;
#39533=DIRECTION('',(-4.54195640846217E-14,1.66321791214601E-16,-1.)) ;
#39534=DIRECTION('center_axis',(-4.54195640846217E-14,1.66321791214601E-16,
-1.)) ;
#39535=DIRECTION('ref_axis',(-1.,5.55236256206829E-46,4.54195640846217E-14)) ;
#39536=DIRECTION('',(1.75658099177411E-13,1.,1.66321791206623E-16)) ;
#39537=DIRECTION('',(1.,-1.75658099177411E-13,-4.54195640846217E-14)) ;
#39538=DIRECTION('',(-1.75658099177411E-13,-1.,-1.66321791206623E-16)) ;
#39539=DIRECTION('',(-1.,1.75658099177411E-13,4.54195640846217E-14)) ;
#39540=DIRECTION('',(-1.,3.33066907386739E-16,4.54195640846217E-14)) ;
#39541=DIRECTION('center_axis',(-4.54195640846217E-14,1.66321791214601E-16,
-1.)) ;
#39542=DIRECTION('ref_axis',(1.,-5.55236256206829E-46,-4.54195640846217E-14)) ;
#39543=DIRECTION('',(-8.32667268460786E-17,-1.,-1.66321791214597E-16)) ;
#39544=DIRECTION('center_axis',(-4.54195640846217E-14,1.66321791214601E-16,
-1.)) ;
#39545=DIRECTION('ref_axis',(1.,-5.55236256206829E-46,-4.54195640846217E-14)) ;
#39546=DIRECTION('',(1.,-3.33066907386739E-16,-4.54195640846217E-14)) ;
#39547=DIRECTION('center_axis',(-4.54195640846217E-14,1.66321791214601E-16,
-1.)) ;
#39548=DIRECTION('ref_axis',(1.,-5.55236256206829E-46,-4.54195640846217E-14)) ;
#39549=DIRECTION('',(1.66533453692965E-16,1.,1.66321791214593E-16)) ;
#39550=DIRECTION('center_axis',(-4.54195640846217E-14,1.66321791214601E-16,
-1.)) ;
#39551=DIRECTION('ref_axis',(1.,-5.55236256206829E-46,-4.54195640846217E-14)) ;
#39552=DIRECTION('center_axis',(-4.54195640846217E-14,1.66321791214601E-16,
-1.)) ;
#39553=DIRECTION('ref_axis',(-1.,0.,4.46626862477777E-14)) ;
#39554=DIRECTION('center_axis',(4.54195640846217E-14,-1.66321791214601E-16,
1.)) ;
#39555=DIRECTION('ref_axis',(-1.,1.8946420272009E-13,4.54195640846217E-14)) ;
#39556=DIRECTION('center_axis',(-7.59720474939486E-30,-1.,-1.66321791214601E-16)) ;
#39557=DIRECTION('ref_axis',(1.,0.,-4.56777472988634E-14)) ;
#39558=DIRECTION('center_axis',(-4.54195640846217E-14,1.66321791214601E-16,
-1.)) ;
#39559=DIRECTION('ref_axis',(-1.,1.8946420272009E-13,4.54195640846217E-14)) ;
#39560=DIRECTION('center_axis',(-4.54195640846217E-14,1.66321791214601E-16,
-1.)) ;
#39561=DIRECTION('ref_axis',(-1.,1.75658099177411E-13,4.54195640846217E-14)) ;
#39562=DIRECTION('center_axis',(-2.1716102378779E-15,3.83815143260386E-28,
1.)) ;
#39563=DIRECTION('ref_axis',(-1.,1.75658099177411E-13,-2.1716102378779E-15)) ;
#39564=DIRECTION('',(-4.54195640846217E-14,1.66321791214601E-16,-1.)) ;
#39565=DIRECTION('center_axis',(-4.54195640846217E-14,1.66321791214601E-16,
-1.)) ;
#39566=DIRECTION('ref_axis',(-1.,5.55236256206829E-46,4.54195640846217E-14)) ;
#39567=DIRECTION('',(-1.75658099177411E-13,-1.,-1.66321791206623E-16)) ;
#39568=DIRECTION('',(-1.,1.75658099177411E-13,4.54195640846217E-14)) ;
#39569=DIRECTION('',(1.75658099177411E-13,1.,1.66321791206623E-16)) ;
#39570=DIRECTION('',(1.,-1.75658099177411E-13,-4.54195640846217E-14)) ;
#39571=DIRECTION('',(-1.,3.33066907386739E-16,4.54195640846217E-14)) ;
#39572=DIRECTION('center_axis',(-4.54195640846217E-14,1.66321791214601E-16,
-1.)) ;
#39573=DIRECTION('ref_axis',(1.,-5.55236256206829E-46,-4.54195640846217E-14)) ;
#39574=DIRECTION('',(-8.32667268460786E-17,-1.,-1.66321791214597E-16)) ;
#39575=DIRECTION('center_axis',(-4.54195640846217E-14,1.66321791214601E-16,
-1.)) ;
#39576=DIRECTION('ref_axis',(1.,-5.55236256206829E-46,-4.54195640846217E-14)) ;
#39577=DIRECTION('',(1.,-3.33066907386739E-16,-4.54195640846217E-14)) ;
#39578=DIRECTION('center_axis',(-4.54195640846217E-14,1.66321791214601E-16,
-1.)) ;
#39579=DIRECTION('ref_axis',(1.,-5.55236256206829E-46,-4.54195640846217E-14)) ;
#39580=DIRECTION('',(1.66533453692965E-16,1.,1.66321791214593E-16)) ;
#39581=DIRECTION('center_axis',(-4.54195640846217E-14,1.66321791214601E-16,
-1.)) ;
#39582=DIRECTION('ref_axis',(1.,-5.55236256206829E-46,-4.54195640846217E-14)) ;
#39583=DIRECTION('center_axis',(-4.54195640846217E-14,1.66321791214601E-16,
-1.)) ;
#39584=DIRECTION('ref_axis',(-1.,0.,4.46626862477777E-14)) ;
#39585=DIRECTION('center_axis',(4.54195640846217E-14,-1.66321791214601E-16,
1.)) ;
#39586=DIRECTION('ref_axis',(-1.,1.8946420272009E-13,4.54195640846217E-14)) ;
#39587=DIRECTION('center_axis',(-7.59720474939486E-30,-1.,-1.66321791214601E-16)) ;
#39588=DIRECTION('ref_axis',(1.,0.,-4.56777472988634E-14)) ;
#39589=DIRECTION('center_axis',(-4.54195640846217E-14,1.66321791214601E-16,
-1.)) ;
#39590=DIRECTION('ref_axis',(-1.,1.8946420272009E-13,4.54195640846217E-14)) ;
#39591=DIRECTION('center_axis',(-4.54195640846217E-14,1.66321791214601E-16,
-1.)) ;
#39592=DIRECTION('ref_axis',(-1.,1.75658099177411E-13,4.54195640846217E-14)) ;
#39593=DIRECTION('center_axis',(-2.1716102378779E-15,3.83815143260386E-28,
1.)) ;
#39594=DIRECTION('ref_axis',(-1.,1.75658099177411E-13,-2.1716102378779E-15)) ;
#39595=DIRECTION('',(-4.54195640846217E-14,1.66321791214601E-16,-1.)) ;
#39596=DIRECTION('center_axis',(-4.54195640846217E-14,1.66321791214601E-16,
-1.)) ;
#39597=DIRECTION('ref_axis',(-1.,5.55236256206829E-46,4.54195640846217E-14)) ;
#39598=DIRECTION('',(-1.75658099177411E-13,-1.,-1.66321791206623E-16)) ;
#39599=DIRECTION('',(-1.,1.75658099177411E-13,4.54195640846217E-14)) ;
#39600=DIRECTION('',(1.75658099177411E-13,1.,1.66321791206623E-16)) ;
#39601=DIRECTION('',(1.,-1.75658099177411E-13,-4.54195640846217E-14)) ;
#39602=DIRECTION('',(-1.,3.33066907386739E-16,4.54195640846217E-14)) ;
#39603=DIRECTION('center_axis',(-4.54195640846217E-14,1.66321791214601E-16,
-1.)) ;
#39604=DIRECTION('ref_axis',(1.,-5.55236256206829E-46,-4.54195640846217E-14)) ;
#39605=DIRECTION('',(-8.32667268460786E-17,-1.,-1.66321791214597E-16)) ;
#39606=DIRECTION('center_axis',(-4.54195640846217E-14,1.66321791214601E-16,
-1.)) ;
#39607=DIRECTION('ref_axis',(1.,-5.55236256206829E-46,-4.54195640846217E-14)) ;
#39608=DIRECTION('',(1.,-3.33066907386739E-16,-4.54195640846217E-14)) ;
#39609=DIRECTION('center_axis',(-4.54195640846217E-14,1.66321791214601E-16,
-1.)) ;
#39610=DIRECTION('ref_axis',(1.,-5.55236256206829E-46,-4.54195640846217E-14)) ;
#39611=DIRECTION('',(1.66533453692965E-16,1.,1.66321791214593E-16)) ;
#39612=DIRECTION('center_axis',(-4.54195640846217E-14,1.66321791214601E-16,
-1.)) ;
#39613=DIRECTION('ref_axis',(1.,-5.55236256206829E-46,-4.54195640846217E-14)) ;
#39614=DIRECTION('center_axis',(-4.54195640846217E-14,1.66321791214601E-16,
-1.)) ;
#39615=DIRECTION('ref_axis',(-1.,0.,4.46626862477777E-14)) ;
#39616=DIRECTION('center_axis',(4.54195640846217E-14,-1.66321791214601E-16,
1.)) ;
#39617=DIRECTION('ref_axis',(-1.,1.8946420272009E-13,4.54195640846217E-14)) ;
#39618=DIRECTION('center_axis',(-7.59720474939486E-30,-1.,-1.66321791214601E-16)) ;
#39619=DIRECTION('ref_axis',(1.,0.,-4.56777472988634E-14)) ;
#39620=DIRECTION('center_axis',(-4.54195640846217E-14,1.66321791214601E-16,
-1.)) ;
#39621=DIRECTION('ref_axis',(-1.,1.8946420272009E-13,4.54195640846217E-14)) ;
#39622=DIRECTION('center_axis',(-4.54195640846217E-14,1.66321791214601E-16,
-1.)) ;
#39623=DIRECTION('ref_axis',(-1.,1.75658099177411E-13,4.54195640846217E-14)) ;
#39624=DIRECTION('center_axis',(-2.1716102378779E-15,3.83815143260386E-28,
1.)) ;
#39625=DIRECTION('ref_axis',(-1.,1.75658099177411E-13,-2.1716102378779E-15)) ;
#39626=DIRECTION('',(-4.54195640846217E-14,1.66321791214601E-16,-1.)) ;
#39627=DIRECTION('center_axis',(-4.54195640846217E-14,1.66321791214601E-16,
-1.)) ;
#39628=DIRECTION('ref_axis',(-1.,5.55236256206829E-46,4.54195640846217E-14)) ;
#39629=DIRECTION('',(-1.75658099177411E-13,-1.,-1.66321791206623E-16)) ;
#39630=DIRECTION('',(-1.,1.75658099177411E-13,4.54195640846217E-14)) ;
#39631=DIRECTION('',(1.75658099177411E-13,1.,1.66321791206623E-16)) ;
#39632=DIRECTION('',(1.,-1.75658099177411E-13,-4.54195640846217E-14)) ;
#39633=DIRECTION('',(-1.,3.33066907386739E-16,4.54195640846217E-14)) ;
#39634=DIRECTION('center_axis',(-4.54195640846217E-14,1.66321791214601E-16,
-1.)) ;
#39635=DIRECTION('ref_axis',(1.,-5.55236256206829E-46,-4.54195640846217E-14)) ;
#39636=DIRECTION('',(-8.32667268460786E-17,-1.,-1.66321791214597E-16)) ;
#39637=DIRECTION('center_axis',(-4.54195640846217E-14,1.66321791214601E-16,
-1.)) ;
#39638=DIRECTION('ref_axis',(1.,-5.55236256206829E-46,-4.54195640846217E-14)) ;
#39639=DIRECTION('',(1.,-3.33066907386739E-16,-4.54195640846217E-14)) ;
#39640=DIRECTION('center_axis',(-4.54195640846217E-14,1.66321791214601E-16,
-1.)) ;
#39641=DIRECTION('ref_axis',(1.,-5.55236256206829E-46,-4.54195640846217E-14)) ;
#39642=DIRECTION('',(1.66533453692965E-16,1.,1.66321791214593E-16)) ;
#39643=DIRECTION('center_axis',(-4.54195640846217E-14,1.66321791214601E-16,
-1.)) ;
#39644=DIRECTION('ref_axis',(1.,-5.55236256206829E-46,-4.54195640846217E-14)) ;
#39645=DIRECTION('center_axis',(-4.54195640846217E-14,1.66321791214601E-16,
-1.)) ;
#39646=DIRECTION('ref_axis',(-1.,0.,4.46626862477777E-14)) ;
#39647=DIRECTION('center_axis',(4.54195640846217E-14,-1.66321791214601E-16,
1.)) ;
#39648=DIRECTION('ref_axis',(-1.,1.8946420272009E-13,4.54195640846217E-14)) ;
#39649=DIRECTION('center_axis',(-7.59720474939486E-30,-1.,-1.66321791214601E-16)) ;
#39650=DIRECTION('ref_axis',(1.,0.,-4.56777472988634E-14)) ;
#39651=DIRECTION('center_axis',(-4.54195640846217E-14,1.66321791214601E-16,
-1.)) ;
#39652=DIRECTION('ref_axis',(-1.,1.8946420272009E-13,4.54195640846217E-14)) ;
#39653=DIRECTION('center_axis',(-4.54195640846217E-14,1.66321791214601E-16,
-1.)) ;
#39654=DIRECTION('ref_axis',(-1.,1.75658099177411E-13,4.54195640846217E-14)) ;
#39655=DIRECTION('center_axis',(-2.1716102378779E-15,3.83815143260386E-28,
1.)) ;
#39656=DIRECTION('ref_axis',(-1.,1.75658099177411E-13,-2.1716102378779E-15)) ;
#39657=DIRECTION('',(-4.54195640846217E-14,1.66321791214601E-16,-1.)) ;
#39658=DIRECTION('center_axis',(-4.54195640846217E-14,1.66321791214601E-16,
-1.)) ;
#39659=DIRECTION('ref_axis',(-1.,5.55236256206829E-46,4.54195640846217E-14)) ;
#39660=DIRECTION('',(-1.75658099177411E-13,-1.,-1.66321791206623E-16)) ;
#39661=DIRECTION('',(-1.,1.75658099177411E-13,4.54195640846217E-14)) ;
#39662=DIRECTION('',(1.75658099177411E-13,1.,1.66321791206623E-16)) ;
#39663=DIRECTION('',(1.,-1.75658099177411E-13,-4.54195640846217E-14)) ;
#39664=DIRECTION('',(-1.,3.33066907386739E-16,4.54195640846217E-14)) ;
#39665=DIRECTION('center_axis',(-4.54195640846217E-14,1.66321791214601E-16,
-1.)) ;
#39666=DIRECTION('ref_axis',(1.,-5.55236256206829E-46,-4.54195640846217E-14)) ;
#39667=DIRECTION('',(-8.32667268460786E-17,-1.,-1.66321791214597E-16)) ;
#39668=DIRECTION('center_axis',(-4.54195640846217E-14,1.66321791214601E-16,
-1.)) ;
#39669=DIRECTION('ref_axis',(1.,-5.55236256206829E-46,-4.54195640846217E-14)) ;
#39670=DIRECTION('',(1.,-3.33066907386739E-16,-4.54195640846217E-14)) ;
#39671=DIRECTION('center_axis',(-4.54195640846217E-14,1.66321791214601E-16,
-1.)) ;
#39672=DIRECTION('ref_axis',(1.,-5.55236256206829E-46,-4.54195640846217E-14)) ;
#39673=DIRECTION('',(1.66533453692965E-16,1.,1.66321791214593E-16)) ;
#39674=DIRECTION('center_axis',(-4.54195640846217E-14,1.66321791214601E-16,
-1.)) ;
#39675=DIRECTION('ref_axis',(1.,-5.55236256206829E-46,-4.54195640846217E-14)) ;
#39676=DIRECTION('center_axis',(-4.54195640846217E-14,1.66321791214601E-16,
-1.)) ;
#39677=DIRECTION('ref_axis',(-1.,0.,4.46626862477777E-14)) ;
#39678=DIRECTION('center_axis',(4.54195640846217E-14,-1.66321791214601E-16,
1.)) ;
#39679=DIRECTION('ref_axis',(-1.,1.8946420272009E-13,4.54195640846217E-14)) ;
#39680=DIRECTION('center_axis',(-7.59720474939486E-30,-1.,-1.66321791214601E-16)) ;
#39681=DIRECTION('ref_axis',(1.,0.,-4.56777472988634E-14)) ;
#39682=DIRECTION('center_axis',(-4.54195640846217E-14,1.66321791214601E-16,
-1.)) ;
#39683=DIRECTION('ref_axis',(-1.,1.8946420272009E-13,4.54195640846217E-14)) ;
#39684=DIRECTION('center_axis',(-4.54195640846217E-14,1.66321791214601E-16,
-1.)) ;
#39685=DIRECTION('ref_axis',(-1.,5.55236256206829E-46,4.54195640846217E-14)) ;
#39686=DIRECTION('',(-1.75658099177411E-13,-1.,-1.66321791206623E-16)) ;
#39687=DIRECTION('',(-1.,1.75658099177411E-13,4.54195640846217E-14)) ;
#39688=DIRECTION('',(1.75658099177411E-13,1.,1.66321791206623E-16)) ;
#39689=DIRECTION('',(1.,-1.75658099177411E-13,-4.54195640846217E-14)) ;
#39690=DIRECTION('',(1.,-3.33066907386739E-16,-4.54195640846217E-14)) ;
#39691=DIRECTION('center_axis',(-4.54195640846217E-14,1.66321791214601E-16,
-1.)) ;
#39692=DIRECTION('ref_axis',(-0.707106781186502,0.707106781186593,3.22340890291979E-14)) ;
#39693=DIRECTION('',(8.32667268460786E-17,1.,1.66321791214597E-16)) ;
#39694=DIRECTION('center_axis',(-4.54195640846217E-14,1.66321791214601E-16,
-1.)) ;
#39695=DIRECTION('ref_axis',(-0.707106781186502,-0.707106781186593,3.1998874496344E-14)) ;
#39696=DIRECTION('',(-1.,3.33066907386739E-16,4.54195640846217E-14)) ;
#39697=DIRECTION('center_axis',(-4.54195640846217E-14,1.66321791214601E-16,
-1.)) ;
#39698=DIRECTION('ref_axis',(0.707106781186593,-0.707106781186502,-3.2234089029202E-14)) ;
#39699=DIRECTION('',(-1.66533453692965E-16,-1.,-1.66321791214593E-16)) ;
#39700=DIRECTION('center_axis',(-4.54195640846217E-14,1.66321791214601E-16,
-1.)) ;
#39701=DIRECTION('ref_axis',(0.707106781186593,0.707106781186502,-3.19988744963481E-14)) ;
#39702=DIRECTION('center_axis',(-4.54195640846217E-14,1.66321791214601E-16,
-1.)) ;
#39703=DIRECTION('ref_axis',(-1.,1.75658099177411E-13,4.54195640846217E-14)) ;
#39704=DIRECTION('center_axis',(-2.1716102378779E-15,3.83815143260386E-28,
1.)) ;
#39705=DIRECTION('ref_axis',(-1.,1.75658099177411E-13,-2.1716102378779E-15)) ;
#39706=DIRECTION('',(-4.54195640846217E-14,1.66321791214601E-16,-1.)) ;
#39707=DIRECTION('center_axis',(2.1716102378779E-15,-3.83815143260386E-28,
-1.)) ;
#39708=DIRECTION('ref_axis',(1.,-1.66533453692941E-16,2.1716102378779E-15)) ;
#39709=DIRECTION('center_axis',(-2.1716102378779E-15,3.83815143260386E-28,
1.)) ;
#39710=DIRECTION('ref_axis',(-1.,-7.33033736753389E-16,-2.1716102378779E-15)) ;
#39711=DIRECTION('center_axis',(2.1716102378779E-15,-3.83815143260386E-28,
-1.)) ;
#39712=DIRECTION('ref_axis',(1.,-1.66533453692941E-16,2.1716102378779E-15)) ;
#39713=DIRECTION('center_axis',(-2.1716102378779E-15,3.83815143260386E-28,
1.)) ;
#39714=DIRECTION('ref_axis',(-1.,-7.33033736753389E-16,-2.1716102378779E-15)) ;
#39715=DIRECTION('center_axis',(2.1716102378779E-15,-3.83815143260386E-28,
-1.)) ;
#39716=DIRECTION('ref_axis',(1.,-1.66533453692941E-16,2.1716102378779E-15)) ;
#39717=DIRECTION('center_axis',(-2.1716102378779E-15,3.83815143260386E-28,
1.)) ;
#39718=DIRECTION('ref_axis',(-1.,-7.33033736753389E-16,-2.1716102378779E-15)) ;
#39719=DIRECTION('center_axis',(2.1716102378779E-15,-3.83815143260386E-28,
-1.)) ;
#39720=DIRECTION('ref_axis',(1.,-1.66533453692941E-16,2.1716102378779E-15)) ;
#39721=DIRECTION('center_axis',(-2.1716102378779E-15,3.83815143260386E-28,
1.)) ;
#39722=DIRECTION('ref_axis',(-1.,-7.33033736753389E-16,-2.1716102378779E-15)) ;
#39723=DIRECTION('center_axis',(2.1716102378779E-15,-3.83815143260386E-28,
-1.)) ;
#39724=DIRECTION('ref_axis',(1.,-1.66533453692941E-16,2.1716102378779E-15)) ;
#39725=DIRECTION('center_axis',(-2.1716102378779E-15,3.83815143260386E-28,
1.)) ;
#39726=DIRECTION('ref_axis',(-1.,-7.33033736753389E-16,-2.1716102378779E-15)) ;
#39727=DIRECTION('center_axis',(2.1716102378779E-15,-3.83815143260386E-28,
-1.)) ;
#39728=DIRECTION('ref_axis',(1.,-1.66533453692941E-16,2.1716102378779E-15)) ;
#39729=DIRECTION('center_axis',(-2.1716102378779E-15,3.83815143260386E-28,
1.)) ;
#39730=DIRECTION('ref_axis',(-1.,-7.33033736753389E-16,-2.1716102378779E-15)) ;
#39731=DIRECTION('center_axis',(2.1716102378779E-15,-3.83815143260386E-28,
-1.)) ;
#39732=DIRECTION('ref_axis',(1.,-1.66533453692941E-16,2.1716102378779E-15)) ;
#39733=DIRECTION('center_axis',(-2.1716102378779E-15,3.83815143260386E-28,
1.)) ;
#39734=DIRECTION('ref_axis',(-1.,-7.33033736753389E-16,-2.1716102378779E-15)) ;
#39735=DIRECTION('center_axis',(2.1716102378779E-15,-3.83815143260386E-28,
-1.)) ;
#39736=DIRECTION('ref_axis',(1.,-1.66533453692941E-16,2.1716102378779E-15)) ;
#39737=DIRECTION('center_axis',(-2.1716102378779E-15,3.83815143260386E-28,
1.)) ;
#39738=DIRECTION('ref_axis',(-1.,-7.33033736753389E-16,-2.1716102378779E-15)) ;
#39739=DIRECTION('center_axis',(-1.,3.33066907386739E-16,4.54195640846217E-14)) ;
#39740=DIRECTION('ref_axis',(-3.23519956315716E-14,-0.707106781186623,-0.707106781186472)) ;
#39741=DIRECTION('center_axis',(-1.,0.,0.)) ;
#39742=DIRECTION('ref_axis',(0.,0.,-1.)) ;
#39743=DIRECTION('',(-1.,3.33066907386739E-16,4.54195640846217E-14)) ;
#39744=DIRECTION('center_axis',(1.,0.,0.)) ;
#39745=DIRECTION('ref_axis',(0.,-1.,0.)) ;
#39746=DIRECTION('center_axis',(4.54195640846217E-14,-1.66321791214601E-16,
1.)) ;
#39747=DIRECTION('ref_axis',(1.,0.,-4.54747350886464E-14)) ;
#39748=DIRECTION('center_axis',(0.,1.,0.)) ;
#39749=DIRECTION('ref_axis',(1.,0.,-3.5527136788002E-14)) ;
#39750=DIRECTION('center_axis',(2.17161023787787E-15,-3.6685463379813E-28,
-1.)) ;
#39751=DIRECTION('ref_axis',(-0.707106781186543,0.707106781186552,-1.53556032529782E-15)) ;
#39752=DIRECTION('center_axis',(-8.32667268460786E-17,-1.,-1.66321791214597E-16)) ;
#39753=DIRECTION('ref_axis',(0.707106781186522,5.87287992268709E-17,-0.707106781186573)) ;
#39754=DIRECTION('center_axis',(0.,1.,0.)) ;
#39755=DIRECTION('ref_axis',(1.,0.,0.)) ;
#39756=DIRECTION('',(-8.32667268460786E-17,-1.,-1.66321791214597E-16)) ;
#39757=DIRECTION('center_axis',(4.54195640846217E-14,-1.66321791214601E-16,
1.)) ;
#39758=DIRECTION('ref_axis',(1.,0.,-4.54747350886464E-14)) ;
#39759=DIRECTION('center_axis',(-1.,-2.84217094303975E-13,0.)) ;
#39760=DIRECTION('ref_axis',(-2.84217094303975E-13,1.,0.)) ;
#39761=DIRECTION('center_axis',(-2.17161023787787E-15,3.6685463379813E-28,
1.)) ;
#39762=DIRECTION('ref_axis',(-0.707106781186552,-0.707106781186543,-1.53556032529732E-15)) ;
#39763=DIRECTION('center_axis',(1.,-3.33066907386739E-16,-4.54195640846217E-14)) ;
#39764=DIRECTION('ref_axis',(-3.18809678939767E-14,0.707106781186422,-0.707106781186673)) ;
#39765=DIRECTION('center_axis',(-1.,0.,0.)) ;
#39766=DIRECTION('ref_axis',(0.,1.,0.)) ;
#39767=DIRECTION('',(1.,-3.33066907386739E-16,-4.54195640846217E-14)) ;
#39768=DIRECTION('center_axis',(4.54195640846217E-14,-1.66321791214601E-16,
1.)) ;
#39769=DIRECTION('ref_axis',(1.,0.,-4.54747350886464E-14)) ;
#39770=DIRECTION('center_axis',(0.,-1.,0.)) ;
#39771=DIRECTION('ref_axis',(-1.,0.,3.5527136788007E-14)) ;
#39772=DIRECTION('center_axis',(2.1716102378779E-15,-3.66854633798134E-28,
-1.)) ;
#39773=DIRECTION('ref_axis',(0.707106781186543,-0.707106781186552,1.53556032529784E-15)) ;
#39774=DIRECTION('center_axis',(1.66533453692965E-16,1.,1.66321791214593E-16)) ;
#39775=DIRECTION('ref_axis',(-0.707106781186522,2.35364200827643E-16,-0.707106781186573)) ;
#39776=DIRECTION('center_axis',(0.,-1.,0.)) ;
#39777=DIRECTION('ref_axis',(-1.,0.,0.)) ;
#39778=DIRECTION('',(1.66533453692965E-16,1.,1.66321791214593E-16)) ;
#39779=DIRECTION('center_axis',(4.54195640846217E-14,-1.66321791214601E-16,
1.)) ;
#39780=DIRECTION('ref_axis',(1.,0.,-4.54747350886464E-14)) ;
#39781=DIRECTION('center_axis',(-2.1716102378779E-15,3.66854633798134E-28,
1.)) ;
#39782=DIRECTION('ref_axis',(0.707106781186452,0.707106781186643,1.53556032529713E-15)) ;
#39783=DIRECTION('center_axis',(-2.17161023787787E-15,3.6685463379813E-28,
1.)) ;
#39784=DIRECTION('ref_axis',(-0.707106781186552,-0.707106781186543,-1.53556032529732E-15)) ;
#39785=DIRECTION('',(2.17161023787787E-15,-3.6685463379813E-28,-1.)) ;
#39786=DIRECTION('center_axis',(1.88526971141291E-28,-2.90739654573716E-15,
-1.)) ;
#39787=DIRECTION('ref_axis',(1.35627620245787E-13,-1.,2.90739654573716E-15)) ;
#39788=DIRECTION('',(-2.17161023787787E-15,3.6685463379813E-28,1.)) ;
#39789=DIRECTION('center_axis',(-1.,8.32667268460789E-17,-2.17161023787787E-15)) ;
#39790=DIRECTION('ref_axis',(8.32667268460789E-17,1.,-3.92101138914083E-28)) ;
#39791=DIRECTION('',(-2.17161023787787E-15,3.6685463379813E-28,1.)) ;
#39792=DIRECTION('center_axis',(-1.,8.32667268460789E-17,-2.17161023787787E-15)) ;
#39793=DIRECTION('ref_axis',(-1.59443879249779E-15,-0.707106781186479,0.707106781186616)) ;
#39794=DIRECTION('',(8.32667268460789E-17,1.,-3.83780830390118E-28)) ;
#39795=DIRECTION('',(-2.17161023787787E-15,3.83815143260382E-28,1.)) ;
#39796=DIRECTION('',(8.32667268460786E-17,1.,1.66321791214597E-16)) ;
#39797=DIRECTION('',(2.17161023787787E-15,-3.83420712807771E-28,-1.)) ;
#39798=DIRECTION('',(8.32667268460789E-17,1.,-3.83780830390118E-28)) ;
#39799=DIRECTION('center_axis',(-1.,8.32667268460789E-17,-2.17161023787787E-15)) ;
#39800=DIRECTION('ref_axis',(-1.47668185809765E-15,0.707106781186483,0.707106781186612)) ;
#39801=DIRECTION('center_axis',(2.17161023787787E-15,-3.6685463379813E-28,
-1.)) ;
#39802=DIRECTION('ref_axis',(-0.707106781186543,0.707106781186552,-1.53556032529782E-15)) ;
#39803=DIRECTION('',(2.17161023787787E-15,-3.6685463379813E-28,-1.)) ;
#39804=DIRECTION('center_axis',(1.88526971141291E-28,-2.90739654573716E-15,
-1.)) ;
#39805=DIRECTION('ref_axis',(-1.,6.48092690620067E-15,-2.07369595641554E-28)) ;
#39806=DIRECTION('center_axis',(3.33066907386739E-16,1.,-3.66031460022645E-28)) ;
#39807=DIRECTION('ref_axis',(2.17161023787795E-15,-3.66754751528624E-28,
-1.)) ;
#39808=DIRECTION('',(-2.1716102378779E-15,3.66854633798134E-28,1.)) ;
#39809=DIRECTION('',(-1.,3.33066907386739E-16,-2.1716102378779E-15)) ;
#39810=DIRECTION('center_axis',(-1.,3.33066907386739E-16,4.54195640846217E-14)) ;
#39811=DIRECTION('ref_axis',(-3.23519956315716E-14,-0.707106781186623,-0.707106781186472)) ;
#39812=DIRECTION('center_axis',(-1.,0.,0.)) ;
#39813=DIRECTION('ref_axis',(0.,0.,-1.)) ;
#39814=DIRECTION('',(-1.,3.33066907386739E-16,4.54195640846217E-14)) ;
#39815=DIRECTION('center_axis',(1.,0.,0.)) ;
#39816=DIRECTION('ref_axis',(0.,-1.,0.)) ;
#39817=DIRECTION('center_axis',(4.54195640846217E-14,-1.66321791214601E-16,
1.)) ;
#39818=DIRECTION('ref_axis',(1.,0.,-4.54747350886464E-14)) ;
#39819=DIRECTION('center_axis',(0.,1.,0.)) ;
#39820=DIRECTION('ref_axis',(1.,0.,-3.5527136788002E-14)) ;
#39821=DIRECTION('center_axis',(2.17161023787787E-15,-3.6685463379813E-28,
-1.)) ;
#39822=DIRECTION('ref_axis',(-0.707106781186543,0.707106781186552,-1.53556032529782E-15)) ;
#39823=DIRECTION('center_axis',(-8.32667268460786E-17,-1.,-1.66321791214597E-16)) ;
#39824=DIRECTION('ref_axis',(0.707106781186522,5.87287992268709E-17,-0.707106781186573)) ;
#39825=DIRECTION('center_axis',(0.,1.,0.)) ;
#39826=DIRECTION('ref_axis',(1.,0.,0.)) ;
#39827=DIRECTION('',(-8.32667268460786E-17,-1.,-1.66321791214597E-16)) ;
#39828=DIRECTION('center_axis',(4.54195640846217E-14,-1.66321791214601E-16,
1.)) ;
#39829=DIRECTION('ref_axis',(1.,0.,-4.54747350886464E-14)) ;
#39830=DIRECTION('center_axis',(-1.,-2.84217094303975E-13,0.)) ;
#39831=DIRECTION('ref_axis',(-2.84217094303975E-13,1.,0.)) ;
#39832=DIRECTION('center_axis',(-2.17161023787787E-15,3.6685463379813E-28,
1.)) ;
#39833=DIRECTION('ref_axis',(-0.707106781186552,-0.707106781186543,-1.53556032529732E-15)) ;
#39834=DIRECTION('center_axis',(1.,-3.33066907386739E-16,-4.54195640846217E-14)) ;
#39835=DIRECTION('ref_axis',(-3.18809678939767E-14,0.707106781186422,-0.707106781186673)) ;
#39836=DIRECTION('center_axis',(-1.,0.,0.)) ;
#39837=DIRECTION('ref_axis',(0.,1.,0.)) ;
#39838=DIRECTION('',(1.,-3.33066907386739E-16,-4.54195640846217E-14)) ;
#39839=DIRECTION('center_axis',(4.54195640846217E-14,-1.66321791214601E-16,
1.)) ;
#39840=DIRECTION('ref_axis',(1.,0.,-4.54747350886464E-14)) ;
#39841=DIRECTION('center_axis',(0.,-1.,0.)) ;
#39842=DIRECTION('ref_axis',(-1.,0.,3.5527136788007E-14)) ;
#39843=DIRECTION('center_axis',(2.1716102378779E-15,-3.66854633798134E-28,
-1.)) ;
#39844=DIRECTION('ref_axis',(0.707106781186543,-0.707106781186552,1.53556032529784E-15)) ;
#39845=DIRECTION('center_axis',(1.66533453692965E-16,1.,1.66321791214593E-16)) ;
#39846=DIRECTION('ref_axis',(-0.707106781186522,2.35364200827643E-16,-0.707106781186573)) ;
#39847=DIRECTION('center_axis',(0.,-1.,0.)) ;
#39848=DIRECTION('ref_axis',(-1.,0.,0.)) ;
#39849=DIRECTION('',(1.66533453692965E-16,1.,1.66321791214593E-16)) ;
#39850=DIRECTION('center_axis',(4.54195640846217E-14,-1.66321791214601E-16,
1.)) ;
#39851=DIRECTION('ref_axis',(1.,0.,-4.54747350886464E-14)) ;
#39852=DIRECTION('center_axis',(-2.1716102378779E-15,3.66854633798134E-28,
1.)) ;
#39853=DIRECTION('ref_axis',(0.707106781186452,0.707106781186643,1.53556032529713E-15)) ;
#39854=DIRECTION('center_axis',(-2.17161023787787E-15,3.6685463379813E-28,
1.)) ;
#39855=DIRECTION('ref_axis',(-0.707106781186552,-0.707106781186543,-1.53556032529732E-15)) ;
#39856=DIRECTION('',(2.17161023787787E-15,-3.6685463379813E-28,-1.)) ;
#39857=DIRECTION('center_axis',(1.88526971141291E-28,-2.90739654573716E-15,
-1.)) ;
#39858=DIRECTION('ref_axis',(1.35627620245787E-13,-1.,2.90739654573716E-15)) ;
#39859=DIRECTION('',(-2.17161023787787E-15,3.6685463379813E-28,1.)) ;
#39860=DIRECTION('center_axis',(-1.,8.32667268460789E-17,-2.17161023787787E-15)) ;
#39861=DIRECTION('ref_axis',(8.32667268460789E-17,1.,-3.92101138914083E-28)) ;
#39862=DIRECTION('',(-2.17161023787787E-15,3.6685463379813E-28,1.)) ;
#39863=DIRECTION('center_axis',(-1.,8.32667268460789E-17,-2.17161023787787E-15)) ;
#39864=DIRECTION('ref_axis',(-1.59443879249779E-15,-0.707106781186479,0.707106781186616)) ;
#39865=DIRECTION('',(8.32667268460789E-17,1.,-3.83780830390118E-28)) ;
#39866=DIRECTION('',(-2.17161023787787E-15,3.83815143260382E-28,1.)) ;
#39867=DIRECTION('',(8.32667268460786E-17,1.,1.66321791214597E-16)) ;
#39868=DIRECTION('',(2.17161023787787E-15,-3.83420712807771E-28,-1.)) ;
#39869=DIRECTION('',(8.32667268460789E-17,1.,-3.83780830390118E-28)) ;
#39870=DIRECTION('center_axis',(-1.,8.32667268460789E-17,-2.17161023787787E-15)) ;
#39871=DIRECTION('ref_axis',(-1.47668185809765E-15,0.707106781186483,0.707106781186612)) ;
#39872=DIRECTION('center_axis',(2.17161023787787E-15,-3.6685463379813E-28,
-1.)) ;
#39873=DIRECTION('ref_axis',(-0.707106781186543,0.707106781186552,-1.53556032529782E-15)) ;
#39874=DIRECTION('',(2.17161023787787E-15,-3.6685463379813E-28,-1.)) ;
#39875=DIRECTION('center_axis',(1.88526971141291E-28,-2.90739654573716E-15,
-1.)) ;
#39876=DIRECTION('ref_axis',(-1.,6.48092690620067E-15,-2.07369595641554E-28)) ;
#39877=DIRECTION('center_axis',(3.33066907386739E-16,1.,-3.66031460022645E-28)) ;
#39878=DIRECTION('ref_axis',(2.17161023787795E-15,-3.66754751528624E-28,
-1.)) ;
#39879=DIRECTION('',(-2.1716102378779E-15,3.66854633798134E-28,1.)) ;
#39880=DIRECTION('',(-1.,3.33066907386739E-16,-2.1716102378779E-15)) ;
#39881=DIRECTION('center_axis',(-1.,3.33066907386739E-16,4.54195640846217E-14)) ;
#39882=DIRECTION('ref_axis',(-3.23519956315716E-14,-0.707106781186623,-0.707106781186472)) ;
#39883=DIRECTION('center_axis',(-1.,0.,0.)) ;
#39884=DIRECTION('ref_axis',(0.,0.,-1.)) ;
#39885=DIRECTION('',(-1.,3.33066907386739E-16,4.54195640846217E-14)) ;
#39886=DIRECTION('center_axis',(1.,0.,0.)) ;
#39887=DIRECTION('ref_axis',(0.,-1.,0.)) ;
#39888=DIRECTION('center_axis',(4.54195640846217E-14,-1.66321791214601E-16,
1.)) ;
#39889=DIRECTION('ref_axis',(1.,0.,-4.54747350886464E-14)) ;
#39890=DIRECTION('center_axis',(0.,1.,0.)) ;
#39891=DIRECTION('ref_axis',(1.,0.,-3.5527136788002E-14)) ;
#39892=DIRECTION('center_axis',(2.17161023787787E-15,-3.6685463379813E-28,
-1.)) ;
#39893=DIRECTION('ref_axis',(-0.707106781186543,0.707106781186552,-1.53556032529782E-15)) ;
#39894=DIRECTION('center_axis',(-8.32667268460786E-17,-1.,-1.66321791214597E-16)) ;
#39895=DIRECTION('ref_axis',(0.707106781186522,5.87287992268709E-17,-0.707106781186573)) ;
#39896=DIRECTION('center_axis',(0.,1.,0.)) ;
#39897=DIRECTION('ref_axis',(1.,0.,0.)) ;
#39898=DIRECTION('',(-8.32667268460786E-17,-1.,-1.66321791214597E-16)) ;
#39899=DIRECTION('center_axis',(4.54195640846217E-14,-1.66321791214601E-16,
1.)) ;
#39900=DIRECTION('ref_axis',(1.,0.,-4.54747350886464E-14)) ;
#39901=DIRECTION('center_axis',(-1.,-2.84217094303975E-13,0.)) ;
#39902=DIRECTION('ref_axis',(-2.84217094303975E-13,1.,0.)) ;
#39903=DIRECTION('center_axis',(-2.17161023787787E-15,3.6685463379813E-28,
1.)) ;
#39904=DIRECTION('ref_axis',(-0.707106781186552,-0.707106781186543,-1.53556032529732E-15)) ;
#39905=DIRECTION('center_axis',(1.,-3.33066907386739E-16,-4.54195640846217E-14)) ;
#39906=DIRECTION('ref_axis',(-3.18809678939767E-14,0.707106781186422,-0.707106781186673)) ;
#39907=DIRECTION('center_axis',(-1.,0.,0.)) ;
#39908=DIRECTION('ref_axis',(0.,1.,0.)) ;
#39909=DIRECTION('',(1.,-3.33066907386739E-16,-4.54195640846217E-14)) ;
#39910=DIRECTION('center_axis',(4.54195640846217E-14,-1.66321791214601E-16,
1.)) ;
#39911=DIRECTION('ref_axis',(1.,0.,-4.54747350886464E-14)) ;
#39912=DIRECTION('center_axis',(0.,-1.,0.)) ;
#39913=DIRECTION('ref_axis',(-1.,0.,3.5527136788007E-14)) ;
#39914=DIRECTION('center_axis',(2.1716102378779E-15,-3.66854633798134E-28,
-1.)) ;
#39915=DIRECTION('ref_axis',(0.707106781186543,-0.707106781186552,1.53556032529784E-15)) ;
#39916=DIRECTION('center_axis',(1.66533453692965E-16,1.,1.66321791214593E-16)) ;
#39917=DIRECTION('ref_axis',(-0.707106781186522,2.35364200827643E-16,-0.707106781186573)) ;
#39918=DIRECTION('center_axis',(0.,-1.,0.)) ;
#39919=DIRECTION('ref_axis',(-1.,0.,0.)) ;
#39920=DIRECTION('',(1.66533453692965E-16,1.,1.66321791214593E-16)) ;
#39921=DIRECTION('center_axis',(4.54195640846217E-14,-1.66321791214601E-16,
1.)) ;
#39922=DIRECTION('ref_axis',(1.,0.,-4.54747350886464E-14)) ;
#39923=DIRECTION('center_axis',(-2.1716102378779E-15,3.66854633798134E-28,
1.)) ;
#39924=DIRECTION('ref_axis',(0.707106781186452,0.707106781186643,1.53556032529713E-15)) ;
#39925=DIRECTION('center_axis',(-2.17161023787787E-15,3.6685463379813E-28,
1.)) ;
#39926=DIRECTION('ref_axis',(-0.707106781186552,-0.707106781186543,-1.53556032529732E-15)) ;
#39927=DIRECTION('',(2.17161023787787E-15,-3.6685463379813E-28,-1.)) ;
#39928=DIRECTION('center_axis',(1.88526971141291E-28,-2.90739654573716E-15,
-1.)) ;
#39929=DIRECTION('ref_axis',(1.35627620245787E-13,-1.,2.90739654573716E-15)) ;
#39930=DIRECTION('',(-2.17161023787787E-15,3.6685463379813E-28,1.)) ;
#39931=DIRECTION('center_axis',(-1.,8.32667268460789E-17,-2.17161023787787E-15)) ;
#39932=DIRECTION('ref_axis',(8.32667268460789E-17,1.,-3.92101138914083E-28)) ;
#39933=DIRECTION('',(-2.17161023787787E-15,3.6685463379813E-28,1.)) ;
#39934=DIRECTION('center_axis',(-1.,8.32667268460789E-17,-2.17161023787787E-15)) ;
#39935=DIRECTION('ref_axis',(-1.59443879249779E-15,-0.707106781186479,0.707106781186616)) ;
#39936=DIRECTION('',(8.32667268460789E-17,1.,-3.83780830390118E-28)) ;
#39937=DIRECTION('',(-2.17161023787787E-15,3.83815143260382E-28,1.)) ;
#39938=DIRECTION('',(8.32667268460786E-17,1.,1.66321791214597E-16)) ;
#39939=DIRECTION('',(2.17161023787787E-15,-3.83420712807771E-28,-1.)) ;
#39940=DIRECTION('',(8.32667268460789E-17,1.,-3.83780830390118E-28)) ;
#39941=DIRECTION('center_axis',(-1.,8.32667268460789E-17,-2.17161023787787E-15)) ;
#39942=DIRECTION('ref_axis',(-1.47668185809765E-15,0.707106781186483,0.707106781186612)) ;
#39943=DIRECTION('center_axis',(2.17161023787787E-15,-3.6685463379813E-28,
-1.)) ;
#39944=DIRECTION('ref_axis',(-0.707106781186543,0.707106781186552,-1.53556032529782E-15)) ;
#39945=DIRECTION('',(2.17161023787787E-15,-3.6685463379813E-28,-1.)) ;
#39946=DIRECTION('center_axis',(1.88526971141291E-28,-2.90739654573716E-15,
-1.)) ;
#39947=DIRECTION('ref_axis',(-1.,6.48092690620067E-15,-2.07369595641554E-28)) ;
#39948=DIRECTION('center_axis',(3.33066907386739E-16,1.,-3.66031460022645E-28)) ;
#39949=DIRECTION('ref_axis',(2.17161023787795E-15,-3.66754751528624E-28,
-1.)) ;
#39950=DIRECTION('',(-2.1716102378779E-15,3.66854633798134E-28,1.)) ;
#39951=DIRECTION('',(-1.,3.33066907386739E-16,-2.1716102378779E-15)) ;
#39952=DIRECTION('center_axis',(-1.,3.33066907386739E-16,4.54195640846217E-14)) ;
#39953=DIRECTION('ref_axis',(-3.23519956315716E-14,-0.707106781186623,-0.707106781186472)) ;
#39954=DIRECTION('center_axis',(-1.,0.,0.)) ;
#39955=DIRECTION('ref_axis',(0.,0.,-1.)) ;
#39956=DIRECTION('',(-1.,3.33066907386739E-16,4.54195640846217E-14)) ;
#39957=DIRECTION('center_axis',(1.,0.,0.)) ;
#39958=DIRECTION('ref_axis',(0.,-1.,0.)) ;
#39959=DIRECTION('center_axis',(4.54195640846217E-14,-1.66321791214601E-16,
1.)) ;
#39960=DIRECTION('ref_axis',(1.,0.,-4.54747350886464E-14)) ;
#39961=DIRECTION('center_axis',(0.,1.,0.)) ;
#39962=DIRECTION('ref_axis',(1.,0.,-3.5527136788002E-14)) ;
#39963=DIRECTION('center_axis',(2.17161023787787E-15,-3.6685463379813E-28,
-1.)) ;
#39964=DIRECTION('ref_axis',(-0.707106781186543,0.707106781186552,-1.53556032529782E-15)) ;
#39965=DIRECTION('center_axis',(-8.32667268460786E-17,-1.,-1.66321791214597E-16)) ;
#39966=DIRECTION('ref_axis',(0.707106781186522,5.87287992268709E-17,-0.707106781186573)) ;
#39967=DIRECTION('center_axis',(0.,1.,0.)) ;
#39968=DIRECTION('ref_axis',(1.,0.,0.)) ;
#39969=DIRECTION('',(-8.32667268460786E-17,-1.,-1.66321791214597E-16)) ;
#39970=DIRECTION('center_axis',(4.54195640846217E-14,-1.66321791214601E-16,
1.)) ;
#39971=DIRECTION('ref_axis',(1.,0.,-4.54747350886464E-14)) ;
#39972=DIRECTION('center_axis',(-1.,-2.84217094303975E-13,0.)) ;
#39973=DIRECTION('ref_axis',(-2.84217094303975E-13,1.,0.)) ;
#39974=DIRECTION('center_axis',(-2.17161023787787E-15,3.6685463379813E-28,
1.)) ;
#39975=DIRECTION('ref_axis',(-0.707106781186552,-0.707106781186543,-1.53556032529732E-15)) ;
#39976=DIRECTION('center_axis',(1.,-3.33066907386739E-16,-4.54195640846217E-14)) ;
#39977=DIRECTION('ref_axis',(-3.18809678939767E-14,0.707106781186422,-0.707106781186673)) ;
#39978=DIRECTION('center_axis',(-1.,0.,0.)) ;
#39979=DIRECTION('ref_axis',(0.,1.,0.)) ;
#39980=DIRECTION('',(1.,-3.33066907386739E-16,-4.54195640846217E-14)) ;
#39981=DIRECTION('center_axis',(4.54195640846217E-14,-1.66321791214601E-16,
1.)) ;
#39982=DIRECTION('ref_axis',(1.,0.,-4.54747350886464E-14)) ;
#39983=DIRECTION('center_axis',(0.,-1.,0.)) ;
#39984=DIRECTION('ref_axis',(-1.,0.,3.5527136788007E-14)) ;
#39985=DIRECTION('center_axis',(2.1716102378779E-15,-3.66854633798134E-28,
-1.)) ;
#39986=DIRECTION('ref_axis',(0.707106781186543,-0.707106781186552,1.53556032529784E-15)) ;
#39987=DIRECTION('center_axis',(1.66533453692965E-16,1.,1.66321791214593E-16)) ;
#39988=DIRECTION('ref_axis',(-0.707106781186522,2.35364200827643E-16,-0.707106781186573)) ;
#39989=DIRECTION('center_axis',(0.,-1.,0.)) ;
#39990=DIRECTION('ref_axis',(-1.,0.,0.)) ;
#39991=DIRECTION('',(1.66533453692965E-16,1.,1.66321791214593E-16)) ;
#39992=DIRECTION('center_axis',(4.54195640846217E-14,-1.66321791214601E-16,
1.)) ;
#39993=DIRECTION('ref_axis',(1.,0.,-4.54747350886464E-14)) ;
#39994=DIRECTION('center_axis',(-2.1716102378779E-15,3.66854633798134E-28,
1.)) ;
#39995=DIRECTION('ref_axis',(0.707106781186452,0.707106781186643,1.53556032529713E-15)) ;
#39996=DIRECTION('center_axis',(-2.17161023787787E-15,3.6685463379813E-28,
1.)) ;
#39997=DIRECTION('ref_axis',(-0.707106781186552,-0.707106781186543,-1.53556032529732E-15)) ;
#39998=DIRECTION('',(2.17161023787787E-15,-3.6685463379813E-28,-1.)) ;
#39999=DIRECTION('center_axis',(1.88526971141291E-28,-2.90739654573716E-15,
-1.)) ;
#40000=DIRECTION('ref_axis',(1.35627620245787E-13,-1.,2.90739654573716E-15)) ;
#40001=DIRECTION('',(-2.17161023787787E-15,3.6685463379813E-28,1.)) ;
#40002=DIRECTION('center_axis',(-1.,8.32667268460789E-17,-2.17161023787787E-15)) ;
#40003=DIRECTION('ref_axis',(8.32667268460789E-17,1.,-3.92101138914083E-28)) ;
#40004=DIRECTION('',(-2.17161023787787E-15,3.6685463379813E-28,1.)) ;
#40005=DIRECTION('center_axis',(-1.,8.32667268460789E-17,-2.17161023787787E-15)) ;
#40006=DIRECTION('ref_axis',(-1.59443879249779E-15,-0.707106781186479,0.707106781186616)) ;
#40007=DIRECTION('',(8.32667268460789E-17,1.,-3.83780830390118E-28)) ;
#40008=DIRECTION('',(-2.17161023787787E-15,3.83815143260382E-28,1.)) ;
#40009=DIRECTION('',(8.32667268460786E-17,1.,1.66321791214597E-16)) ;
#40010=DIRECTION('',(2.17161023787787E-15,-3.83420712807771E-28,-1.)) ;
#40011=DIRECTION('',(8.32667268460789E-17,1.,-3.83780830390118E-28)) ;
#40012=DIRECTION('center_axis',(-1.,8.32667268460789E-17,-2.17161023787787E-15)) ;
#40013=DIRECTION('ref_axis',(-1.47668185809765E-15,0.707106781186483,0.707106781186612)) ;
#40014=DIRECTION('center_axis',(2.17161023787787E-15,-3.6685463379813E-28,
-1.)) ;
#40015=DIRECTION('ref_axis',(-0.707106781186543,0.707106781186552,-1.53556032529782E-15)) ;
#40016=DIRECTION('',(2.17161023787787E-15,-3.6685463379813E-28,-1.)) ;
#40017=DIRECTION('center_axis',(1.88526971141291E-28,-2.90739654573716E-15,
-1.)) ;
#40018=DIRECTION('ref_axis',(-1.,6.48092690620067E-15,-2.07369595641554E-28)) ;
#40019=DIRECTION('center_axis',(3.33066907386739E-16,1.,-3.66031460022645E-28)) ;
#40020=DIRECTION('ref_axis',(2.17161023787795E-15,-3.66754751528624E-28,
-1.)) ;
#40021=DIRECTION('',(-2.1716102378779E-15,3.66854633798134E-28,1.)) ;
#40022=DIRECTION('',(-1.,3.33066907386739E-16,-2.1716102378779E-15)) ;
#40023=DIRECTION('center_axis',(-1.,3.33066907386739E-16,4.54195640846217E-14)) ;
#40024=DIRECTION('ref_axis',(-3.23519956315716E-14,-0.707106781186623,-0.707106781186472)) ;
#40025=DIRECTION('center_axis',(-1.,0.,0.)) ;
#40026=DIRECTION('ref_axis',(0.,0.,-1.)) ;
#40027=DIRECTION('',(-1.,3.33066907386739E-16,4.54195640846217E-14)) ;
#40028=DIRECTION('center_axis',(1.,0.,0.)) ;
#40029=DIRECTION('ref_axis',(0.,-1.,0.)) ;
#40030=DIRECTION('center_axis',(4.54195640846217E-14,-1.66321791214601E-16,
1.)) ;
#40031=DIRECTION('ref_axis',(1.,0.,-4.54747350886464E-14)) ;
#40032=DIRECTION('center_axis',(0.,1.,0.)) ;
#40033=DIRECTION('ref_axis',(1.,0.,-3.5527136788002E-14)) ;
#40034=DIRECTION('center_axis',(2.17161023787787E-15,-3.6685463379813E-28,
-1.)) ;
#40035=DIRECTION('ref_axis',(-0.707106781186543,0.707106781186552,-1.53556032529782E-15)) ;
#40036=DIRECTION('center_axis',(-8.32667268460786E-17,-1.,-1.66321791214597E-16)) ;
#40037=DIRECTION('ref_axis',(0.707106781186522,5.87287992268709E-17,-0.707106781186573)) ;
#40038=DIRECTION('center_axis',(0.,1.,0.)) ;
#40039=DIRECTION('ref_axis',(1.,0.,0.)) ;
#40040=DIRECTION('',(-8.32667268460786E-17,-1.,-1.66321791214597E-16)) ;
#40041=DIRECTION('center_axis',(4.54195640846217E-14,-1.66321791214601E-16,
1.)) ;
#40042=DIRECTION('ref_axis',(1.,0.,-4.54747350886464E-14)) ;
#40043=DIRECTION('center_axis',(-1.,-2.84217094303975E-13,0.)) ;
#40044=DIRECTION('ref_axis',(-2.84217094303975E-13,1.,0.)) ;
#40045=DIRECTION('center_axis',(-2.17161023787787E-15,3.6685463379813E-28,
1.)) ;
#40046=DIRECTION('ref_axis',(-0.707106781186552,-0.707106781186543,-1.53556032529732E-15)) ;
#40047=DIRECTION('center_axis',(1.,-3.33066907386739E-16,-4.54195640846217E-14)) ;
#40048=DIRECTION('ref_axis',(-3.18809678939767E-14,0.707106781186422,-0.707106781186673)) ;
#40049=DIRECTION('center_axis',(-1.,0.,0.)) ;
#40050=DIRECTION('ref_axis',(0.,1.,0.)) ;
#40051=DIRECTION('',(1.,-3.33066907386739E-16,-4.54195640846217E-14)) ;
#40052=DIRECTION('center_axis',(4.54195640846217E-14,-1.66321791214601E-16,
1.)) ;
#40053=DIRECTION('ref_axis',(1.,0.,-4.54747350886464E-14)) ;
#40054=DIRECTION('center_axis',(0.,-1.,0.)) ;
#40055=DIRECTION('ref_axis',(-1.,0.,3.5527136788007E-14)) ;
#40056=DIRECTION('center_axis',(2.1716102378779E-15,-3.66854633798134E-28,
-1.)) ;
#40057=DIRECTION('ref_axis',(0.707106781186543,-0.707106781186552,1.53556032529784E-15)) ;
#40058=DIRECTION('center_axis',(1.66533453692965E-16,1.,1.66321791214593E-16)) ;
#40059=DIRECTION('ref_axis',(-0.707106781186522,2.35364200827643E-16,-0.707106781186573)) ;
#40060=DIRECTION('center_axis',(0.,-1.,0.)) ;
#40061=DIRECTION('ref_axis',(-1.,0.,0.)) ;
#40062=DIRECTION('',(1.66533453692965E-16,1.,1.66321791214593E-16)) ;
#40063=DIRECTION('center_axis',(4.54195640846217E-14,-1.66321791214601E-16,
1.)) ;
#40064=DIRECTION('ref_axis',(1.,0.,-4.54747350886464E-14)) ;
#40065=DIRECTION('center_axis',(-2.1716102378779E-15,3.66854633798134E-28,
1.)) ;
#40066=DIRECTION('ref_axis',(0.707106781186452,0.707106781186643,1.53556032529713E-15)) ;
#40067=DIRECTION('center_axis',(-2.17161023787787E-15,3.6685463379813E-28,
1.)) ;
#40068=DIRECTION('ref_axis',(-0.707106781186552,-0.707106781186543,-1.53556032529732E-15)) ;
#40069=DIRECTION('',(2.17161023787787E-15,-3.6685463379813E-28,-1.)) ;
#40070=DIRECTION('center_axis',(1.88526971141291E-28,-2.90739654573716E-15,
-1.)) ;
#40071=DIRECTION('ref_axis',(1.35627620245787E-13,-1.,2.90739654573716E-15)) ;
#40072=DIRECTION('',(-2.17161023787787E-15,3.6685463379813E-28,1.)) ;
#40073=DIRECTION('center_axis',(-1.,8.32667268460789E-17,-2.17161023787787E-15)) ;
#40074=DIRECTION('ref_axis',(8.32667268460789E-17,1.,-3.92101138914083E-28)) ;
#40075=DIRECTION('',(-2.17161023787787E-15,3.6685463379813E-28,1.)) ;
#40076=DIRECTION('center_axis',(-1.,8.32667268460789E-17,-2.17161023787787E-15)) ;
#40077=DIRECTION('ref_axis',(-1.59443879249779E-15,-0.707106781186479,0.707106781186616)) ;
#40078=DIRECTION('',(8.32667268460789E-17,1.,-3.83780830390118E-28)) ;
#40079=DIRECTION('',(-2.17161023787787E-15,3.83815143260382E-28,1.)) ;
#40080=DIRECTION('',(8.32667268460786E-17,1.,1.66321791214597E-16)) ;
#40081=DIRECTION('',(2.17161023787787E-15,-3.83420712807771E-28,-1.)) ;
#40082=DIRECTION('',(8.32667268460789E-17,1.,-3.83780830390118E-28)) ;
#40083=DIRECTION('center_axis',(-1.,8.32667268460789E-17,-2.17161023787787E-15)) ;
#40084=DIRECTION('ref_axis',(-1.47668185809765E-15,0.707106781186483,0.707106781186612)) ;
#40085=DIRECTION('center_axis',(2.17161023787787E-15,-3.6685463379813E-28,
-1.)) ;
#40086=DIRECTION('ref_axis',(-0.707106781186543,0.707106781186552,-1.53556032529782E-15)) ;
#40087=DIRECTION('',(2.17161023787787E-15,-3.6685463379813E-28,-1.)) ;
#40088=DIRECTION('center_axis',(1.88526971141291E-28,-2.90739654573716E-15,
-1.)) ;
#40089=DIRECTION('ref_axis',(-1.,6.48092690620067E-15,-2.07369595641554E-28)) ;
#40090=DIRECTION('center_axis',(3.33066907386739E-16,1.,-3.66031460022645E-28)) ;
#40091=DIRECTION('ref_axis',(2.17161023787795E-15,-3.66754751528624E-28,
-1.)) ;
#40092=DIRECTION('',(-2.1716102378779E-15,3.66854633798134E-28,1.)) ;
#40093=DIRECTION('',(-1.,3.33066907386739E-16,-2.1716102378779E-15)) ;
#40094=DIRECTION('center_axis',(-1.,3.33066907386739E-16,4.54195640846217E-14)) ;
#40095=DIRECTION('ref_axis',(-3.23519956315716E-14,-0.707106781186623,-0.707106781186472)) ;
#40096=DIRECTION('center_axis',(-1.,0.,0.)) ;
#40097=DIRECTION('ref_axis',(0.,0.,-1.)) ;
#40098=DIRECTION('',(-1.,3.33066907386739E-16,4.54195640846217E-14)) ;
#40099=DIRECTION('center_axis',(1.,0.,0.)) ;
#40100=DIRECTION('ref_axis',(0.,-1.,0.)) ;
#40101=DIRECTION('center_axis',(4.54195640846217E-14,-1.66321791214601E-16,
1.)) ;
#40102=DIRECTION('ref_axis',(1.,0.,-4.54747350886464E-14)) ;
#40103=DIRECTION('center_axis',(0.,1.,0.)) ;
#40104=DIRECTION('ref_axis',(1.,0.,-3.5527136788002E-14)) ;
#40105=DIRECTION('center_axis',(2.17161023787787E-15,-3.6685463379813E-28,
-1.)) ;
#40106=DIRECTION('ref_axis',(-0.707106781186543,0.707106781186552,-1.53556032529782E-15)) ;
#40107=DIRECTION('center_axis',(-8.32667268460786E-17,-1.,-1.66321791214597E-16)) ;
#40108=DIRECTION('ref_axis',(0.707106781186522,5.87287992268709E-17,-0.707106781186573)) ;
#40109=DIRECTION('center_axis',(0.,1.,0.)) ;
#40110=DIRECTION('ref_axis',(1.,0.,0.)) ;
#40111=DIRECTION('',(-8.32667268460786E-17,-1.,-1.66321791214597E-16)) ;
#40112=DIRECTION('center_axis',(4.54195640846217E-14,-1.66321791214601E-16,
1.)) ;
#40113=DIRECTION('ref_axis',(1.,0.,-4.54747350886464E-14)) ;
#40114=DIRECTION('center_axis',(-1.,-2.84217094303975E-13,0.)) ;
#40115=DIRECTION('ref_axis',(-2.84217094303975E-13,1.,0.)) ;
#40116=DIRECTION('center_axis',(-2.17161023787787E-15,3.6685463379813E-28,
1.)) ;
#40117=DIRECTION('ref_axis',(-0.707106781186552,-0.707106781186543,-1.53556032529732E-15)) ;
#40118=DIRECTION('center_axis',(1.,-3.33066907386739E-16,-4.54195640846217E-14)) ;
#40119=DIRECTION('ref_axis',(-3.18809678939767E-14,0.707106781186422,-0.707106781186673)) ;
#40120=DIRECTION('center_axis',(-1.,0.,0.)) ;
#40121=DIRECTION('ref_axis',(0.,1.,0.)) ;
#40122=DIRECTION('',(1.,-3.33066907386739E-16,-4.54195640846217E-14)) ;
#40123=DIRECTION('center_axis',(4.54195640846217E-14,-1.66321791214601E-16,
1.)) ;
#40124=DIRECTION('ref_axis',(1.,0.,-4.54747350886464E-14)) ;
#40125=DIRECTION('center_axis',(0.,-1.,0.)) ;
#40126=DIRECTION('ref_axis',(-1.,0.,3.5527136788007E-14)) ;
#40127=DIRECTION('center_axis',(2.1716102378779E-15,-3.66854633798134E-28,
-1.)) ;
#40128=DIRECTION('ref_axis',(0.707106781186543,-0.707106781186552,1.53556032529784E-15)) ;
#40129=DIRECTION('center_axis',(1.66533453692965E-16,1.,1.66321791214593E-16)) ;
#40130=DIRECTION('ref_axis',(-0.707106781186522,2.35364200827643E-16,-0.707106781186573)) ;
#40131=DIRECTION('center_axis',(0.,-1.,0.)) ;
#40132=DIRECTION('ref_axis',(-1.,0.,0.)) ;
#40133=DIRECTION('',(1.66533453692965E-16,1.,1.66321791214593E-16)) ;
#40134=DIRECTION('center_axis',(4.54195640846217E-14,-1.66321791214601E-16,
1.)) ;
#40135=DIRECTION('ref_axis',(1.,0.,-4.54747350886464E-14)) ;
#40136=DIRECTION('center_axis',(-2.1716102378779E-15,3.66854633798134E-28,
1.)) ;
#40137=DIRECTION('ref_axis',(0.707106781186452,0.707106781186643,1.53556032529713E-15)) ;
#40138=DIRECTION('center_axis',(-2.17161023787787E-15,3.6685463379813E-28,
1.)) ;
#40139=DIRECTION('ref_axis',(-0.707106781186552,-0.707106781186543,-1.53556032529732E-15)) ;
#40140=DIRECTION('',(2.17161023787787E-15,-3.6685463379813E-28,-1.)) ;
#40141=DIRECTION('center_axis',(1.88526971141291E-28,-2.90739654573716E-15,
-1.)) ;
#40142=DIRECTION('ref_axis',(1.35627620245787E-13,-1.,2.90739654573716E-15)) ;
#40143=DIRECTION('',(-2.17161023787787E-15,3.6685463379813E-28,1.)) ;
#40144=DIRECTION('center_axis',(-1.,8.32667268460789E-17,-2.17161023787787E-15)) ;
#40145=DIRECTION('ref_axis',(8.32667268460789E-17,1.,-3.92101138914083E-28)) ;
#40146=DIRECTION('',(-2.17161023787787E-15,3.6685463379813E-28,1.)) ;
#40147=DIRECTION('center_axis',(-1.,8.32667268460789E-17,-2.17161023787787E-15)) ;
#40148=DIRECTION('ref_axis',(-1.59443879249779E-15,-0.707106781186479,0.707106781186616)) ;
#40149=DIRECTION('',(8.32667268460789E-17,1.,-3.83780830390118E-28)) ;
#40150=DIRECTION('',(-2.17161023787787E-15,3.83815143260382E-28,1.)) ;
#40151=DIRECTION('',(8.32667268460786E-17,1.,1.66321791214597E-16)) ;
#40152=DIRECTION('',(2.17161023787787E-15,-3.83420712807771E-28,-1.)) ;
#40153=DIRECTION('',(8.32667268460789E-17,1.,-3.83780830390118E-28)) ;
#40154=DIRECTION('center_axis',(-1.,8.32667268460789E-17,-2.17161023787787E-15)) ;
#40155=DIRECTION('ref_axis',(-1.47668185809765E-15,0.707106781186483,0.707106781186612)) ;
#40156=DIRECTION('center_axis',(2.17161023787787E-15,-3.6685463379813E-28,
-1.)) ;
#40157=DIRECTION('ref_axis',(-0.707106781186543,0.707106781186552,-1.53556032529782E-15)) ;
#40158=DIRECTION('',(2.17161023787787E-15,-3.6685463379813E-28,-1.)) ;
#40159=DIRECTION('center_axis',(1.88526971141291E-28,-2.90739654573716E-15,
-1.)) ;
#40160=DIRECTION('ref_axis',(-1.,6.48092690620067E-15,-2.07369595641554E-28)) ;
#40161=DIRECTION('center_axis',(3.33066907386739E-16,1.,-3.66031460022645E-28)) ;
#40162=DIRECTION('ref_axis',(2.17161023787795E-15,-3.66754751528624E-28,
-1.)) ;
#40163=DIRECTION('',(-2.1716102378779E-15,3.66854633798134E-28,1.)) ;
#40164=DIRECTION('',(-1.,3.33066907386739E-16,-2.1716102378779E-15)) ;
#40165=DIRECTION('center_axis',(-1.,3.33066907386739E-16,4.54195640846217E-14)) ;
#40166=DIRECTION('ref_axis',(-3.23519956315716E-14,-0.707106781186623,-0.707106781186472)) ;
#40167=DIRECTION('center_axis',(-1.,0.,0.)) ;
#40168=DIRECTION('ref_axis',(0.,0.,-1.)) ;
#40169=DIRECTION('',(-1.,3.33066907386739E-16,4.54195640846217E-14)) ;
#40170=DIRECTION('center_axis',(1.,0.,0.)) ;
#40171=DIRECTION('ref_axis',(0.,-1.,0.)) ;
#40172=DIRECTION('center_axis',(4.54195640846217E-14,-1.66321791214601E-16,
1.)) ;
#40173=DIRECTION('ref_axis',(1.,0.,-4.54747350886464E-14)) ;
#40174=DIRECTION('center_axis',(0.,1.,0.)) ;
#40175=DIRECTION('ref_axis',(1.,0.,-3.5527136788002E-14)) ;
#40176=DIRECTION('center_axis',(2.17161023787787E-15,-3.6685463379813E-28,
-1.)) ;
#40177=DIRECTION('ref_axis',(-0.707106781186543,0.707106781186552,-1.53556032529782E-15)) ;
#40178=DIRECTION('center_axis',(-8.32667268460786E-17,-1.,-1.66321791214597E-16)) ;
#40179=DIRECTION('ref_axis',(0.707106781186522,5.87287992268709E-17,-0.707106781186573)) ;
#40180=DIRECTION('center_axis',(0.,1.,0.)) ;
#40181=DIRECTION('ref_axis',(1.,0.,0.)) ;
#40182=DIRECTION('',(-8.32667268460786E-17,-1.,-1.66321791214597E-16)) ;
#40183=DIRECTION('center_axis',(4.54195640846217E-14,-1.66321791214601E-16,
1.)) ;
#40184=DIRECTION('ref_axis',(1.,0.,-4.54747350886464E-14)) ;
#40185=DIRECTION('center_axis',(-1.,-2.84217094303975E-13,0.)) ;
#40186=DIRECTION('ref_axis',(-2.84217094303975E-13,1.,0.)) ;
#40187=DIRECTION('center_axis',(-2.17161023787787E-15,3.6685463379813E-28,
1.)) ;
#40188=DIRECTION('ref_axis',(-0.707106781186552,-0.707106781186543,-1.53556032529732E-15)) ;
#40189=DIRECTION('center_axis',(1.,-3.33066907386739E-16,-4.54195640846217E-14)) ;
#40190=DIRECTION('ref_axis',(-3.18809678939767E-14,0.707106781186422,-0.707106781186673)) ;
#40191=DIRECTION('center_axis',(-1.,0.,0.)) ;
#40192=DIRECTION('ref_axis',(0.,1.,0.)) ;
#40193=DIRECTION('',(1.,-3.33066907386739E-16,-4.54195640846217E-14)) ;
#40194=DIRECTION('center_axis',(4.54195640846217E-14,-1.66321791214601E-16,
1.)) ;
#40195=DIRECTION('ref_axis',(1.,0.,-4.54747350886464E-14)) ;
#40196=DIRECTION('center_axis',(0.,-1.,0.)) ;
#40197=DIRECTION('ref_axis',(-1.,0.,3.5527136788007E-14)) ;
#40198=DIRECTION('center_axis',(2.1716102378779E-15,-3.66854633798134E-28,
-1.)) ;
#40199=DIRECTION('ref_axis',(0.707106781186543,-0.707106781186552,1.53556032529784E-15)) ;
#40200=DIRECTION('center_axis',(1.66533453692965E-16,1.,1.66321791214593E-16)) ;
#40201=DIRECTION('ref_axis',(-0.707106781186522,2.35364200827643E-16,-0.707106781186573)) ;
#40202=DIRECTION('center_axis',(0.,-1.,0.)) ;
#40203=DIRECTION('ref_axis',(-1.,0.,0.)) ;
#40204=DIRECTION('',(1.66533453692965E-16,1.,1.66321791214593E-16)) ;
#40205=DIRECTION('center_axis',(4.54195640846217E-14,-1.66321791214601E-16,
1.)) ;
#40206=DIRECTION('ref_axis',(1.,0.,-4.54747350886464E-14)) ;
#40207=DIRECTION('center_axis',(-2.1716102378779E-15,3.66854633798134E-28,
1.)) ;
#40208=DIRECTION('ref_axis',(0.707106781186452,0.707106781186643,1.53556032529713E-15)) ;
#40209=DIRECTION('center_axis',(-2.17161023787787E-15,3.6685463379813E-28,
1.)) ;
#40210=DIRECTION('ref_axis',(-0.707106781186552,-0.707106781186543,-1.53556032529732E-15)) ;
#40211=DIRECTION('',(2.17161023787787E-15,-3.6685463379813E-28,-1.)) ;
#40212=DIRECTION('center_axis',(1.88526971141291E-28,-2.90739654573716E-15,
-1.)) ;
#40213=DIRECTION('ref_axis',(1.35627620245787E-13,-1.,2.90739654573716E-15)) ;
#40214=DIRECTION('',(-2.17161023787787E-15,3.6685463379813E-28,1.)) ;
#40215=DIRECTION('center_axis',(-1.,8.32667268460789E-17,-2.17161023787787E-15)) ;
#40216=DIRECTION('ref_axis',(8.32667268460789E-17,1.,-3.92101138914083E-28)) ;
#40217=DIRECTION('',(-2.17161023787787E-15,3.6685463379813E-28,1.)) ;
#40218=DIRECTION('center_axis',(-1.,8.32667268460789E-17,-2.17161023787787E-15)) ;
#40219=DIRECTION('ref_axis',(-1.59443879249779E-15,-0.707106781186479,0.707106781186616)) ;
#40220=DIRECTION('',(8.32667268460789E-17,1.,-3.83780830390118E-28)) ;
#40221=DIRECTION('',(-2.17161023787787E-15,3.83815143260382E-28,1.)) ;
#40222=DIRECTION('',(8.32667268460786E-17,1.,1.66321791214597E-16)) ;
#40223=DIRECTION('',(2.17161023787787E-15,-3.83420712807771E-28,-1.)) ;
#40224=DIRECTION('',(8.32667268460789E-17,1.,-3.83780830390118E-28)) ;
#40225=DIRECTION('center_axis',(-1.,8.32667268460789E-17,-2.17161023787787E-15)) ;
#40226=DIRECTION('ref_axis',(-1.47668185809765E-15,0.707106781186483,0.707106781186612)) ;
#40227=DIRECTION('center_axis',(2.17161023787787E-15,-3.6685463379813E-28,
-1.)) ;
#40228=DIRECTION('ref_axis',(-0.707106781186543,0.707106781186552,-1.53556032529782E-15)) ;
#40229=DIRECTION('',(2.17161023787787E-15,-3.6685463379813E-28,-1.)) ;
#40230=DIRECTION('center_axis',(1.88526971141291E-28,-2.90739654573716E-15,
-1.)) ;
#40231=DIRECTION('ref_axis',(-1.,6.48092690620067E-15,-2.07369595641554E-28)) ;
#40232=DIRECTION('center_axis',(3.33066907386739E-16,1.,-3.66031460022645E-28)) ;
#40233=DIRECTION('ref_axis',(2.17161023787795E-15,-3.66754751528624E-28,
-1.)) ;
#40234=DIRECTION('',(-2.1716102378779E-15,3.66854633798134E-28,1.)) ;
#40235=DIRECTION('',(-1.,3.33066907386739E-16,-2.1716102378779E-15)) ;
#40236=DIRECTION('center_axis',(-1.,3.33066907386739E-16,4.54195640846217E-14)) ;
#40237=DIRECTION('ref_axis',(-3.23519956315716E-14,-0.707106781186623,-0.707106781186472)) ;
#40238=DIRECTION('center_axis',(-1.,0.,0.)) ;
#40239=DIRECTION('ref_axis',(0.,0.,-1.)) ;
#40240=DIRECTION('',(-1.,3.33066907386739E-16,4.54195640846217E-14)) ;
#40241=DIRECTION('center_axis',(1.,0.,0.)) ;
#40242=DIRECTION('ref_axis',(0.,-1.,0.)) ;
#40243=DIRECTION('center_axis',(4.54195640846217E-14,-1.66321791214601E-16,
1.)) ;
#40244=DIRECTION('ref_axis',(1.,0.,-4.54747350886464E-14)) ;
#40245=DIRECTION('center_axis',(0.,1.,0.)) ;
#40246=DIRECTION('ref_axis',(1.,0.,-3.5527136788002E-14)) ;
#40247=DIRECTION('center_axis',(2.17161023787787E-15,-3.6685463379813E-28,
-1.)) ;
#40248=DIRECTION('ref_axis',(-0.707106781186543,0.707106781186552,-1.53556032529782E-15)) ;
#40249=DIRECTION('center_axis',(-8.32667268460786E-17,-1.,-1.66321791214597E-16)) ;
#40250=DIRECTION('ref_axis',(0.707106781186522,5.87287992268709E-17,-0.707106781186573)) ;
#40251=DIRECTION('center_axis',(0.,1.,0.)) ;
#40252=DIRECTION('ref_axis',(1.,0.,0.)) ;
#40253=DIRECTION('',(-8.32667268460786E-17,-1.,-1.66321791214597E-16)) ;
#40254=DIRECTION('center_axis',(4.54195640846217E-14,-1.66321791214601E-16,
1.)) ;
#40255=DIRECTION('ref_axis',(1.,0.,-4.54747350886464E-14)) ;
#40256=DIRECTION('center_axis',(-1.,-2.84217094303975E-13,0.)) ;
#40257=DIRECTION('ref_axis',(-2.84217094303975E-13,1.,0.)) ;
#40258=DIRECTION('center_axis',(-2.17161023787787E-15,3.6685463379813E-28,
1.)) ;
#40259=DIRECTION('ref_axis',(-0.707106781186552,-0.707106781186543,-1.53556032529732E-15)) ;
#40260=DIRECTION('center_axis',(1.,-3.33066907386739E-16,-4.54195640846217E-14)) ;
#40261=DIRECTION('ref_axis',(-3.18809678939767E-14,0.707106781186422,-0.707106781186673)) ;
#40262=DIRECTION('center_axis',(-1.,0.,0.)) ;
#40263=DIRECTION('ref_axis',(0.,1.,0.)) ;
#40264=DIRECTION('',(1.,-3.33066907386739E-16,-4.54195640846217E-14)) ;
#40265=DIRECTION('center_axis',(4.54195640846217E-14,-1.66321791214601E-16,
1.)) ;
#40266=DIRECTION('ref_axis',(1.,0.,-4.54747350886464E-14)) ;
#40267=DIRECTION('center_axis',(0.,-1.,0.)) ;
#40268=DIRECTION('ref_axis',(-1.,0.,3.5527136788007E-14)) ;
#40269=DIRECTION('center_axis',(2.1716102378779E-15,-3.66854633798134E-28,
-1.)) ;
#40270=DIRECTION('ref_axis',(0.707106781186543,-0.707106781186552,1.53556032529784E-15)) ;
#40271=DIRECTION('center_axis',(1.66533453692965E-16,1.,1.66321791214593E-16)) ;
#40272=DIRECTION('ref_axis',(-0.707106781186522,2.35364200827643E-16,-0.707106781186573)) ;
#40273=DIRECTION('center_axis',(0.,-1.,0.)) ;
#40274=DIRECTION('ref_axis',(-1.,0.,0.)) ;
#40275=DIRECTION('',(1.66533453692965E-16,1.,1.66321791214593E-16)) ;
#40276=DIRECTION('center_axis',(4.54195640846217E-14,-1.66321791214601E-16,
1.)) ;
#40277=DIRECTION('ref_axis',(1.,0.,-4.54747350886464E-14)) ;
#40278=DIRECTION('center_axis',(-2.1716102378779E-15,3.66854633798134E-28,
1.)) ;
#40279=DIRECTION('ref_axis',(0.707106781186452,0.707106781186643,1.53556032529713E-15)) ;
#40280=DIRECTION('center_axis',(-2.17161023787787E-15,3.6685463379813E-28,
1.)) ;
#40281=DIRECTION('ref_axis',(-0.707106781186552,-0.707106781186543,-1.53556032529732E-15)) ;
#40282=DIRECTION('',(2.17161023787787E-15,-3.6685463379813E-28,-1.)) ;
#40283=DIRECTION('center_axis',(1.88526971141291E-28,-2.90739654573716E-15,
-1.)) ;
#40284=DIRECTION('ref_axis',(1.35627620245787E-13,-1.,2.90739654573716E-15)) ;
#40285=DIRECTION('',(-2.17161023787787E-15,3.6685463379813E-28,1.)) ;
#40286=DIRECTION('center_axis',(-1.,8.32667268460789E-17,-2.17161023787787E-15)) ;
#40287=DIRECTION('ref_axis',(8.32667268460789E-17,1.,-3.92101138914083E-28)) ;
#40288=DIRECTION('',(-2.17161023787787E-15,3.6685463379813E-28,1.)) ;
#40289=DIRECTION('center_axis',(-1.,8.32667268460789E-17,-2.17161023787787E-15)) ;
#40290=DIRECTION('ref_axis',(-1.59443879249779E-15,-0.707106781186479,0.707106781186616)) ;
#40291=DIRECTION('',(8.32667268460789E-17,1.,-3.83780830390118E-28)) ;
#40292=DIRECTION('',(-2.17161023787787E-15,3.83815143260382E-28,1.)) ;
#40293=DIRECTION('',(8.32667268460786E-17,1.,1.66321791214597E-16)) ;
#40294=DIRECTION('',(2.17161023787787E-15,-3.83420712807771E-28,-1.)) ;
#40295=DIRECTION('',(8.32667268460789E-17,1.,-3.83780830390118E-28)) ;
#40296=DIRECTION('center_axis',(-1.,8.32667268460789E-17,-2.17161023787787E-15)) ;
#40297=DIRECTION('ref_axis',(-1.47668185809765E-15,0.707106781186483,0.707106781186612)) ;
#40298=DIRECTION('center_axis',(2.17161023787787E-15,-3.6685463379813E-28,
-1.)) ;
#40299=DIRECTION('ref_axis',(-0.707106781186543,0.707106781186552,-1.53556032529782E-15)) ;
#40300=DIRECTION('',(2.17161023787787E-15,-3.6685463379813E-28,-1.)) ;
#40301=DIRECTION('center_axis',(1.88526971141291E-28,-2.90739654573716E-15,
-1.)) ;
#40302=DIRECTION('ref_axis',(-1.,6.48092690620067E-15,-2.07369595641554E-28)) ;
#40303=DIRECTION('center_axis',(3.33066907386739E-16,1.,-3.66031460022645E-28)) ;
#40304=DIRECTION('ref_axis',(2.17161023787795E-15,-3.66754751528624E-28,
-1.)) ;
#40305=DIRECTION('',(-2.1716102378779E-15,3.66854633798134E-28,1.)) ;
#40306=DIRECTION('',(-1.,3.33066907386739E-16,-2.1716102378779E-15)) ;
#40307=DIRECTION('center_axis',(-1.,3.33066907386739E-16,4.54195640846217E-14)) ;
#40308=DIRECTION('ref_axis',(-3.23519956315716E-14,-0.707106781186623,-0.707106781186472)) ;
#40309=DIRECTION('center_axis',(-1.,0.,0.)) ;
#40310=DIRECTION('ref_axis',(0.,0.,-1.)) ;
#40311=DIRECTION('',(-1.,3.33066907386739E-16,4.54195640846217E-14)) ;
#40312=DIRECTION('center_axis',(1.,0.,0.)) ;
#40313=DIRECTION('ref_axis',(0.,-1.,0.)) ;
#40314=DIRECTION('center_axis',(4.54195640846217E-14,-1.66321791214601E-16,
1.)) ;
#40315=DIRECTION('ref_axis',(1.,0.,-4.54747350886464E-14)) ;
#40316=DIRECTION('center_axis',(0.,1.,0.)) ;
#40317=DIRECTION('ref_axis',(1.,0.,-3.5527136788002E-14)) ;
#40318=DIRECTION('center_axis',(4.54195640846217E-14,-1.66321791214601E-16,
1.)) ;
#40319=DIRECTION('ref_axis',(-0.707106781186502,0.707106781186593,3.22340890291979E-14)) ;
#40320=DIRECTION('center_axis',(-8.32667268460786E-17,-1.,-1.66321791214597E-16)) ;
#40321=DIRECTION('ref_axis',(0.707106781186522,5.87287992268709E-17,-0.707106781186573)) ;
#40322=DIRECTION('center_axis',(0.,1.,0.)) ;
#40323=DIRECTION('ref_axis',(1.,0.,0.)) ;
#40324=DIRECTION('',(-8.32667268460786E-17,-1.,-1.66321791214597E-16)) ;
#40325=DIRECTION('center_axis',(4.54195640846217E-14,-1.66321791214601E-16,
1.)) ;
#40326=DIRECTION('ref_axis',(1.,0.,-4.54747350886464E-14)) ;
#40327=DIRECTION('center_axis',(-1.,-2.84217094303975E-13,0.)) ;
#40328=DIRECTION('ref_axis',(-2.84217094303975E-13,1.,0.)) ;
#40329=DIRECTION('center_axis',(4.54195640846217E-14,-1.66321791214601E-16,
1.)) ;
#40330=DIRECTION('ref_axis',(-0.707106781186502,-0.707106781186593,3.1998874496344E-14)) ;
#40331=DIRECTION('center_axis',(1.,-3.33066907386739E-16,-4.54195640846217E-14)) ;
#40332=DIRECTION('ref_axis',(-3.18809678939767E-14,0.707106781186422,-0.707106781186673)) ;
#40333=DIRECTION('center_axis',(-1.,0.,0.)) ;
#40334=DIRECTION('ref_axis',(0.,1.,0.)) ;
#40335=DIRECTION('',(1.,-3.33066907386739E-16,-4.54195640846217E-14)) ;
#40336=DIRECTION('center_axis',(4.54195640846217E-14,-1.66321791214601E-16,
1.)) ;
#40337=DIRECTION('ref_axis',(1.,0.,-4.54747350886464E-14)) ;
#40338=DIRECTION('center_axis',(0.,-1.,0.)) ;
#40339=DIRECTION('ref_axis',(-1.,0.,3.5527136788007E-14)) ;
#40340=DIRECTION('center_axis',(4.54195640846217E-14,-1.66321791214601E-16,
1.)) ;
#40341=DIRECTION('ref_axis',(0.707106781186593,-0.707106781186502,-3.2234089029202E-14)) ;
#40342=DIRECTION('center_axis',(1.66533453692965E-16,1.,1.66321791214593E-16)) ;
#40343=DIRECTION('ref_axis',(-0.707106781186522,2.35364200827643E-16,-0.707106781186573)) ;
#40344=DIRECTION('center_axis',(0.,-1.,0.)) ;
#40345=DIRECTION('ref_axis',(-1.,0.,0.)) ;
#40346=DIRECTION('',(1.66533453692965E-16,1.,1.66321791214593E-16)) ;
#40347=DIRECTION('center_axis',(4.54195640846217E-14,-1.66321791214601E-16,
1.)) ;
#40348=DIRECTION('ref_axis',(1.,0.,-4.54747350886464E-14)) ;
#40349=DIRECTION('center_axis',(4.54195640846217E-14,-1.66321791214601E-16,
1.)) ;
#40350=DIRECTION('ref_axis',(0.707106781186593,0.707106781186502,-3.19988744963481E-14)) ;
#40351=DIRECTION('center_axis',(-2.17161023787787E-15,3.6685463379813E-28,
1.)) ;
#40352=DIRECTION('ref_axis',(-0.707106781186552,-0.707106781186543,-1.53556032529732E-15)) ;
#40353=DIRECTION('',(2.17161023787787E-15,-3.6685463379813E-28,-1.)) ;
#40354=DIRECTION('center_axis',(1.88526971141291E-28,-2.90739654573716E-15,
-1.)) ;
#40355=DIRECTION('ref_axis',(1.35627620245787E-13,-1.,2.90739654573716E-15)) ;
#40356=DIRECTION('',(-2.17161023787787E-15,3.6685463379813E-28,1.)) ;
#40357=DIRECTION('center_axis',(-1.,8.32667268460789E-17,-2.17161023787787E-15)) ;
#40358=DIRECTION('ref_axis',(8.32667268460789E-17,1.,-3.92101138914083E-28)) ;
#40359=DIRECTION('',(8.32667268460786E-17,1.,1.66321791214597E-16)) ;
#40360=DIRECTION('',(2.17161023787787E-15,-3.83420712807771E-28,-1.)) ;
#40361=DIRECTION('',(8.32667268460789E-17,1.,-3.83780830390118E-28)) ;
#40362=DIRECTION('center_axis',(-1.,8.32667268460789E-17,-2.17161023787787E-15)) ;
#40363=DIRECTION('ref_axis',(-1.47668185809765E-15,0.707106781186483,0.707106781186612)) ;
#40364=DIRECTION('',(-2.17161023787787E-15,3.6685463379813E-28,1.)) ;
#40365=DIRECTION('center_axis',(-1.,8.32667268460789E-17,-2.17161023787787E-15)) ;
#40366=DIRECTION('ref_axis',(-1.59443879249779E-15,-0.707106781186479,0.707106781186616)) ;
#40367=DIRECTION('',(8.32667268460789E-17,1.,-3.83780830390118E-28)) ;
#40368=DIRECTION('',(-2.17161023787787E-15,3.83815143260382E-28,1.)) ;
#40369=DIRECTION('center_axis',(2.17161023787787E-15,-3.6685463379813E-28,
-1.)) ;
#40370=DIRECTION('ref_axis',(-0.707106781186543,0.707106781186552,-1.53556032529782E-15)) ;
#40371=DIRECTION('',(2.17161023787787E-15,-3.6685463379813E-28,-1.)) ;
#40372=DIRECTION('center_axis',(1.88526971141291E-28,-2.90739654573716E-15,
-1.)) ;
#40373=DIRECTION('ref_axis',(-1.,6.48092690620067E-15,-2.07369595641554E-28)) ;
#40374=DIRECTION('center_axis',(3.33066907386739E-16,1.,-3.66031460022645E-28)) ;
#40375=DIRECTION('ref_axis',(2.17161023787795E-15,-3.66754751528624E-28,
-1.)) ;
#40376=DIRECTION('',(-2.1716102378779E-15,3.66854633798134E-28,1.)) ;
#40377=DIRECTION('',(-1.,3.33066907386739E-16,-2.1716102378779E-15)) ;
#40378=DIRECTION('center_axis',(1.,-1.66533453692966E-16,-4.54195640846217E-14)) ;
#40379=DIRECTION('ref_axis',(3.19987248283774E-14,-0.707106781186434,0.707106781186661)) ;
#40380=DIRECTION('center_axis',(1.,0.,0.)) ;
#40381=DIRECTION('ref_axis',(0.,0.,1.)) ;
#40382=DIRECTION('',(1.,-1.66533453692966E-16,-4.54195640846217E-14)) ;
#40383=DIRECTION('center_axis',(-1.,0.,0.)) ;
#40384=DIRECTION('ref_axis',(0.,-1.,0.)) ;
#40385=DIRECTION('',(1.,-1.66533453692966E-16,-4.54195640846217E-14)) ;
#40386=DIRECTION('center_axis',(-4.54195640846217E-14,1.66321791214601E-16,
-1.)) ;
#40387=DIRECTION('ref_axis',(-1.,0.,4.54747350886464E-14)) ;
#40388=DIRECTION('center_axis',(0.,1.,0.)) ;
#40389=DIRECTION('ref_axis',(-1.,0.,5.32907051820105E-14)) ;
#40390=DIRECTION('center_axis',(4.54195640846217E-14,-1.66321791214601E-16,
1.)) ;
#40391=DIRECTION('ref_axis',(-1.,5.55236256206829E-46,4.54195640846217E-14)) ;
#40392=DIRECTION('center_axis',(2.17161023787787E-15,-3.83815143260382E-28,
-1.)) ;
#40393=DIRECTION('ref_axis',(0.707106781186452,0.707106781186643,1.53556032529709E-15)) ;
#40394=DIRECTION('center_axis',(-8.32667268460786E-17,-1.,-1.66321791214597E-16)) ;
#40395=DIRECTION('ref_axis',(-0.707106781186535,-5.87287992268677E-17,0.70710678118656)) ;
#40396=DIRECTION('center_axis',(0.,1.,0.)) ;
#40397=DIRECTION('ref_axis',(-1.,0.,0.)) ;
#40398=DIRECTION('',(-8.32667268460786E-17,-1.,-1.66321791214597E-16)) ;
#40399=DIRECTION('',(-8.32667268460786E-17,-1.,-1.66321791214597E-16)) ;
#40400=DIRECTION('center_axis',(-4.54195640846217E-14,1.66321791214601E-16,
-1.)) ;
#40401=DIRECTION('ref_axis',(-1.,0.,4.54747350886464E-14)) ;
#40402=DIRECTION('center_axis',(1.,2.84217094304056E-13,0.)) ;
#40403=DIRECTION('ref_axis',(-2.84217094304056E-13,1.,0.)) ;
#40404=DIRECTION('center_axis',(4.54195640846217E-14,-1.66321791214601E-16,
1.)) ;
#40405=DIRECTION('ref_axis',(-1.,5.55236256206829E-46,4.54195640846217E-14)) ;
#40406=DIRECTION('center_axis',(-2.17161023787787E-15,3.83420712807771E-28,
1.)) ;
#40407=DIRECTION('ref_axis',(0.707106781186543,-0.707106781186552,1.53556032529783E-15)) ;
#40408=DIRECTION('center_axis',(-1.,1.66533453692587E-16,4.54195640846217E-14)) ;
#40409=DIRECTION('ref_axis',(3.22342386971791E-14,0.707106781186422,0.707106781186673)) ;
#40410=DIRECTION('center_axis',(1.,0.,0.)) ;
#40411=DIRECTION('ref_axis',(0.,1.,0.)) ;
#40412=DIRECTION('',(-1.,1.66533453692587E-16,4.54195640846217E-14)) ;
#40413=DIRECTION('',(-1.,1.66533453692587E-16,4.54195640846217E-14)) ;
#40414=DIRECTION('center_axis',(-4.54195640846217E-14,1.66321791214601E-16,
-1.)) ;
#40415=DIRECTION('ref_axis',(-1.,0.,4.54747350886464E-14)) ;
#40416=DIRECTION('center_axis',(0.,-1.,0.)) ;
#40417=DIRECTION('ref_axis',(1.,0.,-5.32907051820105E-14)) ;
#40418=DIRECTION('center_axis',(4.54195640846217E-14,-1.66321791214601E-16,
1.)) ;
#40419=DIRECTION('ref_axis',(-1.,5.55236256206829E-46,4.54195640846217E-14)) ;
#40420=DIRECTION('center_axis',(2.1716102378779E-15,-3.83420712807775E-28,
-1.)) ;
#40421=DIRECTION('ref_axis',(-0.707106781186452,-0.707106781186643,-1.53556032529712E-15)) ;
#40422=DIRECTION('center_axis',(1.66533453692965E-16,1.,1.66321791214593E-16)) ;
#40423=DIRECTION('ref_axis',(0.707106781186535,-2.35364200827643E-16,0.70710678118656)) ;
#40424=DIRECTION('center_axis',(0.,-1.,0.)) ;
#40425=DIRECTION('ref_axis',(1.,0.,0.)) ;
#40426=DIRECTION('',(1.66533453692965E-16,1.,1.66321791214593E-16)) ;
#40427=DIRECTION('',(1.66533453692965E-16,1.,1.66321791214593E-16)) ;
#40428=DIRECTION('center_axis',(-4.54195640846217E-14,1.66321791214601E-16,
-1.)) ;
#40429=DIRECTION('ref_axis',(-1.,0.,4.54747350886464E-14)) ;
#40430=DIRECTION('center_axis',(4.54195640846217E-14,-1.66321791214601E-16,
1.)) ;
#40431=DIRECTION('ref_axis',(-1.,5.55236256206829E-46,4.54195640846217E-14)) ;
#40432=DIRECTION('center_axis',(-2.1716102378779E-15,3.83815143260386E-28,
1.)) ;
#40433=DIRECTION('ref_axis',(-0.707106781186643,0.707106781186452,-1.53556032529807E-15)) ;
#40434=DIRECTION('center_axis',(-2.17161023787787E-15,3.83420712807771E-28,
1.)) ;
#40435=DIRECTION('ref_axis',(0.707106781186543,-0.707106781186552,1.53556032529783E-15)) ;
#40436=DIRECTION('',(-2.17161023787787E-15,3.83420712807771E-28,1.)) ;
#40437=DIRECTION('center_axis',(2.17161023787792E-15,-2.90739654573749E-15,
-1.)) ;
#40438=DIRECTION('ref_axis',(1.35627620245787E-13,-1.,2.90739654573778E-15)) ;
#40439=DIRECTION('',(2.17161023787787E-15,-3.83420712807771E-28,-1.)) ;
#40440=DIRECTION('center_axis',(1.,-8.32667268460789E-17,2.17161023787787E-15)) ;
#40441=DIRECTION('ref_axis',(-8.32667268460789E-17,-1.,3.92101138914083E-28)) ;
#40442=DIRECTION('',(2.17161023787787E-15,-3.83815143260382E-28,-1.)) ;
#40443=DIRECTION('',(-8.32667268460789E-17,-1.,3.83780830390118E-28)) ;
#40444=DIRECTION('center_axis',(2.17161023787787E-15,-3.83815143260382E-28,
-1.)) ;
#40445=DIRECTION('ref_axis',(0.707106781186452,0.707106781186643,1.53556032529709E-15)) ;
#40446=DIRECTION('',(-2.17161023787787E-15,3.83815143260382E-28,1.)) ;
#40447=DIRECTION('center_axis',(2.17161023787746E-15,-7.39616701217516E-14,
-1.)) ;
#40448=DIRECTION('ref_axis',(1.,-6.48092690624108E-15,2.17161023787794E-15)) ;
#40449=DIRECTION('center_axis',(1.66533453692966E-16,1.,-3.83386399937507E-28)) ;
#40450=DIRECTION('ref_axis',(2.1716102378779E-15,-3.83748045690496E-28,
-1.)) ;
#40451=DIRECTION('',(2.1716102378779E-15,-3.83815143260386E-28,-1.)) ;
#40452=DIRECTION('',(1.,-1.66533453692966E-16,2.1716102378779E-15)) ;
#40453=DIRECTION('center_axis',(1.,-1.66533453692966E-16,-4.54195640846217E-14)) ;
#40454=DIRECTION('ref_axis',(3.19987248283774E-14,-0.707106781186434,0.707106781186661)) ;
#40455=DIRECTION('center_axis',(1.,0.,0.)) ;
#40456=DIRECTION('ref_axis',(0.,0.,1.)) ;
#40457=DIRECTION('',(1.,-1.66533453692966E-16,-4.54195640846217E-14)) ;
#40458=DIRECTION('center_axis',(-1.,0.,0.)) ;
#40459=DIRECTION('ref_axis',(0.,-1.,0.)) ;
#40460=DIRECTION('',(1.,-1.66533453692966E-16,-4.54195640846217E-14)) ;
#40461=DIRECTION('center_axis',(-4.54195640846217E-14,1.66321791214601E-16,
-1.)) ;
#40462=DIRECTION('ref_axis',(-1.,0.,4.54747350886464E-14)) ;
#40463=DIRECTION('center_axis',(0.,1.,0.)) ;
#40464=DIRECTION('ref_axis',(-1.,0.,5.32907051820105E-14)) ;
#40465=DIRECTION('center_axis',(4.54195640846217E-14,-1.66321791214601E-16,
1.)) ;
#40466=DIRECTION('ref_axis',(-1.,5.55236256206829E-46,4.54195640846217E-14)) ;
#40467=DIRECTION('center_axis',(2.17161023787787E-15,-3.83815143260382E-28,
-1.)) ;
#40468=DIRECTION('ref_axis',(0.707106781186452,0.707106781186643,1.53556032529709E-15)) ;
#40469=DIRECTION('center_axis',(-8.32667268460786E-17,-1.,-1.66321791214597E-16)) ;
#40470=DIRECTION('ref_axis',(-0.707106781186535,-5.87287992268677E-17,0.70710678118656)) ;
#40471=DIRECTION('center_axis',(0.,1.,0.)) ;
#40472=DIRECTION('ref_axis',(-1.,0.,0.)) ;
#40473=DIRECTION('',(-8.32667268460786E-17,-1.,-1.66321791214597E-16)) ;
#40474=DIRECTION('',(-8.32667268460786E-17,-1.,-1.66321791214597E-16)) ;
#40475=DIRECTION('center_axis',(-4.54195640846217E-14,1.66321791214601E-16,
-1.)) ;
#40476=DIRECTION('ref_axis',(-1.,0.,4.54747350886464E-14)) ;
#40477=DIRECTION('center_axis',(1.,2.84217094304056E-13,0.)) ;
#40478=DIRECTION('ref_axis',(-2.84217094304056E-13,1.,0.)) ;
#40479=DIRECTION('center_axis',(4.54195640846217E-14,-1.66321791214601E-16,
1.)) ;
#40480=DIRECTION('ref_axis',(-1.,5.55236256206829E-46,4.54195640846217E-14)) ;
#40481=DIRECTION('center_axis',(-2.17161023787787E-15,3.83420712807771E-28,
1.)) ;
#40482=DIRECTION('ref_axis',(0.707106781186543,-0.707106781186552,1.53556032529783E-15)) ;
#40483=DIRECTION('center_axis',(-1.,1.66533453692587E-16,4.54195640846217E-14)) ;
#40484=DIRECTION('ref_axis',(3.22342386971791E-14,0.707106781186422,0.707106781186673)) ;
#40485=DIRECTION('center_axis',(1.,0.,0.)) ;
#40486=DIRECTION('ref_axis',(0.,1.,0.)) ;
#40487=DIRECTION('',(-1.,1.66533453692587E-16,4.54195640846217E-14)) ;
#40488=DIRECTION('',(-1.,1.66533453692587E-16,4.54195640846217E-14)) ;
#40489=DIRECTION('center_axis',(-4.54195640846217E-14,1.66321791214601E-16,
-1.)) ;
#40490=DIRECTION('ref_axis',(-1.,0.,4.54747350886464E-14)) ;
#40491=DIRECTION('center_axis',(0.,-1.,0.)) ;
#40492=DIRECTION('ref_axis',(1.,0.,-5.32907051820105E-14)) ;
#40493=DIRECTION('center_axis',(4.54195640846217E-14,-1.66321791214601E-16,
1.)) ;
#40494=DIRECTION('ref_axis',(-1.,5.55236256206829E-46,4.54195640846217E-14)) ;
#40495=DIRECTION('center_axis',(2.1716102378779E-15,-3.83420712807775E-28,
-1.)) ;
#40496=DIRECTION('ref_axis',(-0.707106781186452,-0.707106781186643,-1.53556032529712E-15)) ;
#40497=DIRECTION('center_axis',(1.66533453692965E-16,1.,1.66321791214593E-16)) ;
#40498=DIRECTION('ref_axis',(0.707106781186535,-2.35364200827643E-16,0.70710678118656)) ;
#40499=DIRECTION('center_axis',(0.,-1.,0.)) ;
#40500=DIRECTION('ref_axis',(1.,0.,0.)) ;
#40501=DIRECTION('',(1.66533453692965E-16,1.,1.66321791214593E-16)) ;
#40502=DIRECTION('',(1.66533453692965E-16,1.,1.66321791214593E-16)) ;
#40503=DIRECTION('center_axis',(-4.54195640846217E-14,1.66321791214601E-16,
-1.)) ;
#40504=DIRECTION('ref_axis',(-1.,0.,4.54747350886464E-14)) ;
#40505=DIRECTION('center_axis',(4.54195640846217E-14,-1.66321791214601E-16,
1.)) ;
#40506=DIRECTION('ref_axis',(-1.,5.55236256206829E-46,4.54195640846217E-14)) ;
#40507=DIRECTION('center_axis',(-2.1716102378779E-15,3.83815143260386E-28,
1.)) ;
#40508=DIRECTION('ref_axis',(-0.707106781186643,0.707106781186452,-1.53556032529807E-15)) ;
#40509=DIRECTION('center_axis',(-2.17161023787787E-15,3.83420712807771E-28,
1.)) ;
#40510=DIRECTION('ref_axis',(0.707106781186543,-0.707106781186552,1.53556032529783E-15)) ;
#40511=DIRECTION('',(-2.17161023787787E-15,3.83420712807771E-28,1.)) ;
#40512=DIRECTION('center_axis',(2.17161023787792E-15,-2.90739654573749E-15,
-1.)) ;
#40513=DIRECTION('ref_axis',(1.35627620245787E-13,-1.,2.90739654573778E-15)) ;
#40514=DIRECTION('',(2.17161023787787E-15,-3.83420712807771E-28,-1.)) ;
#40515=DIRECTION('center_axis',(1.,-8.32667268460789E-17,2.17161023787787E-15)) ;
#40516=DIRECTION('ref_axis',(-8.32667268460789E-17,-1.,3.92101138914083E-28)) ;
#40517=DIRECTION('',(2.17161023787787E-15,-3.83815143260382E-28,-1.)) ;
#40518=DIRECTION('',(-8.32667268460789E-17,-1.,3.83780830390118E-28)) ;
#40519=DIRECTION('center_axis',(2.17161023787787E-15,-3.83815143260382E-28,
-1.)) ;
#40520=DIRECTION('ref_axis',(0.707106781186452,0.707106781186643,1.53556032529709E-15)) ;
#40521=DIRECTION('',(-2.17161023787787E-15,3.83815143260382E-28,1.)) ;
#40522=DIRECTION('center_axis',(2.17161023787746E-15,-7.39616701217516E-14,
-1.)) ;
#40523=DIRECTION('ref_axis',(1.,-6.48092690624108E-15,2.17161023787794E-15)) ;
#40524=DIRECTION('center_axis',(1.66533453692966E-16,1.,-3.83386399937507E-28)) ;
#40525=DIRECTION('ref_axis',(2.1716102378779E-15,-3.83748045690496E-28,
-1.)) ;
#40526=DIRECTION('',(2.1716102378779E-15,-3.83815143260386E-28,-1.)) ;
#40527=DIRECTION('',(1.,-1.66533453692966E-16,2.1716102378779E-15)) ;
#40528=DIRECTION('center_axis',(1.,-1.66533453692966E-16,-4.54195640846217E-14)) ;
#40529=DIRECTION('ref_axis',(3.19987248283774E-14,-0.707106781186434,0.707106781186661)) ;
#40530=DIRECTION('center_axis',(1.,0.,0.)) ;
#40531=DIRECTION('ref_axis',(0.,0.,1.)) ;
#40532=DIRECTION('',(1.,-1.66533453692966E-16,-4.54195640846217E-14)) ;
#40533=DIRECTION('center_axis',(-1.,0.,0.)) ;
#40534=DIRECTION('ref_axis',(0.,-1.,0.)) ;
#40535=DIRECTION('',(1.,-1.66533453692966E-16,-4.54195640846217E-14)) ;
#40536=DIRECTION('center_axis',(-4.54195640846217E-14,1.66321791214601E-16,
-1.)) ;
#40537=DIRECTION('ref_axis',(-1.,0.,4.54747350886464E-14)) ;
#40538=DIRECTION('center_axis',(0.,1.,0.)) ;
#40539=DIRECTION('ref_axis',(-1.,0.,5.32907051820105E-14)) ;
#40540=DIRECTION('center_axis',(4.54195640846217E-14,-1.66321791214601E-16,
1.)) ;
#40541=DIRECTION('ref_axis',(-1.,5.55236256206829E-46,4.54195640846217E-14)) ;
#40542=DIRECTION('center_axis',(2.17161023787787E-15,-3.83815143260382E-28,
-1.)) ;
#40543=DIRECTION('ref_axis',(0.707106781186452,0.707106781186643,1.53556032529709E-15)) ;
#40544=DIRECTION('center_axis',(-8.32667268460786E-17,-1.,-1.66321791214597E-16)) ;
#40545=DIRECTION('ref_axis',(-0.707106781186535,-5.87287992268677E-17,0.70710678118656)) ;
#40546=DIRECTION('center_axis',(0.,1.,0.)) ;
#40547=DIRECTION('ref_axis',(-1.,0.,0.)) ;
#40548=DIRECTION('',(-8.32667268460786E-17,-1.,-1.66321791214597E-16)) ;
#40549=DIRECTION('',(-8.32667268460786E-17,-1.,-1.66321791214597E-16)) ;
#40550=DIRECTION('center_axis',(-4.54195640846217E-14,1.66321791214601E-16,
-1.)) ;
#40551=DIRECTION('ref_axis',(-1.,0.,4.54747350886464E-14)) ;
#40552=DIRECTION('center_axis',(1.,2.84217094304056E-13,0.)) ;
#40553=DIRECTION('ref_axis',(-2.84217094304056E-13,1.,0.)) ;
#40554=DIRECTION('center_axis',(4.54195640846217E-14,-1.66321791214601E-16,
1.)) ;
#40555=DIRECTION('ref_axis',(-1.,5.55236256206829E-46,4.54195640846217E-14)) ;
#40556=DIRECTION('center_axis',(-2.17161023787787E-15,3.83420712807771E-28,
1.)) ;
#40557=DIRECTION('ref_axis',(0.707106781186543,-0.707106781186552,1.53556032529783E-15)) ;
#40558=DIRECTION('center_axis',(-1.,1.66533453692587E-16,4.54195640846217E-14)) ;
#40559=DIRECTION('ref_axis',(3.22342386971791E-14,0.707106781186422,0.707106781186673)) ;
#40560=DIRECTION('center_axis',(1.,0.,0.)) ;
#40561=DIRECTION('ref_axis',(0.,1.,0.)) ;
#40562=DIRECTION('',(-1.,1.66533453692587E-16,4.54195640846217E-14)) ;
#40563=DIRECTION('',(-1.,1.66533453692587E-16,4.54195640846217E-14)) ;
#40564=DIRECTION('center_axis',(-4.54195640846217E-14,1.66321791214601E-16,
-1.)) ;
#40565=DIRECTION('ref_axis',(-1.,0.,4.54747350886464E-14)) ;
#40566=DIRECTION('center_axis',(0.,-1.,0.)) ;
#40567=DIRECTION('ref_axis',(1.,0.,-5.32907051820105E-14)) ;
#40568=DIRECTION('center_axis',(4.54195640846217E-14,-1.66321791214601E-16,
1.)) ;
#40569=DIRECTION('ref_axis',(-1.,5.55236256206829E-46,4.54195640846217E-14)) ;
#40570=DIRECTION('center_axis',(2.1716102378779E-15,-3.83420712807775E-28,
-1.)) ;
#40571=DIRECTION('ref_axis',(-0.707106781186452,-0.707106781186643,-1.53556032529712E-15)) ;
#40572=DIRECTION('center_axis',(1.66533453692965E-16,1.,1.66321791214593E-16)) ;
#40573=DIRECTION('ref_axis',(0.707106781186535,-2.35364200827643E-16,0.70710678118656)) ;
#40574=DIRECTION('center_axis',(0.,-1.,0.)) ;
#40575=DIRECTION('ref_axis',(1.,0.,0.)) ;
#40576=DIRECTION('',(1.66533453692965E-16,1.,1.66321791214593E-16)) ;
#40577=DIRECTION('',(1.66533453692965E-16,1.,1.66321791214593E-16)) ;
#40578=DIRECTION('center_axis',(-4.54195640846217E-14,1.66321791214601E-16,
-1.)) ;
#40579=DIRECTION('ref_axis',(-1.,0.,4.54747350886464E-14)) ;
#40580=DIRECTION('center_axis',(4.54195640846217E-14,-1.66321791214601E-16,
1.)) ;
#40581=DIRECTION('ref_axis',(-1.,5.55236256206829E-46,4.54195640846217E-14)) ;
#40582=DIRECTION('center_axis',(-2.1716102378779E-15,3.83815143260386E-28,
1.)) ;
#40583=DIRECTION('ref_axis',(-0.707106781186643,0.707106781186452,-1.53556032529807E-15)) ;
#40584=DIRECTION('center_axis',(-2.17161023787787E-15,3.83420712807771E-28,
1.)) ;
#40585=DIRECTION('ref_axis',(0.707106781186543,-0.707106781186552,1.53556032529783E-15)) ;
#40586=DIRECTION('',(-2.17161023787787E-15,3.83420712807771E-28,1.)) ;
#40587=DIRECTION('center_axis',(2.17161023787792E-15,-2.90739654573749E-15,
-1.)) ;
#40588=DIRECTION('ref_axis',(1.35627620245787E-13,-1.,2.90739654573778E-15)) ;
#40589=DIRECTION('',(2.17161023787787E-15,-3.83420712807771E-28,-1.)) ;
#40590=DIRECTION('center_axis',(1.,-8.32667268460789E-17,2.17161023787787E-15)) ;
#40591=DIRECTION('ref_axis',(-8.32667268460789E-17,-1.,3.92101138914083E-28)) ;
#40592=DIRECTION('',(2.17161023787787E-15,-3.83815143260382E-28,-1.)) ;
#40593=DIRECTION('',(-8.32667268460789E-17,-1.,3.83780830390118E-28)) ;
#40594=DIRECTION('center_axis',(2.17161023787787E-15,-3.83815143260382E-28,
-1.)) ;
#40595=DIRECTION('ref_axis',(0.707106781186452,0.707106781186643,1.53556032529709E-15)) ;
#40596=DIRECTION('',(-2.17161023787787E-15,3.83815143260382E-28,1.)) ;
#40597=DIRECTION('center_axis',(2.17161023787746E-15,-7.39616701217516E-14,
-1.)) ;
#40598=DIRECTION('ref_axis',(1.,-6.48092690624108E-15,2.17161023787794E-15)) ;
#40599=DIRECTION('center_axis',(1.66533453692966E-16,1.,-3.83386399937507E-28)) ;
#40600=DIRECTION('ref_axis',(2.1716102378779E-15,-3.83748045690496E-28,
-1.)) ;
#40601=DIRECTION('',(2.1716102378779E-15,-3.83815143260386E-28,-1.)) ;
#40602=DIRECTION('',(1.,-1.66533453692966E-16,2.1716102378779E-15)) ;
#40603=DIRECTION('center_axis',(1.,-1.66533453692966E-16,-4.54195640846217E-14)) ;
#40604=DIRECTION('ref_axis',(3.19987248283774E-14,-0.707106781186434,0.707106781186661)) ;
#40605=DIRECTION('center_axis',(1.,0.,0.)) ;
#40606=DIRECTION('ref_axis',(0.,0.,1.)) ;
#40607=DIRECTION('',(1.,-1.66533453692966E-16,-4.54195640846217E-14)) ;
#40608=DIRECTION('center_axis',(-1.,0.,0.)) ;
#40609=DIRECTION('ref_axis',(0.,-1.,0.)) ;
#40610=DIRECTION('',(1.,-1.66533453692966E-16,-4.54195640846217E-14)) ;
#40611=DIRECTION('center_axis',(-4.54195640846217E-14,1.66321791214601E-16,
-1.)) ;
#40612=DIRECTION('ref_axis',(-1.,0.,4.54747350886464E-14)) ;
#40613=DIRECTION('center_axis',(0.,1.,0.)) ;
#40614=DIRECTION('ref_axis',(-1.,0.,5.32907051820105E-14)) ;
#40615=DIRECTION('center_axis',(4.54195640846217E-14,-1.66321791214601E-16,
1.)) ;
#40616=DIRECTION('ref_axis',(-1.,5.55236256206829E-46,4.54195640846217E-14)) ;
#40617=DIRECTION('center_axis',(2.17161023787787E-15,-3.83815143260382E-28,
-1.)) ;
#40618=DIRECTION('ref_axis',(0.707106781186452,0.707106781186643,1.53556032529709E-15)) ;
#40619=DIRECTION('center_axis',(-8.32667268460786E-17,-1.,-1.66321791214597E-16)) ;
#40620=DIRECTION('ref_axis',(-0.707106781186535,-5.87287992268677E-17,0.70710678118656)) ;
#40621=DIRECTION('center_axis',(0.,1.,0.)) ;
#40622=DIRECTION('ref_axis',(-1.,0.,0.)) ;
#40623=DIRECTION('',(-8.32667268460786E-17,-1.,-1.66321791214597E-16)) ;
#40624=DIRECTION('',(-8.32667268460786E-17,-1.,-1.66321791214597E-16)) ;
#40625=DIRECTION('center_axis',(-4.54195640846217E-14,1.66321791214601E-16,
-1.)) ;
#40626=DIRECTION('ref_axis',(-1.,0.,4.54747350886464E-14)) ;
#40627=DIRECTION('center_axis',(1.,2.84217094304056E-13,0.)) ;
#40628=DIRECTION('ref_axis',(-2.84217094304056E-13,1.,0.)) ;
#40629=DIRECTION('center_axis',(4.54195640846217E-14,-1.66321791214601E-16,
1.)) ;
#40630=DIRECTION('ref_axis',(-1.,5.55236256206829E-46,4.54195640846217E-14)) ;
#40631=DIRECTION('center_axis',(-2.17161023787787E-15,3.83420712807771E-28,
1.)) ;
#40632=DIRECTION('ref_axis',(0.707106781186543,-0.707106781186552,1.53556032529783E-15)) ;
#40633=DIRECTION('center_axis',(-1.,1.66533453692587E-16,4.54195640846217E-14)) ;
#40634=DIRECTION('ref_axis',(3.22342386971791E-14,0.707106781186422,0.707106781186673)) ;
#40635=DIRECTION('center_axis',(1.,0.,0.)) ;
#40636=DIRECTION('ref_axis',(0.,1.,0.)) ;
#40637=DIRECTION('',(-1.,1.66533453692587E-16,4.54195640846217E-14)) ;
#40638=DIRECTION('',(-1.,1.66533453692587E-16,4.54195640846217E-14)) ;
#40639=DIRECTION('center_axis',(-4.54195640846217E-14,1.66321791214601E-16,
-1.)) ;
#40640=DIRECTION('ref_axis',(-1.,0.,4.54747350886464E-14)) ;
#40641=DIRECTION('center_axis',(0.,-1.,0.)) ;
#40642=DIRECTION('ref_axis',(1.,0.,-5.32907051820105E-14)) ;
#40643=DIRECTION('center_axis',(4.54195640846217E-14,-1.66321791214601E-16,
1.)) ;
#40644=DIRECTION('ref_axis',(-1.,5.55236256206829E-46,4.54195640846217E-14)) ;
#40645=DIRECTION('center_axis',(2.1716102378779E-15,-3.83420712807775E-28,
-1.)) ;
#40646=DIRECTION('ref_axis',(-0.707106781186452,-0.707106781186643,-1.53556032529712E-15)) ;
#40647=DIRECTION('center_axis',(1.66533453692965E-16,1.,1.66321791214593E-16)) ;
#40648=DIRECTION('ref_axis',(0.707106781186535,-2.35364200827643E-16,0.70710678118656)) ;
#40649=DIRECTION('center_axis',(0.,-1.,0.)) ;
#40650=DIRECTION('ref_axis',(1.,0.,0.)) ;
#40651=DIRECTION('',(1.66533453692965E-16,1.,1.66321791214593E-16)) ;
#40652=DIRECTION('',(1.66533453692965E-16,1.,1.66321791214593E-16)) ;
#40653=DIRECTION('center_axis',(-4.54195640846217E-14,1.66321791214601E-16,
-1.)) ;
#40654=DIRECTION('ref_axis',(-1.,0.,4.54747350886464E-14)) ;
#40655=DIRECTION('center_axis',(4.54195640846217E-14,-1.66321791214601E-16,
1.)) ;
#40656=DIRECTION('ref_axis',(-1.,5.55236256206829E-46,4.54195640846217E-14)) ;
#40657=DIRECTION('center_axis',(-2.1716102378779E-15,3.83815143260386E-28,
1.)) ;
#40658=DIRECTION('ref_axis',(-0.707106781186643,0.707106781186452,-1.53556032529807E-15)) ;
#40659=DIRECTION('center_axis',(-2.17161023787787E-15,3.83420712807771E-28,
1.)) ;
#40660=DIRECTION('ref_axis',(0.707106781186543,-0.707106781186552,1.53556032529783E-15)) ;
#40661=DIRECTION('',(-2.17161023787787E-15,3.83420712807771E-28,1.)) ;
#40662=DIRECTION('center_axis',(2.17161023787792E-15,-2.90739654573749E-15,
-1.)) ;
#40663=DIRECTION('ref_axis',(1.35627620245787E-13,-1.,2.90739654573778E-15)) ;
#40664=DIRECTION('',(2.17161023787787E-15,-3.83420712807771E-28,-1.)) ;
#40665=DIRECTION('center_axis',(1.,-8.32667268460789E-17,2.17161023787787E-15)) ;
#40666=DIRECTION('ref_axis',(-8.32667268460789E-17,-1.,3.92101138914083E-28)) ;
#40667=DIRECTION('',(2.17161023787787E-15,-3.83815143260382E-28,-1.)) ;
#40668=DIRECTION('',(-8.32667268460789E-17,-1.,3.83780830390118E-28)) ;
#40669=DIRECTION('center_axis',(2.17161023787787E-15,-3.83815143260382E-28,
-1.)) ;
#40670=DIRECTION('ref_axis',(0.707106781186452,0.707106781186643,1.53556032529709E-15)) ;
#40671=DIRECTION('',(-2.17161023787787E-15,3.83815143260382E-28,1.)) ;
#40672=DIRECTION('center_axis',(2.17161023787746E-15,-7.39616701217516E-14,
-1.)) ;
#40673=DIRECTION('ref_axis',(1.,-6.48092690624108E-15,2.17161023787794E-15)) ;
#40674=DIRECTION('center_axis',(1.66533453692966E-16,1.,-3.83386399937507E-28)) ;
#40675=DIRECTION('ref_axis',(2.1716102378779E-15,-3.83748045690496E-28,
-1.)) ;
#40676=DIRECTION('',(2.1716102378779E-15,-3.83815143260386E-28,-1.)) ;
#40677=DIRECTION('',(1.,-1.66533453692966E-16,2.1716102378779E-15)) ;
#40678=DIRECTION('center_axis',(1.,-1.66533453692966E-16,-4.54195640846217E-14)) ;
#40679=DIRECTION('ref_axis',(3.19987248283774E-14,-0.707106781186434,0.707106781186661)) ;
#40680=DIRECTION('center_axis',(1.,0.,0.)) ;
#40681=DIRECTION('ref_axis',(0.,0.,1.)) ;
#40682=DIRECTION('',(1.,-1.66533453692966E-16,-4.54195640846217E-14)) ;
#40683=DIRECTION('center_axis',(-1.,0.,0.)) ;
#40684=DIRECTION('ref_axis',(0.,-1.,0.)) ;
#40685=DIRECTION('',(1.,-1.66533453692966E-16,-4.54195640846217E-14)) ;
#40686=DIRECTION('center_axis',(-4.54195640846217E-14,1.66321791214601E-16,
-1.)) ;
#40687=DIRECTION('ref_axis',(-1.,0.,4.54747350886464E-14)) ;
#40688=DIRECTION('center_axis',(0.,1.,0.)) ;
#40689=DIRECTION('ref_axis',(-1.,0.,5.32907051820105E-14)) ;
#40690=DIRECTION('center_axis',(4.54195640846217E-14,-1.66321791214601E-16,
1.)) ;
#40691=DIRECTION('ref_axis',(-1.,5.55236256206829E-46,4.54195640846217E-14)) ;
#40692=DIRECTION('center_axis',(2.17161023787787E-15,-3.83815143260382E-28,
-1.)) ;
#40693=DIRECTION('ref_axis',(0.707106781186452,0.707106781186643,1.53556032529709E-15)) ;
#40694=DIRECTION('center_axis',(-8.32667268460786E-17,-1.,-1.66321791214597E-16)) ;
#40695=DIRECTION('ref_axis',(-0.707106781186535,-5.87287992268677E-17,0.70710678118656)) ;
#40696=DIRECTION('center_axis',(0.,1.,0.)) ;
#40697=DIRECTION('ref_axis',(-1.,0.,0.)) ;
#40698=DIRECTION('',(-8.32667268460786E-17,-1.,-1.66321791214597E-16)) ;
#40699=DIRECTION('',(-8.32667268460786E-17,-1.,-1.66321791214597E-16)) ;
#40700=DIRECTION('center_axis',(-4.54195640846217E-14,1.66321791214601E-16,
-1.)) ;
#40701=DIRECTION('ref_axis',(-1.,0.,4.54747350886464E-14)) ;
#40702=DIRECTION('center_axis',(1.,2.84217094304056E-13,0.)) ;
#40703=DIRECTION('ref_axis',(-2.84217094304056E-13,1.,0.)) ;
#40704=DIRECTION('center_axis',(4.54195640846217E-14,-1.66321791214601E-16,
1.)) ;
#40705=DIRECTION('ref_axis',(-1.,5.55236256206829E-46,4.54195640846217E-14)) ;
#40706=DIRECTION('center_axis',(-2.17161023787787E-15,3.83420712807771E-28,
1.)) ;
#40707=DIRECTION('ref_axis',(0.707106781186543,-0.707106781186552,1.53556032529783E-15)) ;
#40708=DIRECTION('center_axis',(-1.,1.66533453692587E-16,4.54195640846217E-14)) ;
#40709=DIRECTION('ref_axis',(3.22342386971791E-14,0.707106781186422,0.707106781186673)) ;
#40710=DIRECTION('center_axis',(1.,0.,0.)) ;
#40711=DIRECTION('ref_axis',(0.,1.,0.)) ;
#40712=DIRECTION('',(-1.,1.66533453692587E-16,4.54195640846217E-14)) ;
#40713=DIRECTION('',(-1.,1.66533453692587E-16,4.54195640846217E-14)) ;
#40714=DIRECTION('center_axis',(-4.54195640846217E-14,1.66321791214601E-16,
-1.)) ;
#40715=DIRECTION('ref_axis',(-1.,0.,4.54747350886464E-14)) ;
#40716=DIRECTION('center_axis',(0.,-1.,0.)) ;
#40717=DIRECTION('ref_axis',(1.,0.,-5.32907051820105E-14)) ;
#40718=DIRECTION('center_axis',(4.54195640846217E-14,-1.66321791214601E-16,
1.)) ;
#40719=DIRECTION('ref_axis',(-1.,5.55236256206829E-46,4.54195640846217E-14)) ;
#40720=DIRECTION('center_axis',(2.1716102378779E-15,-3.83420712807775E-28,
-1.)) ;
#40721=DIRECTION('ref_axis',(-0.707106781186452,-0.707106781186643,-1.53556032529712E-15)) ;
#40722=DIRECTION('center_axis',(1.66533453692965E-16,1.,1.66321791214593E-16)) ;
#40723=DIRECTION('ref_axis',(0.707106781186535,-2.35364200827643E-16,0.70710678118656)) ;
#40724=DIRECTION('center_axis',(0.,-1.,0.)) ;
#40725=DIRECTION('ref_axis',(1.,0.,0.)) ;
#40726=DIRECTION('',(1.66533453692965E-16,1.,1.66321791214593E-16)) ;
#40727=DIRECTION('',(1.66533453692965E-16,1.,1.66321791214593E-16)) ;
#40728=DIRECTION('center_axis',(-4.54195640846217E-14,1.66321791214601E-16,
-1.)) ;
#40729=DIRECTION('ref_axis',(-1.,0.,4.54747350886464E-14)) ;
#40730=DIRECTION('center_axis',(4.54195640846217E-14,-1.66321791214601E-16,
1.)) ;
#40731=DIRECTION('ref_axis',(-1.,5.55236256206829E-46,4.54195640846217E-14)) ;
#40732=DIRECTION('center_axis',(-2.1716102378779E-15,3.83815143260386E-28,
1.)) ;
#40733=DIRECTION('ref_axis',(-0.707106781186643,0.707106781186452,-1.53556032529807E-15)) ;
#40734=DIRECTION('center_axis',(-2.17161023787787E-15,3.83420712807771E-28,
1.)) ;
#40735=DIRECTION('ref_axis',(0.707106781186543,-0.707106781186552,1.53556032529783E-15)) ;
#40736=DIRECTION('',(-2.17161023787787E-15,3.83420712807771E-28,1.)) ;
#40737=DIRECTION('center_axis',(2.17161023787792E-15,-2.90739654573749E-15,
-1.)) ;
#40738=DIRECTION('ref_axis',(1.35627620245787E-13,-1.,2.90739654573778E-15)) ;
#40739=DIRECTION('',(2.17161023787787E-15,-3.83420712807771E-28,-1.)) ;
#40740=DIRECTION('center_axis',(1.,-8.32667268460789E-17,2.17161023787787E-15)) ;
#40741=DIRECTION('ref_axis',(-8.32667268460789E-17,-1.,3.92101138914083E-28)) ;
#40742=DIRECTION('',(2.17161023787787E-15,-3.83815143260382E-28,-1.)) ;
#40743=DIRECTION('',(-8.32667268460789E-17,-1.,3.83780830390118E-28)) ;
#40744=DIRECTION('center_axis',(2.17161023787787E-15,-3.83815143260382E-28,
-1.)) ;
#40745=DIRECTION('ref_axis',(0.707106781186452,0.707106781186643,1.53556032529709E-15)) ;
#40746=DIRECTION('',(-2.17161023787787E-15,3.83815143260382E-28,1.)) ;
#40747=DIRECTION('center_axis',(2.17161023787746E-15,-7.39616701217516E-14,
-1.)) ;
#40748=DIRECTION('ref_axis',(1.,-6.48092690624108E-15,2.17161023787794E-15)) ;
#40749=DIRECTION('center_axis',(1.66533453692966E-16,1.,-3.83386399937507E-28)) ;
#40750=DIRECTION('ref_axis',(2.1716102378779E-15,-3.83748045690496E-28,
-1.)) ;
#40751=DIRECTION('',(2.1716102378779E-15,-3.83815143260386E-28,-1.)) ;
#40752=DIRECTION('',(1.,-1.66533453692966E-16,2.1716102378779E-15)) ;
#40753=DIRECTION('center_axis',(1.,-1.66533453692966E-16,-4.54195640846217E-14)) ;
#40754=DIRECTION('ref_axis',(3.19987248283774E-14,-0.707106781186434,0.707106781186661)) ;
#40755=DIRECTION('center_axis',(1.,0.,0.)) ;
#40756=DIRECTION('ref_axis',(0.,0.,1.)) ;
#40757=DIRECTION('',(1.,-1.66533453692966E-16,-4.54195640846217E-14)) ;
#40758=DIRECTION('center_axis',(-1.,0.,0.)) ;
#40759=DIRECTION('ref_axis',(0.,-1.,0.)) ;
#40760=DIRECTION('',(1.,-1.66533453692966E-16,-4.54195640846217E-14)) ;
#40761=DIRECTION('center_axis',(-4.54195640846217E-14,1.66321791214601E-16,
-1.)) ;
#40762=DIRECTION('ref_axis',(-1.,0.,4.54747350886464E-14)) ;
#40763=DIRECTION('center_axis',(0.,1.,0.)) ;
#40764=DIRECTION('ref_axis',(-1.,0.,5.32907051820105E-14)) ;
#40765=DIRECTION('center_axis',(4.54195640846217E-14,-1.66321791214601E-16,
1.)) ;
#40766=DIRECTION('ref_axis',(-1.,5.55236256206829E-46,4.54195640846217E-14)) ;
#40767=DIRECTION('center_axis',(2.17161023787787E-15,-3.83815143260382E-28,
-1.)) ;
#40768=DIRECTION('ref_axis',(0.707106781186452,0.707106781186643,1.53556032529709E-15)) ;
#40769=DIRECTION('center_axis',(-8.32667268460786E-17,-1.,-1.66321791214597E-16)) ;
#40770=DIRECTION('ref_axis',(-0.707106781186535,-5.87287992268677E-17,0.70710678118656)) ;
#40771=DIRECTION('center_axis',(0.,1.,0.)) ;
#40772=DIRECTION('ref_axis',(-1.,0.,0.)) ;
#40773=DIRECTION('',(-8.32667268460786E-17,-1.,-1.66321791214597E-16)) ;
#40774=DIRECTION('',(-8.32667268460786E-17,-1.,-1.66321791214597E-16)) ;
#40775=DIRECTION('center_axis',(-4.54195640846217E-14,1.66321791214601E-16,
-1.)) ;
#40776=DIRECTION('ref_axis',(-1.,0.,4.54747350886464E-14)) ;
#40777=DIRECTION('center_axis',(1.,2.84217094304056E-13,0.)) ;
#40778=DIRECTION('ref_axis',(-2.84217094304056E-13,1.,0.)) ;
#40779=DIRECTION('center_axis',(4.54195640846217E-14,-1.66321791214601E-16,
1.)) ;
#40780=DIRECTION('ref_axis',(-1.,5.55236256206829E-46,4.54195640846217E-14)) ;
#40781=DIRECTION('center_axis',(-2.17161023787787E-15,3.83420712807771E-28,
1.)) ;
#40782=DIRECTION('ref_axis',(0.707106781186543,-0.707106781186552,1.53556032529783E-15)) ;
#40783=DIRECTION('center_axis',(-1.,1.66533453692587E-16,4.54195640846217E-14)) ;
#40784=DIRECTION('ref_axis',(3.22342386971791E-14,0.707106781186422,0.707106781186673)) ;
#40785=DIRECTION('center_axis',(1.,0.,0.)) ;
#40786=DIRECTION('ref_axis',(0.,1.,0.)) ;
#40787=DIRECTION('',(-1.,1.66533453692587E-16,4.54195640846217E-14)) ;
#40788=DIRECTION('',(-1.,1.66533453692587E-16,4.54195640846217E-14)) ;
#40789=DIRECTION('center_axis',(-4.54195640846217E-14,1.66321791214601E-16,
-1.)) ;
#40790=DIRECTION('ref_axis',(-1.,0.,4.54747350886464E-14)) ;
#40791=DIRECTION('center_axis',(0.,-1.,0.)) ;
#40792=DIRECTION('ref_axis',(1.,0.,-5.32907051820105E-14)) ;
#40793=DIRECTION('center_axis',(4.54195640846217E-14,-1.66321791214601E-16,
1.)) ;
#40794=DIRECTION('ref_axis',(-1.,5.55236256206829E-46,4.54195640846217E-14)) ;
#40795=DIRECTION('center_axis',(2.1716102378779E-15,-3.83420712807775E-28,
-1.)) ;
#40796=DIRECTION('ref_axis',(-0.707106781186452,-0.707106781186643,-1.53556032529712E-15)) ;
#40797=DIRECTION('center_axis',(1.66533453692965E-16,1.,1.66321791214593E-16)) ;
#40798=DIRECTION('ref_axis',(0.707106781186535,-2.35364200827643E-16,0.70710678118656)) ;
#40799=DIRECTION('center_axis',(0.,-1.,0.)) ;
#40800=DIRECTION('ref_axis',(1.,0.,0.)) ;
#40801=DIRECTION('',(1.66533453692965E-16,1.,1.66321791214593E-16)) ;
#40802=DIRECTION('',(1.66533453692965E-16,1.,1.66321791214593E-16)) ;
#40803=DIRECTION('center_axis',(-4.54195640846217E-14,1.66321791214601E-16,
-1.)) ;
#40804=DIRECTION('ref_axis',(-1.,0.,4.54747350886464E-14)) ;
#40805=DIRECTION('center_axis',(4.54195640846217E-14,-1.66321791214601E-16,
1.)) ;
#40806=DIRECTION('ref_axis',(-1.,5.55236256206829E-46,4.54195640846217E-14)) ;
#40807=DIRECTION('center_axis',(-2.1716102378779E-15,3.83815143260386E-28,
1.)) ;
#40808=DIRECTION('ref_axis',(-0.707106781186643,0.707106781186452,-1.53556032529807E-15)) ;
#40809=DIRECTION('center_axis',(-2.17161023787787E-15,3.83420712807771E-28,
1.)) ;
#40810=DIRECTION('ref_axis',(0.707106781186543,-0.707106781186552,1.53556032529783E-15)) ;
#40811=DIRECTION('',(-2.17161023787787E-15,3.83420712807771E-28,1.)) ;
#40812=DIRECTION('center_axis',(2.17161023787792E-15,-2.90739654573749E-15,
-1.)) ;
#40813=DIRECTION('ref_axis',(1.35627620245787E-13,-1.,2.90739654573778E-15)) ;
#40814=DIRECTION('',(2.17161023787787E-15,-3.83420712807771E-28,-1.)) ;
#40815=DIRECTION('center_axis',(1.,-8.32667268460789E-17,2.17161023787787E-15)) ;
#40816=DIRECTION('ref_axis',(-8.32667268460789E-17,-1.,3.92101138914083E-28)) ;
#40817=DIRECTION('',(2.17161023787787E-15,-3.83815143260382E-28,-1.)) ;
#40818=DIRECTION('',(-8.32667268460789E-17,-1.,3.83780830390118E-28)) ;
#40819=DIRECTION('center_axis',(2.17161023787787E-15,-3.83815143260382E-28,
-1.)) ;
#40820=DIRECTION('ref_axis',(0.707106781186452,0.707106781186643,1.53556032529709E-15)) ;
#40821=DIRECTION('',(-2.17161023787787E-15,3.83815143260382E-28,1.)) ;
#40822=DIRECTION('center_axis',(2.17161023787746E-15,-7.39616701217516E-14,
-1.)) ;
#40823=DIRECTION('ref_axis',(1.,-6.48092690624108E-15,2.17161023787794E-15)) ;
#40824=DIRECTION('center_axis',(1.66533453692966E-16,1.,-3.83386399937507E-28)) ;
#40825=DIRECTION('ref_axis',(2.1716102378779E-15,-3.83748045690496E-28,
-1.)) ;
#40826=DIRECTION('',(2.1716102378779E-15,-3.83815143260386E-28,-1.)) ;
#40827=DIRECTION('',(1.,-1.66533453692966E-16,2.1716102378779E-15)) ;
#40828=DIRECTION('center_axis',(1.,-1.66533453692966E-16,-4.54195640846217E-14)) ;
#40829=DIRECTION('ref_axis',(3.19987248283774E-14,-0.707106781186434,0.707106781186661)) ;
#40830=DIRECTION('center_axis',(1.,0.,0.)) ;
#40831=DIRECTION('ref_axis',(0.,0.,1.)) ;
#40832=DIRECTION('',(1.,-1.66533453692966E-16,-4.54195640846217E-14)) ;
#40833=DIRECTION('center_axis',(-1.,0.,0.)) ;
#40834=DIRECTION('ref_axis',(0.,-1.,0.)) ;
#40835=DIRECTION('',(1.,-1.66533453692966E-16,-4.54195640846217E-14)) ;
#40836=DIRECTION('center_axis',(-4.54195640846217E-14,1.66321791214601E-16,
-1.)) ;
#40837=DIRECTION('ref_axis',(-1.,0.,4.54747350886464E-14)) ;
#40838=DIRECTION('center_axis',(0.,1.,0.)) ;
#40839=DIRECTION('ref_axis',(-1.,0.,5.32907051820105E-14)) ;
#40840=DIRECTION('center_axis',(4.54195640846217E-14,-1.66321791214601E-16,
1.)) ;
#40841=DIRECTION('ref_axis',(-1.,5.55236256206829E-46,4.54195640846217E-14)) ;
#40842=DIRECTION('center_axis',(2.17161023787787E-15,-3.83815143260382E-28,
-1.)) ;
#40843=DIRECTION('ref_axis',(0.707106781186452,0.707106781186643,1.53556032529709E-15)) ;
#40844=DIRECTION('center_axis',(-8.32667268460786E-17,-1.,-1.66321791214597E-16)) ;
#40845=DIRECTION('ref_axis',(-0.707106781186535,-5.87287992268677E-17,0.70710678118656)) ;
#40846=DIRECTION('center_axis',(0.,1.,0.)) ;
#40847=DIRECTION('ref_axis',(-1.,0.,0.)) ;
#40848=DIRECTION('',(-8.32667268460786E-17,-1.,-1.66321791214597E-16)) ;
#40849=DIRECTION('',(-8.32667268460786E-17,-1.,-1.66321791214597E-16)) ;
#40850=DIRECTION('center_axis',(-4.54195640846217E-14,1.66321791214601E-16,
-1.)) ;
#40851=DIRECTION('ref_axis',(-1.,0.,4.54747350886464E-14)) ;
#40852=DIRECTION('center_axis',(1.,2.84217094304056E-13,0.)) ;
#40853=DIRECTION('ref_axis',(-2.84217094304056E-13,1.,0.)) ;
#40854=DIRECTION('center_axis',(4.54195640846217E-14,-1.66321791214601E-16,
1.)) ;
#40855=DIRECTION('ref_axis',(-1.,5.55236256206829E-46,4.54195640846217E-14)) ;
#40856=DIRECTION('center_axis',(-2.17161023787787E-15,3.83420712807771E-28,
1.)) ;
#40857=DIRECTION('ref_axis',(0.707106781186543,-0.707106781186552,1.53556032529783E-15)) ;
#40858=DIRECTION('center_axis',(-1.,1.66533453692587E-16,4.54195640846217E-14)) ;
#40859=DIRECTION('ref_axis',(3.22342386971791E-14,0.707106781186422,0.707106781186673)) ;
#40860=DIRECTION('center_axis',(1.,0.,0.)) ;
#40861=DIRECTION('ref_axis',(0.,1.,0.)) ;
#40862=DIRECTION('',(-1.,1.66533453692587E-16,4.54195640846217E-14)) ;
#40863=DIRECTION('',(-1.,1.66533453692587E-16,4.54195640846217E-14)) ;
#40864=DIRECTION('center_axis',(-4.54195640846217E-14,1.66321791214601E-16,
-1.)) ;
#40865=DIRECTION('ref_axis',(-1.,0.,4.54747350886464E-14)) ;
#40866=DIRECTION('center_axis',(0.,-1.,0.)) ;
#40867=DIRECTION('ref_axis',(1.,0.,-5.32907051820105E-14)) ;
#40868=DIRECTION('center_axis',(4.54195640846217E-14,-1.66321791214601E-16,
1.)) ;
#40869=DIRECTION('ref_axis',(-1.,5.55236256206829E-46,4.54195640846217E-14)) ;
#40870=DIRECTION('center_axis',(2.1716102378779E-15,-3.83420712807775E-28,
-1.)) ;
#40871=DIRECTION('ref_axis',(-0.707106781186452,-0.707106781186643,-1.53556032529712E-15)) ;
#40872=DIRECTION('center_axis',(1.66533453692965E-16,1.,1.66321791214593E-16)) ;
#40873=DIRECTION('ref_axis',(0.707106781186535,-2.35364200827643E-16,0.70710678118656)) ;
#40874=DIRECTION('center_axis',(0.,-1.,0.)) ;
#40875=DIRECTION('ref_axis',(1.,0.,0.)) ;
#40876=DIRECTION('',(1.66533453692965E-16,1.,1.66321791214593E-16)) ;
#40877=DIRECTION('',(1.66533453692965E-16,1.,1.66321791214593E-16)) ;
#40878=DIRECTION('center_axis',(-4.54195640846217E-14,1.66321791214601E-16,
-1.)) ;
#40879=DIRECTION('ref_axis',(-1.,0.,4.54747350886464E-14)) ;
#40880=DIRECTION('center_axis',(4.54195640846217E-14,-1.66321791214601E-16,
1.)) ;
#40881=DIRECTION('ref_axis',(-1.,5.55236256206829E-46,4.54195640846217E-14)) ;
#40882=DIRECTION('center_axis',(-2.1716102378779E-15,3.83815143260386E-28,
1.)) ;
#40883=DIRECTION('ref_axis',(-0.707106781186643,0.707106781186452,-1.53556032529807E-15)) ;
#40884=DIRECTION('center_axis',(-2.17161023787787E-15,3.83420712807771E-28,
1.)) ;
#40885=DIRECTION('ref_axis',(0.707106781186543,-0.707106781186552,1.53556032529783E-15)) ;
#40886=DIRECTION('',(-2.17161023787787E-15,3.83420712807771E-28,1.)) ;
#40887=DIRECTION('center_axis',(2.17161023787792E-15,-2.90739654573749E-15,
-1.)) ;
#40888=DIRECTION('ref_axis',(1.35627620245787E-13,-1.,2.90739654573778E-15)) ;
#40889=DIRECTION('',(2.17161023787787E-15,-3.83420712807771E-28,-1.)) ;
#40890=DIRECTION('center_axis',(1.,-8.32667268460789E-17,2.17161023787787E-15)) ;
#40891=DIRECTION('ref_axis',(-8.32667268460789E-17,-1.,3.92101138914083E-28)) ;
#40892=DIRECTION('',(2.17161023787787E-15,-3.83815143260382E-28,-1.)) ;
#40893=DIRECTION('',(-8.32667268460789E-17,-1.,3.83780830390118E-28)) ;
#40894=DIRECTION('center_axis',(2.17161023787787E-15,-3.83815143260382E-28,
-1.)) ;
#40895=DIRECTION('ref_axis',(0.707106781186452,0.707106781186643,1.53556032529709E-15)) ;
#40896=DIRECTION('',(-2.17161023787787E-15,3.83815143260382E-28,1.)) ;
#40897=DIRECTION('center_axis',(2.17161023787746E-15,-7.39616701217516E-14,
-1.)) ;
#40898=DIRECTION('ref_axis',(1.,-6.48092690624108E-15,2.17161023787794E-15)) ;
#40899=DIRECTION('center_axis',(1.66533453692966E-16,1.,-3.83386399937507E-28)) ;
#40900=DIRECTION('ref_axis',(2.1716102378779E-15,-3.83748045690496E-28,
-1.)) ;
#40901=DIRECTION('',(2.1716102378779E-15,-3.83815143260386E-28,-1.)) ;
#40902=DIRECTION('',(1.,-1.66533453692966E-16,2.1716102378779E-15)) ;
#40903=DIRECTION('center_axis',(1.,-1.66533453692966E-16,-4.54195640846217E-14)) ;
#40904=DIRECTION('ref_axis',(3.19987248283774E-14,-0.707106781186434,0.707106781186661)) ;
#40905=DIRECTION('center_axis',(1.,0.,0.)) ;
#40906=DIRECTION('ref_axis',(0.,0.,1.)) ;
#40907=DIRECTION('',(1.,-1.66533453692966E-16,-4.54195640846217E-14)) ;
#40908=DIRECTION('center_axis',(-1.,0.,0.)) ;
#40909=DIRECTION('ref_axis',(0.,-1.,0.)) ;
#40910=DIRECTION('',(1.,-1.66533453692966E-16,-4.54195640846217E-14)) ;
#40911=DIRECTION('center_axis',(-4.54195640846217E-14,1.66321791214601E-16,
-1.)) ;
#40912=DIRECTION('ref_axis',(-1.,0.,4.54747350886464E-14)) ;
#40913=DIRECTION('center_axis',(0.,1.,0.)) ;
#40914=DIRECTION('ref_axis',(-1.,0.,5.32907051820105E-14)) ;
#40915=DIRECTION('center_axis',(4.54195640846217E-14,-1.66321791214601E-16,
1.)) ;
#40916=DIRECTION('ref_axis',(-1.,5.55236256206829E-46,4.54195640846217E-14)) ;
#40917=DIRECTION('center_axis',(2.17161023787787E-15,-3.83815143260382E-28,
-1.)) ;
#40918=DIRECTION('ref_axis',(0.707106781186452,0.707106781186643,1.53556032529709E-15)) ;
#40919=DIRECTION('center_axis',(-8.32667268460786E-17,-1.,-1.66321791214597E-16)) ;
#40920=DIRECTION('ref_axis',(-0.707106781186535,-5.87287992268677E-17,0.70710678118656)) ;
#40921=DIRECTION('center_axis',(0.,1.,0.)) ;
#40922=DIRECTION('ref_axis',(-1.,0.,0.)) ;
#40923=DIRECTION('',(-8.32667268460786E-17,-1.,-1.66321791214597E-16)) ;
#40924=DIRECTION('',(-8.32667268460786E-17,-1.,-1.66321791214597E-16)) ;
#40925=DIRECTION('center_axis',(-4.54195640846217E-14,1.66321791214601E-16,
-1.)) ;
#40926=DIRECTION('ref_axis',(-1.,0.,4.54747350886464E-14)) ;
#40927=DIRECTION('center_axis',(1.,2.84217094304056E-13,0.)) ;
#40928=DIRECTION('ref_axis',(-2.84217094304056E-13,1.,0.)) ;
#40929=DIRECTION('center_axis',(4.54195640846217E-14,-1.66321791214601E-16,
1.)) ;
#40930=DIRECTION('ref_axis',(-1.,5.55236256206829E-46,4.54195640846217E-14)) ;
#40931=DIRECTION('center_axis',(-2.17161023787787E-15,3.83420712807771E-28,
1.)) ;
#40932=DIRECTION('ref_axis',(0.707106781186543,-0.707106781186552,1.53556032529783E-15)) ;
#40933=DIRECTION('center_axis',(-1.,1.66533453692587E-16,4.54195640846217E-14)) ;
#40934=DIRECTION('ref_axis',(3.22342386971791E-14,0.707106781186422,0.707106781186673)) ;
#40935=DIRECTION('center_axis',(1.,0.,0.)) ;
#40936=DIRECTION('ref_axis',(0.,1.,0.)) ;
#40937=DIRECTION('',(-1.,1.66533453692587E-16,4.54195640846217E-14)) ;
#40938=DIRECTION('',(-1.,1.66533453692587E-16,4.54195640846217E-14)) ;
#40939=DIRECTION('center_axis',(-4.54195640846217E-14,1.66321791214601E-16,
-1.)) ;
#40940=DIRECTION('ref_axis',(-1.,0.,4.54747350886464E-14)) ;
#40941=DIRECTION('center_axis',(0.,-1.,0.)) ;
#40942=DIRECTION('ref_axis',(1.,0.,-5.32907051820105E-14)) ;
#40943=DIRECTION('center_axis',(4.54195640846217E-14,-1.66321791214601E-16,
1.)) ;
#40944=DIRECTION('ref_axis',(-1.,5.55236256206829E-46,4.54195640846217E-14)) ;
#40945=DIRECTION('center_axis',(2.1716102378779E-15,-3.83420712807775E-28,
-1.)) ;
#40946=DIRECTION('ref_axis',(-0.707106781186452,-0.707106781186643,-1.53556032529712E-15)) ;
#40947=DIRECTION('center_axis',(1.66533453692965E-16,1.,1.66321791214593E-16)) ;
#40948=DIRECTION('ref_axis',(0.707106781186535,-2.35364200827643E-16,0.70710678118656)) ;
#40949=DIRECTION('center_axis',(0.,-1.,0.)) ;
#40950=DIRECTION('ref_axis',(1.,0.,0.)) ;
#40951=DIRECTION('',(1.66533453692965E-16,1.,1.66321791214593E-16)) ;
#40952=DIRECTION('',(1.66533453692965E-16,1.,1.66321791214593E-16)) ;
#40953=DIRECTION('center_axis',(-4.54195640846217E-14,1.66321791214601E-16,
-1.)) ;
#40954=DIRECTION('ref_axis',(-1.,0.,4.54747350886464E-14)) ;
#40955=DIRECTION('center_axis',(4.54195640846217E-14,-1.66321791214601E-16,
1.)) ;
#40956=DIRECTION('ref_axis',(-1.,5.55236256206829E-46,4.54195640846217E-14)) ;
#40957=DIRECTION('center_axis',(-2.1716102378779E-15,3.83815143260386E-28,
1.)) ;
#40958=DIRECTION('ref_axis',(-0.707106781186643,0.707106781186452,-1.53556032529807E-15)) ;
#40959=DIRECTION('center_axis',(-2.17161023787787E-15,3.83420712807771E-28,
1.)) ;
#40960=DIRECTION('ref_axis',(0.707106781186543,-0.707106781186552,1.53556032529783E-15)) ;
#40961=DIRECTION('',(-2.17161023787787E-15,3.83420712807771E-28,1.)) ;
#40962=DIRECTION('center_axis',(2.17161023787792E-15,-2.90739654573749E-15,
-1.)) ;
#40963=DIRECTION('ref_axis',(1.35627620245787E-13,-1.,2.90739654573778E-15)) ;
#40964=DIRECTION('',(2.17161023787787E-15,-3.83420712807771E-28,-1.)) ;
#40965=DIRECTION('center_axis',(1.,-8.32667268460789E-17,2.17161023787787E-15)) ;
#40966=DIRECTION('ref_axis',(-8.32667268460789E-17,-1.,3.92101138914083E-28)) ;
#40967=DIRECTION('',(2.17161023787787E-15,-3.83815143260382E-28,-1.)) ;
#40968=DIRECTION('',(-8.32667268460789E-17,-1.,3.83780830390118E-28)) ;
#40969=DIRECTION('center_axis',(2.17161023787787E-15,-3.83815143260382E-28,
-1.)) ;
#40970=DIRECTION('ref_axis',(0.707106781186452,0.707106781186643,1.53556032529709E-15)) ;
#40971=DIRECTION('',(-2.17161023787787E-15,3.83815143260382E-28,1.)) ;
#40972=DIRECTION('center_axis',(2.17161023787746E-15,-7.39616701217516E-14,
-1.)) ;
#40973=DIRECTION('ref_axis',(1.,-6.48092690624108E-15,2.17161023787794E-15)) ;
#40974=DIRECTION('center_axis',(1.66533453692966E-16,1.,-3.83386399937507E-28)) ;
#40975=DIRECTION('ref_axis',(2.1716102378779E-15,-3.83748045690496E-28,
-1.)) ;
#40976=DIRECTION('',(2.1716102378779E-15,-3.83815143260386E-28,-1.)) ;
#40977=DIRECTION('',(1.,-1.66533453692966E-16,2.1716102378779E-15)) ;
#40978=DIRECTION('center_axis',(1.,-1.66533453692966E-16,-4.54195640846217E-14)) ;
#40979=DIRECTION('ref_axis',(3.19987248283774E-14,-0.707106781186434,0.707106781186661)) ;
#40980=DIRECTION('center_axis',(1.,0.,0.)) ;
#40981=DIRECTION('ref_axis',(0.,0.,1.)) ;
#40982=DIRECTION('',(1.,-1.66533453692966E-16,-4.54195640846217E-14)) ;
#40983=DIRECTION('center_axis',(-1.,0.,0.)) ;
#40984=DIRECTION('ref_axis',(0.,-1.,0.)) ;
#40985=DIRECTION('',(1.,-1.66533453692966E-16,-4.54195640846217E-14)) ;
#40986=DIRECTION('center_axis',(-4.54195640846217E-14,1.66321791214601E-16,
-1.)) ;
#40987=DIRECTION('ref_axis',(-1.,0.,4.54747350886464E-14)) ;
#40988=DIRECTION('center_axis',(0.,1.,0.)) ;
#40989=DIRECTION('ref_axis',(-1.,0.,5.32907051820105E-14)) ;
#40990=DIRECTION('center_axis',(4.54195640846217E-14,-1.66321791214601E-16,
1.)) ;
#40991=DIRECTION('ref_axis',(-1.,5.55236256206829E-46,4.54195640846217E-14)) ;
#40992=DIRECTION('center_axis',(2.1716102378779E-15,-3.83815143260386E-28,
-1.)) ;
#40993=DIRECTION('ref_axis',(0.707106781186552,0.707106781186543,1.53556032529733E-15)) ;
#40994=DIRECTION('center_axis',(-1.66533453692965E-16,-1.,-1.66321791214593E-16)) ;
#40995=DIRECTION('ref_axis',(-0.707106781186535,1.4966797377543E-19,0.70710678118656)) ;
#40996=DIRECTION('center_axis',(0.,1.,0.)) ;
#40997=DIRECTION('ref_axis',(-1.,0.,0.)) ;
#40998=DIRECTION('',(-1.66533453692965E-16,-1.,-1.66321791214593E-16)) ;
#40999=DIRECTION('',(-1.66533453692965E-16,-1.,-1.66321791214593E-16)) ;
#41000=DIRECTION('center_axis',(-4.54195640846217E-14,1.66321791214601E-16,
-1.)) ;
#41001=DIRECTION('ref_axis',(-1.,0.,4.54747350886464E-14)) ;
#41002=DIRECTION('center_axis',(1.,2.84217094304056E-13,0.)) ;
#41003=DIRECTION('ref_axis',(-2.84217094304056E-13,1.,0.)) ;
#41004=DIRECTION('center_axis',(4.54195640846217E-14,-1.66321791214601E-16,
1.)) ;
#41005=DIRECTION('ref_axis',(-1.,5.55236256206829E-46,4.54195640846217E-14)) ;
#41006=DIRECTION('center_axis',(-2.1716102378779E-15,3.83420712807775E-28,
1.)) ;
#41007=DIRECTION('ref_axis',(0.707106781186643,-0.707106781186452,1.53556032529807E-15)) ;
#41008=DIRECTION('center_axis',(-1.,1.66533453692587E-16,4.54195640846217E-14)) ;
#41009=DIRECTION('ref_axis',(3.22342386971791E-14,0.707106781186422,0.707106781186673)) ;
#41010=DIRECTION('center_axis',(1.,0.,0.)) ;
#41011=DIRECTION('ref_axis',(0.,1.,0.)) ;
#41012=DIRECTION('',(-1.,1.66533453692587E-16,4.54195640846217E-14)) ;
#41013=DIRECTION('',(-1.,1.66533453692587E-16,4.54195640846217E-14)) ;
#41014=DIRECTION('center_axis',(-4.54195640846217E-14,1.66321791214601E-16,
-1.)) ;
#41015=DIRECTION('ref_axis',(-1.,0.,4.54747350886464E-14)) ;
#41016=DIRECTION('center_axis',(0.,-1.,0.)) ;
#41017=DIRECTION('ref_axis',(1.,0.,-5.32907051820105E-14)) ;
#41018=DIRECTION('center_axis',(4.54195640846217E-14,-1.66321791214601E-16,
1.)) ;
#41019=DIRECTION('ref_axis',(-1.,5.55236256206829E-46,4.54195640846217E-14)) ;
#41020=DIRECTION('center_axis',(2.17161023787787E-15,-3.83420712807771E-28,
-1.)) ;
#41021=DIRECTION('ref_axis',(-0.707106781186552,-0.707106781186543,-1.53556032529731E-15)) ;
#41022=DIRECTION('center_axis',(8.32667268460786E-17,1.,1.66321791214597E-16)) ;
#41023=DIRECTION('ref_axis',(0.707106781186522,-1.76485733627007E-16,0.707106781186573)) ;
#41024=DIRECTION('center_axis',(0.,-1.,0.)) ;
#41025=DIRECTION('ref_axis',(1.,0.,1.77635683940035E-14)) ;
#41026=DIRECTION('',(8.32667268460786E-17,1.,1.66321791214597E-16)) ;
#41027=DIRECTION('center_axis',(-4.54195640846217E-14,1.66321791214601E-16,
-1.)) ;
#41028=DIRECTION('ref_axis',(-1.,0.,4.54747350886464E-14)) ;
#41029=DIRECTION('center_axis',(4.54195640846217E-14,-1.66321791214601E-16,
1.)) ;
#41030=DIRECTION('ref_axis',(-1.,5.55236256206829E-46,4.54195640846217E-14)) ;
#41031=DIRECTION('center_axis',(-2.17161023787787E-15,3.83815143260382E-28,
1.)) ;
#41032=DIRECTION('ref_axis',(-0.707106781186643,0.707106781186452,-1.53556032529805E-15)) ;
#41033=DIRECTION('center_axis',(-2.1716102378779E-15,3.83420712807775E-28,
1.)) ;
#41034=DIRECTION('ref_axis',(0.707106781186643,-0.707106781186452,1.53556032529807E-15)) ;
#41035=DIRECTION('',(-2.1716102378779E-15,3.83420712807775E-28,1.)) ;
#41036=DIRECTION('center_axis',(2.1716102378779E-15,-3.83420712807775E-28,
-1.)) ;
#41037=DIRECTION('ref_axis',(0.707106781186656,-0.707106781186439,1.5355603252981E-15)) ;
#41038=DIRECTION('',(-2.1716102378779E-15,3.83322105194623E-28,1.)) ;
#41039=DIRECTION('center_axis',(1.,-1.66533453692966E-16,2.1716102378779E-15)) ;
#41040=DIRECTION('ref_axis',(-1.66533453692966E-16,-1.,3.82783884128008E-28)) ;
#41041=DIRECTION('',(-2.1716102378779E-15,3.66854633798134E-28,1.)) ;
#41042=DIRECTION('center_axis',(1.,-1.66533453692966E-16,2.1716102378779E-15)) ;
#41043=DIRECTION('ref_axis',(-1.41780339089703E-15,0.707106781186483,0.707106781186612)) ;
#41044=DIRECTION('',(-1.66533453692966E-16,-1.,3.83386399937507E-28)) ;
#41045=DIRECTION('',(2.1716102378779E-15,-3.83815143260386E-28,-1.)) ;
#41046=DIRECTION('',(-1.66533453692966E-16,-1.,3.83386399937507E-28)) ;
#41047=DIRECTION('center_axis',(1.,-1.66533453692966E-16,2.1716102378779E-15)) ;
#41048=DIRECTION('ref_axis',(-1.65331725969844E-15,-0.707106781186479,0.707106781186616)) ;
#41049=DIRECTION('',(2.1716102378779E-15,-3.66854633798134E-28,-1.)) ;
#41050=DIRECTION('center_axis',(2.1716102378779E-15,-3.83815143260386E-28,
-1.)) ;
#41051=DIRECTION('ref_axis',(0.707106781186552,0.707106781186543,1.53556032529733E-15)) ;
#41052=DIRECTION('',(-2.1716102378779E-15,3.83815143260386E-28,1.)) ;
#41053=DIRECTION('center_axis',(2.1716102378779E-15,-3.83815143260386E-28,
-1.)) ;
#41054=DIRECTION('ref_axis',(0.707106781186582,0.707106781186513,1.5355603252974E-15)) ;
#41055=DIRECTION('center_axis',(1.66533453692966E-16,1.,-3.83386399937507E-28)) ;
#41056=DIRECTION('ref_axis',(2.1716102378779E-15,-3.83748045690496E-28,
-1.)) ;
#41057=DIRECTION('',(2.17161023787787E-15,-3.83815143260382E-28,-1.)) ;
#41058=DIRECTION('',(1.,-1.66533453692966E-16,2.1716102378779E-15)) ;
#41059=DIRECTION('center_axis',(1.,-1.66533453692966E-16,-4.54195640846217E-14)) ;
#41060=DIRECTION('ref_axis',(3.19987248283774E-14,-0.707106781186434,0.707106781186661)) ;
#41061=DIRECTION('center_axis',(1.,0.,0.)) ;
#41062=DIRECTION('ref_axis',(0.,0.,1.)) ;
#41063=DIRECTION('',(1.,-1.66533453692966E-16,-4.54195640846217E-14)) ;
#41064=DIRECTION('center_axis',(-1.,0.,0.)) ;
#41065=DIRECTION('ref_axis',(0.,-1.,0.)) ;
#41066=DIRECTION('',(1.,-1.66533453692966E-16,-4.54195640846217E-14)) ;
#41067=DIRECTION('center_axis',(-4.54195640846217E-14,1.66321791214601E-16,
-1.)) ;
#41068=DIRECTION('ref_axis',(-1.,0.,4.54747350886464E-14)) ;
#41069=DIRECTION('center_axis',(0.,1.,0.)) ;
#41070=DIRECTION('ref_axis',(-1.,0.,5.32907051820105E-14)) ;
#41071=DIRECTION('center_axis',(4.54195640846217E-14,-1.66321791214601E-16,
1.)) ;
#41072=DIRECTION('ref_axis',(-1.,5.55236256206829E-46,4.54195640846217E-14)) ;
#41073=DIRECTION('center_axis',(2.1716102378779E-15,-3.83815143260386E-28,
-1.)) ;
#41074=DIRECTION('ref_axis',(0.707106781186552,0.707106781186543,1.53556032529733E-15)) ;
#41075=DIRECTION('center_axis',(-1.66533453692965E-16,-1.,-1.66321791214593E-16)) ;
#41076=DIRECTION('ref_axis',(-0.707106781186535,1.4966797377543E-19,0.70710678118656)) ;
#41077=DIRECTION('center_axis',(0.,1.,0.)) ;
#41078=DIRECTION('ref_axis',(-1.,0.,0.)) ;
#41079=DIRECTION('',(-1.66533453692965E-16,-1.,-1.66321791214593E-16)) ;
#41080=DIRECTION('',(-1.66533453692965E-16,-1.,-1.66321791214593E-16)) ;
#41081=DIRECTION('center_axis',(-4.54195640846217E-14,1.66321791214601E-16,
-1.)) ;
#41082=DIRECTION('ref_axis',(-1.,0.,4.54747350886464E-14)) ;
#41083=DIRECTION('center_axis',(1.,2.84217094304056E-13,0.)) ;
#41084=DIRECTION('ref_axis',(-2.84217094304056E-13,1.,0.)) ;
#41085=DIRECTION('center_axis',(4.54195640846217E-14,-1.66321791214601E-16,
1.)) ;
#41086=DIRECTION('ref_axis',(-1.,5.55236256206829E-46,4.54195640846217E-14)) ;
#41087=DIRECTION('center_axis',(-2.1716102378779E-15,3.83420712807775E-28,
1.)) ;
#41088=DIRECTION('ref_axis',(0.707106781186643,-0.707106781186452,1.53556032529807E-15)) ;
#41089=DIRECTION('center_axis',(-1.,1.66533453692587E-16,4.54195640846217E-14)) ;
#41090=DIRECTION('ref_axis',(3.22342386971791E-14,0.707106781186422,0.707106781186673)) ;
#41091=DIRECTION('center_axis',(1.,0.,0.)) ;
#41092=DIRECTION('ref_axis',(0.,1.,0.)) ;
#41093=DIRECTION('',(-1.,1.66533453692587E-16,4.54195640846217E-14)) ;
#41094=DIRECTION('',(-1.,1.66533453692587E-16,4.54195640846217E-14)) ;
#41095=DIRECTION('center_axis',(-4.54195640846217E-14,1.66321791214601E-16,
-1.)) ;
#41096=DIRECTION('ref_axis',(-1.,0.,4.54747350886464E-14)) ;
#41097=DIRECTION('center_axis',(0.,-1.,0.)) ;
#41098=DIRECTION('ref_axis',(1.,0.,-5.32907051820105E-14)) ;
#41099=DIRECTION('center_axis',(4.54195640846217E-14,-1.66321791214601E-16,
1.)) ;
#41100=DIRECTION('ref_axis',(-1.,5.55236256206829E-46,4.54195640846217E-14)) ;
#41101=DIRECTION('center_axis',(2.17161023787787E-15,-3.83420712807771E-28,
-1.)) ;
#41102=DIRECTION('ref_axis',(-0.707106781186552,-0.707106781186543,-1.53556032529731E-15)) ;
#41103=DIRECTION('center_axis',(8.32667268460786E-17,1.,1.66321791214597E-16)) ;
#41104=DIRECTION('ref_axis',(0.707106781186522,-1.76485733627007E-16,0.707106781186573)) ;
#41105=DIRECTION('center_axis',(0.,-1.,0.)) ;
#41106=DIRECTION('ref_axis',(1.,0.,1.77635683940035E-14)) ;
#41107=DIRECTION('',(8.32667268460786E-17,1.,1.66321791214597E-16)) ;
#41108=DIRECTION('center_axis',(-4.54195640846217E-14,1.66321791214601E-16,
-1.)) ;
#41109=DIRECTION('ref_axis',(-1.,0.,4.54747350886464E-14)) ;
#41110=DIRECTION('center_axis',(4.54195640846217E-14,-1.66321791214601E-16,
1.)) ;
#41111=DIRECTION('ref_axis',(-1.,5.55236256206829E-46,4.54195640846217E-14)) ;
#41112=DIRECTION('center_axis',(-2.17161023787787E-15,3.83815143260382E-28,
1.)) ;
#41113=DIRECTION('ref_axis',(-0.707106781186643,0.707106781186452,-1.53556032529805E-15)) ;
#41114=DIRECTION('center_axis',(-2.1716102378779E-15,3.83420712807775E-28,
1.)) ;
#41115=DIRECTION('ref_axis',(0.707106781186643,-0.707106781186452,1.53556032529807E-15)) ;
#41116=DIRECTION('',(-2.1716102378779E-15,3.83420712807775E-28,1.)) ;
#41117=DIRECTION('center_axis',(2.1716102378779E-15,-3.83420712807775E-28,
-1.)) ;
#41118=DIRECTION('ref_axis',(0.707106781186656,-0.707106781186439,1.5355603252981E-15)) ;
#41119=DIRECTION('',(-2.1716102378779E-15,3.83322105194623E-28,1.)) ;
#41120=DIRECTION('center_axis',(1.,-1.66533453692966E-16,2.1716102378779E-15)) ;
#41121=DIRECTION('ref_axis',(-1.66533453692966E-16,-1.,3.82783884128008E-28)) ;
#41122=DIRECTION('',(-2.1716102378779E-15,3.66854633798134E-28,1.)) ;
#41123=DIRECTION('center_axis',(1.,-1.66533453692966E-16,2.1716102378779E-15)) ;
#41124=DIRECTION('ref_axis',(-1.41780339089703E-15,0.707106781186483,0.707106781186612)) ;
#41125=DIRECTION('',(-1.66533453692966E-16,-1.,3.83386399937507E-28)) ;
#41126=DIRECTION('',(2.1716102378779E-15,-3.83815143260386E-28,-1.)) ;
#41127=DIRECTION('',(-1.66533453692966E-16,-1.,3.83386399937507E-28)) ;
#41128=DIRECTION('center_axis',(1.,-1.66533453692966E-16,2.1716102378779E-15)) ;
#41129=DIRECTION('ref_axis',(-1.65331725969844E-15,-0.707106781186479,0.707106781186616)) ;
#41130=DIRECTION('',(2.1716102378779E-15,-3.66854633798134E-28,-1.)) ;
#41131=DIRECTION('center_axis',(2.1716102378779E-15,-3.83815143260386E-28,
-1.)) ;
#41132=DIRECTION('ref_axis',(0.707106781186552,0.707106781186543,1.53556032529733E-15)) ;
#41133=DIRECTION('',(-2.1716102378779E-15,3.83815143260386E-28,1.)) ;
#41134=DIRECTION('center_axis',(2.1716102378779E-15,-3.83815143260386E-28,
-1.)) ;
#41135=DIRECTION('ref_axis',(0.707106781186582,0.707106781186513,1.5355603252974E-15)) ;
#41136=DIRECTION('center_axis',(1.66533453692966E-16,1.,-3.83386399937507E-28)) ;
#41137=DIRECTION('ref_axis',(2.1716102378779E-15,-3.83748045690496E-28,
-1.)) ;
#41138=DIRECTION('',(2.17161023787787E-15,-3.83815143260382E-28,-1.)) ;
#41139=DIRECTION('',(1.,-1.66533453692966E-16,2.1716102378779E-15)) ;
#41140=DIRECTION('center_axis',(1.,-1.66533453692966E-16,-4.54195640846217E-14)) ;
#41141=DIRECTION('ref_axis',(3.19987248283774E-14,-0.707106781186434,0.707106781186661)) ;
#41142=DIRECTION('center_axis',(1.,0.,0.)) ;
#41143=DIRECTION('ref_axis',(0.,0.,1.)) ;
#41144=DIRECTION('',(1.,-1.66533453692966E-16,-4.54195640846217E-14)) ;
#41145=DIRECTION('center_axis',(-1.,0.,0.)) ;
#41146=DIRECTION('ref_axis',(0.,-1.,0.)) ;
#41147=DIRECTION('',(1.,-1.66533453692966E-16,-4.54195640846217E-14)) ;
#41148=DIRECTION('center_axis',(-4.54195640846217E-14,1.66321791214601E-16,
-1.)) ;
#41149=DIRECTION('ref_axis',(-1.,0.,4.54747350886464E-14)) ;
#41150=DIRECTION('center_axis',(0.,1.,0.)) ;
#41151=DIRECTION('ref_axis',(-1.,0.,5.32907051820105E-14)) ;
#41152=DIRECTION('center_axis',(4.54195640846217E-14,-1.66321791214601E-16,
1.)) ;
#41153=DIRECTION('ref_axis',(-1.,5.55236256206829E-46,4.54195640846217E-14)) ;
#41154=DIRECTION('center_axis',(2.1716102378779E-15,-3.83815143260386E-28,
-1.)) ;
#41155=DIRECTION('ref_axis',(0.707106781186552,0.707106781186543,1.53556032529733E-15)) ;
#41156=DIRECTION('center_axis',(-1.66533453692965E-16,-1.,-1.66321791214593E-16)) ;
#41157=DIRECTION('ref_axis',(-0.707106781186535,1.4966797377543E-19,0.70710678118656)) ;
#41158=DIRECTION('center_axis',(0.,1.,0.)) ;
#41159=DIRECTION('ref_axis',(-1.,0.,0.)) ;
#41160=DIRECTION('',(-1.66533453692965E-16,-1.,-1.66321791214593E-16)) ;
#41161=DIRECTION('',(-1.66533453692965E-16,-1.,-1.66321791214593E-16)) ;
#41162=DIRECTION('center_axis',(-4.54195640846217E-14,1.66321791214601E-16,
-1.)) ;
#41163=DIRECTION('ref_axis',(-1.,0.,4.54747350886464E-14)) ;
#41164=DIRECTION('center_axis',(1.,2.84217094304056E-13,0.)) ;
#41165=DIRECTION('ref_axis',(-2.84217094304056E-13,1.,0.)) ;
#41166=DIRECTION('center_axis',(4.54195640846217E-14,-1.66321791214601E-16,
1.)) ;
#41167=DIRECTION('ref_axis',(-1.,5.55236256206829E-46,4.54195640846217E-14)) ;
#41168=DIRECTION('center_axis',(-2.1716102378779E-15,3.83420712807775E-28,
1.)) ;
#41169=DIRECTION('ref_axis',(0.707106781186643,-0.707106781186452,1.53556032529807E-15)) ;
#41170=DIRECTION('center_axis',(-1.,1.66533453692587E-16,4.54195640846217E-14)) ;
#41171=DIRECTION('ref_axis',(3.22342386971791E-14,0.707106781186422,0.707106781186673)) ;
#41172=DIRECTION('center_axis',(1.,0.,0.)) ;
#41173=DIRECTION('ref_axis',(0.,1.,0.)) ;
#41174=DIRECTION('',(-1.,1.66533453692587E-16,4.54195640846217E-14)) ;
#41175=DIRECTION('',(-1.,1.66533453692587E-16,4.54195640846217E-14)) ;
#41176=DIRECTION('center_axis',(-4.54195640846217E-14,1.66321791214601E-16,
-1.)) ;
#41177=DIRECTION('ref_axis',(-1.,0.,4.54747350886464E-14)) ;
#41178=DIRECTION('center_axis',(0.,-1.,0.)) ;
#41179=DIRECTION('ref_axis',(1.,0.,-5.32907051820105E-14)) ;
#41180=DIRECTION('center_axis',(4.54195640846217E-14,-1.66321791214601E-16,
1.)) ;
#41181=DIRECTION('ref_axis',(-1.,5.55236256206829E-46,4.54195640846217E-14)) ;
#41182=DIRECTION('center_axis',(2.17161023787787E-15,-3.83420712807771E-28,
-1.)) ;
#41183=DIRECTION('ref_axis',(-0.707106781186552,-0.707106781186543,-1.53556032529731E-15)) ;
#41184=DIRECTION('center_axis',(8.32667268460786E-17,1.,1.66321791214597E-16)) ;
#41185=DIRECTION('ref_axis',(0.707106781186522,-1.76485733627007E-16,0.707106781186573)) ;
#41186=DIRECTION('center_axis',(0.,-1.,0.)) ;
#41187=DIRECTION('ref_axis',(1.,0.,1.77635683940035E-14)) ;
#41188=DIRECTION('',(8.32667268460786E-17,1.,1.66321791214597E-16)) ;
#41189=DIRECTION('center_axis',(-4.54195640846217E-14,1.66321791214601E-16,
-1.)) ;
#41190=DIRECTION('ref_axis',(-1.,0.,4.54747350886464E-14)) ;
#41191=DIRECTION('center_axis',(4.54195640846217E-14,-1.66321791214601E-16,
1.)) ;
#41192=DIRECTION('ref_axis',(-1.,5.55236256206829E-46,4.54195640846217E-14)) ;
#41193=DIRECTION('center_axis',(-2.17161023787787E-15,3.83815143260382E-28,
1.)) ;
#41194=DIRECTION('ref_axis',(-0.707106781186643,0.707106781186452,-1.53556032529805E-15)) ;
#41195=DIRECTION('center_axis',(-2.1716102378779E-15,3.83420712807775E-28,
1.)) ;
#41196=DIRECTION('ref_axis',(0.707106781186643,-0.707106781186452,1.53556032529807E-15)) ;
#41197=DIRECTION('',(-2.1716102378779E-15,3.83420712807775E-28,1.)) ;
#41198=DIRECTION('center_axis',(2.1716102378779E-15,-3.83420712807775E-28,
-1.)) ;
#41199=DIRECTION('ref_axis',(0.707106781186656,-0.707106781186439,1.5355603252981E-15)) ;
#41200=DIRECTION('',(-2.1716102378779E-15,3.83322105194623E-28,1.)) ;
#41201=DIRECTION('center_axis',(1.,-1.66533453692966E-16,2.1716102378779E-15)) ;
#41202=DIRECTION('ref_axis',(-1.66533453692966E-16,-1.,3.82783884128008E-28)) ;
#41203=DIRECTION('',(-2.1716102378779E-15,3.66854633798134E-28,1.)) ;
#41204=DIRECTION('center_axis',(1.,-1.66533453692966E-16,2.1716102378779E-15)) ;
#41205=DIRECTION('ref_axis',(-1.41780339089703E-15,0.707106781186483,0.707106781186612)) ;
#41206=DIRECTION('',(-1.66533453692966E-16,-1.,3.83386399937507E-28)) ;
#41207=DIRECTION('',(2.1716102378779E-15,-3.83815143260386E-28,-1.)) ;
#41208=DIRECTION('',(-1.66533453692966E-16,-1.,3.83386399937507E-28)) ;
#41209=DIRECTION('center_axis',(1.,-1.66533453692966E-16,2.1716102378779E-15)) ;
#41210=DIRECTION('ref_axis',(-1.65331725969844E-15,-0.707106781186479,0.707106781186616)) ;
#41211=DIRECTION('',(2.1716102378779E-15,-3.66854633798134E-28,-1.)) ;
#41212=DIRECTION('center_axis',(2.1716102378779E-15,-3.83815143260386E-28,
-1.)) ;
#41213=DIRECTION('ref_axis',(0.707106781186552,0.707106781186543,1.53556032529733E-15)) ;
#41214=DIRECTION('',(-2.1716102378779E-15,3.83815143260386E-28,1.)) ;
#41215=DIRECTION('center_axis',(2.1716102378779E-15,-3.83815143260386E-28,
-1.)) ;
#41216=DIRECTION('ref_axis',(0.707106781186582,0.707106781186513,1.5355603252974E-15)) ;
#41217=DIRECTION('center_axis',(1.66533453692966E-16,1.,-3.83386399937507E-28)) ;
#41218=DIRECTION('ref_axis',(2.1716102378779E-15,-3.83748045690496E-28,
-1.)) ;
#41219=DIRECTION('',(2.17161023787787E-15,-3.83815143260382E-28,-1.)) ;
#41220=DIRECTION('',(1.,-1.66533453692966E-16,2.1716102378779E-15)) ;
#41221=DIRECTION('center_axis',(1.,-1.66533453692966E-16,-4.54195640846217E-14)) ;
#41222=DIRECTION('ref_axis',(3.19987248283774E-14,-0.707106781186434,0.707106781186661)) ;
#41223=DIRECTION('center_axis',(1.,0.,0.)) ;
#41224=DIRECTION('ref_axis',(0.,0.,1.)) ;
#41225=DIRECTION('',(1.,-1.66533453692966E-16,-4.54195640846217E-14)) ;
#41226=DIRECTION('center_axis',(-1.,0.,0.)) ;
#41227=DIRECTION('ref_axis',(0.,-1.,0.)) ;
#41228=DIRECTION('',(1.,-1.66533453692966E-16,-4.54195640846217E-14)) ;
#41229=DIRECTION('center_axis',(-4.54195640846217E-14,1.66321791214601E-16,
-1.)) ;
#41230=DIRECTION('ref_axis',(-1.,0.,4.54747350886464E-14)) ;
#41231=DIRECTION('center_axis',(0.,1.,0.)) ;
#41232=DIRECTION('ref_axis',(-1.,0.,5.32907051820105E-14)) ;
#41233=DIRECTION('center_axis',(4.54195640846217E-14,-1.66321791214601E-16,
1.)) ;
#41234=DIRECTION('ref_axis',(-1.,5.55236256206829E-46,4.54195640846217E-14)) ;
#41235=DIRECTION('center_axis',(2.1716102378779E-15,-3.83815143260386E-28,
-1.)) ;
#41236=DIRECTION('ref_axis',(0.707106781186552,0.707106781186543,1.53556032529733E-15)) ;
#41237=DIRECTION('center_axis',(-1.66533453692965E-16,-1.,-1.66321791214593E-16)) ;
#41238=DIRECTION('ref_axis',(-0.707106781186535,1.4966797377543E-19,0.70710678118656)) ;
#41239=DIRECTION('center_axis',(0.,1.,0.)) ;
#41240=DIRECTION('ref_axis',(-1.,0.,0.)) ;
#41241=DIRECTION('',(-1.66533453692965E-16,-1.,-1.66321791214593E-16)) ;
#41242=DIRECTION('',(-1.66533453692965E-16,-1.,-1.66321791214593E-16)) ;
#41243=DIRECTION('center_axis',(-4.54195640846217E-14,1.66321791214601E-16,
-1.)) ;
#41244=DIRECTION('ref_axis',(-1.,0.,4.54747350886464E-14)) ;
#41245=DIRECTION('center_axis',(1.,2.84217094304056E-13,0.)) ;
#41246=DIRECTION('ref_axis',(-2.84217094304056E-13,1.,0.)) ;
#41247=DIRECTION('center_axis',(4.54195640846217E-14,-1.66321791214601E-16,
1.)) ;
#41248=DIRECTION('ref_axis',(-1.,5.55236256206829E-46,4.54195640846217E-14)) ;
#41249=DIRECTION('center_axis',(-2.1716102378779E-15,3.83420712807775E-28,
1.)) ;
#41250=DIRECTION('ref_axis',(0.707106781186643,-0.707106781186452,1.53556032529807E-15)) ;
#41251=DIRECTION('center_axis',(-1.,1.66533453692587E-16,4.54195640846217E-14)) ;
#41252=DIRECTION('ref_axis',(3.22342386971791E-14,0.707106781186422,0.707106781186673)) ;
#41253=DIRECTION('center_axis',(1.,0.,0.)) ;
#41254=DIRECTION('ref_axis',(0.,1.,0.)) ;
#41255=DIRECTION('',(-1.,1.66533453692587E-16,4.54195640846217E-14)) ;
#41256=DIRECTION('',(-1.,1.66533453692587E-16,4.54195640846217E-14)) ;
#41257=DIRECTION('center_axis',(-4.54195640846217E-14,1.66321791214601E-16,
-1.)) ;
#41258=DIRECTION('ref_axis',(-1.,0.,4.54747350886464E-14)) ;
#41259=DIRECTION('center_axis',(0.,-1.,0.)) ;
#41260=DIRECTION('ref_axis',(1.,0.,-5.32907051820105E-14)) ;
#41261=DIRECTION('center_axis',(4.54195640846217E-14,-1.66321791214601E-16,
1.)) ;
#41262=DIRECTION('ref_axis',(-1.,5.55236256206829E-46,4.54195640846217E-14)) ;
#41263=DIRECTION('center_axis',(2.17161023787787E-15,-3.83420712807771E-28,
-1.)) ;
#41264=DIRECTION('ref_axis',(-0.707106781186552,-0.707106781186543,-1.53556032529731E-15)) ;
#41265=DIRECTION('center_axis',(8.32667268460786E-17,1.,1.66321791214597E-16)) ;
#41266=DIRECTION('ref_axis',(0.707106781186522,-1.76485733627007E-16,0.707106781186573)) ;
#41267=DIRECTION('center_axis',(0.,-1.,0.)) ;
#41268=DIRECTION('ref_axis',(1.,0.,1.77635683940035E-14)) ;
#41269=DIRECTION('',(8.32667268460786E-17,1.,1.66321791214597E-16)) ;
#41270=DIRECTION('center_axis',(-4.54195640846217E-14,1.66321791214601E-16,
-1.)) ;
#41271=DIRECTION('ref_axis',(-1.,0.,4.54747350886464E-14)) ;
#41272=DIRECTION('center_axis',(4.54195640846217E-14,-1.66321791214601E-16,
1.)) ;
#41273=DIRECTION('ref_axis',(-1.,5.55236256206829E-46,4.54195640846217E-14)) ;
#41274=DIRECTION('center_axis',(-2.17161023787787E-15,3.83815143260382E-28,
1.)) ;
#41275=DIRECTION('ref_axis',(-0.707106781186643,0.707106781186452,-1.53556032529805E-15)) ;
#41276=DIRECTION('center_axis',(-2.1716102378779E-15,3.83420712807775E-28,
1.)) ;
#41277=DIRECTION('ref_axis',(0.707106781186643,-0.707106781186452,1.53556032529807E-15)) ;
#41278=DIRECTION('',(-2.1716102378779E-15,3.83420712807775E-28,1.)) ;
#41279=DIRECTION('center_axis',(2.1716102378779E-15,-3.83420712807775E-28,
-1.)) ;
#41280=DIRECTION('ref_axis',(0.707106781186656,-0.707106781186439,1.5355603252981E-15)) ;
#41281=DIRECTION('',(-2.1716102378779E-15,3.83322105194623E-28,1.)) ;
#41282=DIRECTION('center_axis',(1.,-1.66533453692966E-16,2.1716102378779E-15)) ;
#41283=DIRECTION('ref_axis',(-1.66533453692966E-16,-1.,3.82783884128008E-28)) ;
#41284=DIRECTION('',(-2.1716102378779E-15,3.66854633798134E-28,1.)) ;
#41285=DIRECTION('center_axis',(1.,-1.66533453692966E-16,2.1716102378779E-15)) ;
#41286=DIRECTION('ref_axis',(-1.41780339089703E-15,0.707106781186483,0.707106781186612)) ;
#41287=DIRECTION('',(-1.66533453692966E-16,-1.,3.83386399937507E-28)) ;
#41288=DIRECTION('',(2.1716102378779E-15,-3.83815143260386E-28,-1.)) ;
#41289=DIRECTION('',(-1.66533453692966E-16,-1.,3.83386399937507E-28)) ;
#41290=DIRECTION('center_axis',(1.,-1.66533453692966E-16,2.1716102378779E-15)) ;
#41291=DIRECTION('ref_axis',(-1.65331725969844E-15,-0.707106781186479,0.707106781186616)) ;
#41292=DIRECTION('',(2.1716102378779E-15,-3.66854633798134E-28,-1.)) ;
#41293=DIRECTION('center_axis',(2.1716102378779E-15,-3.83815143260386E-28,
-1.)) ;
#41294=DIRECTION('ref_axis',(0.707106781186552,0.707106781186543,1.53556032529733E-15)) ;
#41295=DIRECTION('',(-2.1716102378779E-15,3.83815143260386E-28,1.)) ;
#41296=DIRECTION('center_axis',(2.1716102378779E-15,-3.83815143260386E-28,
-1.)) ;
#41297=DIRECTION('ref_axis',(0.707106781186582,0.707106781186513,1.5355603252974E-15)) ;
#41298=DIRECTION('center_axis',(1.66533453692966E-16,1.,-3.83386399937507E-28)) ;
#41299=DIRECTION('ref_axis',(2.1716102378779E-15,-3.83748045690496E-28,
-1.)) ;
#41300=DIRECTION('',(2.17161023787787E-15,-3.83815143260382E-28,-1.)) ;
#41301=DIRECTION('',(1.,-1.66533453692966E-16,2.1716102378779E-15)) ;
#41302=DIRECTION('center_axis',(1.,-1.66533453692966E-16,-4.54195640846217E-14)) ;
#41303=DIRECTION('ref_axis',(3.19987248283774E-14,-0.707106781186434,0.707106781186661)) ;
#41304=DIRECTION('center_axis',(1.,0.,0.)) ;
#41305=DIRECTION('ref_axis',(0.,0.,1.)) ;
#41306=DIRECTION('',(1.,-1.66533453692966E-16,-4.54195640846217E-14)) ;
#41307=DIRECTION('center_axis',(-1.,0.,0.)) ;
#41308=DIRECTION('ref_axis',(0.,-1.,0.)) ;
#41309=DIRECTION('',(1.,-1.66533453692966E-16,-4.54195640846217E-14)) ;
#41310=DIRECTION('center_axis',(-4.54195640846217E-14,1.66321791214601E-16,
-1.)) ;
#41311=DIRECTION('ref_axis',(-1.,0.,4.54747350886464E-14)) ;
#41312=DIRECTION('center_axis',(0.,1.,0.)) ;
#41313=DIRECTION('ref_axis',(-1.,0.,5.32907051820105E-14)) ;
#41314=DIRECTION('center_axis',(4.54195640846217E-14,-1.66321791214601E-16,
1.)) ;
#41315=DIRECTION('ref_axis',(-1.,5.55236256206829E-46,4.54195640846217E-14)) ;
#41316=DIRECTION('center_axis',(2.1716102378779E-15,-3.83815143260386E-28,
-1.)) ;
#41317=DIRECTION('ref_axis',(0.707106781186552,0.707106781186543,1.53556032529733E-15)) ;
#41318=DIRECTION('center_axis',(-1.66533453692965E-16,-1.,-1.66321791214593E-16)) ;
#41319=DIRECTION('ref_axis',(-0.707106781186535,1.4966797377543E-19,0.70710678118656)) ;
#41320=DIRECTION('center_axis',(0.,1.,0.)) ;
#41321=DIRECTION('ref_axis',(-1.,0.,0.)) ;
#41322=DIRECTION('',(-1.66533453692965E-16,-1.,-1.66321791214593E-16)) ;
#41323=DIRECTION('',(-1.66533453692965E-16,-1.,-1.66321791214593E-16)) ;
#41324=DIRECTION('center_axis',(-4.54195640846217E-14,1.66321791214601E-16,
-1.)) ;
#41325=DIRECTION('ref_axis',(-1.,0.,4.54747350886464E-14)) ;
#41326=DIRECTION('center_axis',(1.,2.84217094304056E-13,0.)) ;
#41327=DIRECTION('ref_axis',(-2.84217094304056E-13,1.,0.)) ;
#41328=DIRECTION('center_axis',(4.54195640846217E-14,-1.66321791214601E-16,
1.)) ;
#41329=DIRECTION('ref_axis',(-1.,5.55236256206829E-46,4.54195640846217E-14)) ;
#41330=DIRECTION('center_axis',(-2.1716102378779E-15,3.83420712807775E-28,
1.)) ;
#41331=DIRECTION('ref_axis',(0.707106781186643,-0.707106781186452,1.53556032529807E-15)) ;
#41332=DIRECTION('center_axis',(-1.,1.66533453692587E-16,4.54195640846217E-14)) ;
#41333=DIRECTION('ref_axis',(3.22342386971791E-14,0.707106781186422,0.707106781186673)) ;
#41334=DIRECTION('center_axis',(1.,0.,0.)) ;
#41335=DIRECTION('ref_axis',(0.,1.,0.)) ;
#41336=DIRECTION('',(-1.,1.66533453692587E-16,4.54195640846217E-14)) ;
#41337=DIRECTION('',(-1.,1.66533453692587E-16,4.54195640846217E-14)) ;
#41338=DIRECTION('center_axis',(-4.54195640846217E-14,1.66321791214601E-16,
-1.)) ;
#41339=DIRECTION('ref_axis',(-1.,0.,4.54747350886464E-14)) ;
#41340=DIRECTION('center_axis',(0.,-1.,0.)) ;
#41341=DIRECTION('ref_axis',(1.,0.,-5.32907051820105E-14)) ;
#41342=DIRECTION('center_axis',(4.54195640846217E-14,-1.66321791214601E-16,
1.)) ;
#41343=DIRECTION('ref_axis',(-1.,5.55236256206829E-46,4.54195640846217E-14)) ;
#41344=DIRECTION('center_axis',(2.17161023787787E-15,-3.83420712807771E-28,
-1.)) ;
#41345=DIRECTION('ref_axis',(-0.707106781186552,-0.707106781186543,-1.53556032529731E-15)) ;
#41346=DIRECTION('center_axis',(8.32667268460786E-17,1.,1.66321791214597E-16)) ;
#41347=DIRECTION('ref_axis',(0.707106781186522,-1.76485733627007E-16,0.707106781186573)) ;
#41348=DIRECTION('center_axis',(0.,-1.,0.)) ;
#41349=DIRECTION('ref_axis',(1.,0.,1.77635683940035E-14)) ;
#41350=DIRECTION('',(8.32667268460786E-17,1.,1.66321791214597E-16)) ;
#41351=DIRECTION('center_axis',(-4.54195640846217E-14,1.66321791214601E-16,
-1.)) ;
#41352=DIRECTION('ref_axis',(-1.,0.,4.54747350886464E-14)) ;
#41353=DIRECTION('center_axis',(4.54195640846217E-14,-1.66321791214601E-16,
1.)) ;
#41354=DIRECTION('ref_axis',(-1.,5.55236256206829E-46,4.54195640846217E-14)) ;
#41355=DIRECTION('center_axis',(-2.17161023787787E-15,3.83815143260382E-28,
1.)) ;
#41356=DIRECTION('ref_axis',(-0.707106781186643,0.707106781186452,-1.53556032529805E-15)) ;
#41357=DIRECTION('center_axis',(-2.1716102378779E-15,3.83420712807775E-28,
1.)) ;
#41358=DIRECTION('ref_axis',(0.707106781186643,-0.707106781186452,1.53556032529807E-15)) ;
#41359=DIRECTION('',(-2.1716102378779E-15,3.83420712807775E-28,1.)) ;
#41360=DIRECTION('center_axis',(2.1716102378779E-15,-3.83420712807775E-28,
-1.)) ;
#41361=DIRECTION('ref_axis',(0.707106781186656,-0.707106781186439,1.5355603252981E-15)) ;
#41362=DIRECTION('',(-2.1716102378779E-15,3.83322105194623E-28,1.)) ;
#41363=DIRECTION('center_axis',(1.,-1.66533453692966E-16,2.1716102378779E-15)) ;
#41364=DIRECTION('ref_axis',(-1.66533453692966E-16,-1.,3.82783884128008E-28)) ;
#41365=DIRECTION('',(-2.1716102378779E-15,3.66854633798134E-28,1.)) ;
#41366=DIRECTION('center_axis',(1.,-1.66533453692966E-16,2.1716102378779E-15)) ;
#41367=DIRECTION('ref_axis',(-1.41780339089703E-15,0.707106781186483,0.707106781186612)) ;
#41368=DIRECTION('',(-1.66533453692966E-16,-1.,3.83386399937507E-28)) ;
#41369=DIRECTION('',(2.1716102378779E-15,-3.83815143260386E-28,-1.)) ;
#41370=DIRECTION('',(-1.66533453692966E-16,-1.,3.83386399937507E-28)) ;
#41371=DIRECTION('center_axis',(1.,-1.66533453692966E-16,2.1716102378779E-15)) ;
#41372=DIRECTION('ref_axis',(-1.65331725969844E-15,-0.707106781186479,0.707106781186616)) ;
#41373=DIRECTION('',(2.1716102378779E-15,-3.66854633798134E-28,-1.)) ;
#41374=DIRECTION('center_axis',(2.1716102378779E-15,-3.83815143260386E-28,
-1.)) ;
#41375=DIRECTION('ref_axis',(0.707106781186552,0.707106781186543,1.53556032529733E-15)) ;
#41376=DIRECTION('',(-2.1716102378779E-15,3.83815143260386E-28,1.)) ;
#41377=DIRECTION('center_axis',(2.1716102378779E-15,-3.83815143260386E-28,
-1.)) ;
#41378=DIRECTION('ref_axis',(0.707106781186582,0.707106781186513,1.5355603252974E-15)) ;
#41379=DIRECTION('center_axis',(1.66533453692966E-16,1.,-3.83386399937507E-28)) ;
#41380=DIRECTION('ref_axis',(2.1716102378779E-15,-3.83748045690496E-28,
-1.)) ;
#41381=DIRECTION('',(2.17161023787787E-15,-3.83815143260382E-28,-1.)) ;
#41382=DIRECTION('',(1.,-1.66533453692966E-16,2.1716102378779E-15)) ;
#41383=DIRECTION('center_axis',(1.,-1.66533453692966E-16,-4.54195640846217E-14)) ;
#41384=DIRECTION('ref_axis',(3.19987248283774E-14,-0.707106781186434,0.707106781186661)) ;
#41385=DIRECTION('center_axis',(1.,0.,0.)) ;
#41386=DIRECTION('ref_axis',(0.,0.,1.)) ;
#41387=DIRECTION('',(1.,-1.66533453692966E-16,-4.54195640846217E-14)) ;
#41388=DIRECTION('center_axis',(-1.,0.,0.)) ;
#41389=DIRECTION('ref_axis',(0.,-1.,0.)) ;
#41390=DIRECTION('',(1.,-1.66533453692966E-16,-4.54195640846217E-14)) ;
#41391=DIRECTION('center_axis',(-4.54195640846217E-14,1.66321791214601E-16,
-1.)) ;
#41392=DIRECTION('ref_axis',(-1.,0.,4.54747350886464E-14)) ;
#41393=DIRECTION('center_axis',(0.,1.,0.)) ;
#41394=DIRECTION('ref_axis',(-1.,0.,5.32907051820105E-14)) ;
#41395=DIRECTION('center_axis',(4.54195640846217E-14,-1.66321791214601E-16,
1.)) ;
#41396=DIRECTION('ref_axis',(-1.,5.55236256206829E-46,4.54195640846217E-14)) ;
#41397=DIRECTION('center_axis',(2.1716102378779E-15,-3.83815143260386E-28,
-1.)) ;
#41398=DIRECTION('ref_axis',(0.707106781186552,0.707106781186543,1.53556032529733E-15)) ;
#41399=DIRECTION('center_axis',(-1.66533453692965E-16,-1.,-1.66321791214593E-16)) ;
#41400=DIRECTION('ref_axis',(-0.707106781186535,1.4966797377543E-19,0.70710678118656)) ;
#41401=DIRECTION('center_axis',(0.,1.,0.)) ;
#41402=DIRECTION('ref_axis',(-1.,0.,0.)) ;
#41403=DIRECTION('',(-1.66533453692965E-16,-1.,-1.66321791214593E-16)) ;
#41404=DIRECTION('',(-1.66533453692965E-16,-1.,-1.66321791214593E-16)) ;
#41405=DIRECTION('center_axis',(-4.54195640846217E-14,1.66321791214601E-16,
-1.)) ;
#41406=DIRECTION('ref_axis',(-1.,0.,4.54747350886464E-14)) ;
#41407=DIRECTION('center_axis',(1.,2.84217094304056E-13,0.)) ;
#41408=DIRECTION('ref_axis',(-2.84217094304056E-13,1.,0.)) ;
#41409=DIRECTION('center_axis',(4.54195640846217E-14,-1.66321791214601E-16,
1.)) ;
#41410=DIRECTION('ref_axis',(-1.,5.55236256206829E-46,4.54195640846217E-14)) ;
#41411=DIRECTION('center_axis',(-2.1716102378779E-15,3.83420712807775E-28,
1.)) ;
#41412=DIRECTION('ref_axis',(0.707106781186643,-0.707106781186452,1.53556032529807E-15)) ;
#41413=DIRECTION('center_axis',(-1.,1.66533453692587E-16,4.54195640846217E-14)) ;
#41414=DIRECTION('ref_axis',(3.22342386971791E-14,0.707106781186422,0.707106781186673)) ;
#41415=DIRECTION('center_axis',(1.,0.,0.)) ;
#41416=DIRECTION('ref_axis',(0.,1.,0.)) ;
#41417=DIRECTION('',(-1.,1.66533453692587E-16,4.54195640846217E-14)) ;
#41418=DIRECTION('',(-1.,1.66533453692587E-16,4.54195640846217E-14)) ;
#41419=DIRECTION('center_axis',(-4.54195640846217E-14,1.66321791214601E-16,
-1.)) ;
#41420=DIRECTION('ref_axis',(-1.,0.,4.54747350886464E-14)) ;
#41421=DIRECTION('center_axis',(0.,-1.,0.)) ;
#41422=DIRECTION('ref_axis',(1.,0.,-5.32907051820105E-14)) ;
#41423=DIRECTION('center_axis',(4.54195640846217E-14,-1.66321791214601E-16,
1.)) ;
#41424=DIRECTION('ref_axis',(-1.,5.55236256206829E-46,4.54195640846217E-14)) ;
#41425=DIRECTION('center_axis',(2.17161023787787E-15,-3.83420712807771E-28,
-1.)) ;
#41426=DIRECTION('ref_axis',(-0.707106781186552,-0.707106781186543,-1.53556032529731E-15)) ;
#41427=DIRECTION('center_axis',(8.32667268460786E-17,1.,1.66321791214597E-16)) ;
#41428=DIRECTION('ref_axis',(0.707106781186522,-1.76485733627007E-16,0.707106781186573)) ;
#41429=DIRECTION('center_axis',(0.,-1.,0.)) ;
#41430=DIRECTION('ref_axis',(1.,0.,1.77635683940035E-14)) ;
#41431=DIRECTION('',(8.32667268460786E-17,1.,1.66321791214597E-16)) ;
#41432=DIRECTION('center_axis',(-4.54195640846217E-14,1.66321791214601E-16,
-1.)) ;
#41433=DIRECTION('ref_axis',(-1.,0.,4.54747350886464E-14)) ;
#41434=DIRECTION('center_axis',(4.54195640846217E-14,-1.66321791214601E-16,
1.)) ;
#41435=DIRECTION('ref_axis',(-1.,5.55236256206829E-46,4.54195640846217E-14)) ;
#41436=DIRECTION('center_axis',(-2.17161023787787E-15,3.83815143260382E-28,
1.)) ;
#41437=DIRECTION('ref_axis',(-0.707106781186643,0.707106781186452,-1.53556032529805E-15)) ;
#41438=DIRECTION('center_axis',(-2.1716102378779E-15,3.83420712807775E-28,
1.)) ;
#41439=DIRECTION('ref_axis',(0.707106781186643,-0.707106781186452,1.53556032529807E-15)) ;
#41440=DIRECTION('',(-2.1716102378779E-15,3.83420712807775E-28,1.)) ;
#41441=DIRECTION('center_axis',(2.1716102378779E-15,-3.83420712807775E-28,
-1.)) ;
#41442=DIRECTION('ref_axis',(0.707106781186656,-0.707106781186439,1.5355603252981E-15)) ;
#41443=DIRECTION('',(-2.1716102378779E-15,3.83322105194623E-28,1.)) ;
#41444=DIRECTION('center_axis',(1.,-1.66533453692966E-16,2.1716102378779E-15)) ;
#41445=DIRECTION('ref_axis',(-1.66533453692966E-16,-1.,3.82783884128008E-28)) ;
#41446=DIRECTION('',(-2.1716102378779E-15,3.66854633798134E-28,1.)) ;
#41447=DIRECTION('center_axis',(1.,-1.66533453692966E-16,2.1716102378779E-15)) ;
#41448=DIRECTION('ref_axis',(-1.41780339089703E-15,0.707106781186483,0.707106781186612)) ;
#41449=DIRECTION('',(-1.66533453692966E-16,-1.,3.83386399937507E-28)) ;
#41450=DIRECTION('',(2.1716102378779E-15,-3.83815143260386E-28,-1.)) ;
#41451=DIRECTION('',(-1.66533453692966E-16,-1.,3.83386399937507E-28)) ;
#41452=DIRECTION('center_axis',(1.,-1.66533453692966E-16,2.1716102378779E-15)) ;
#41453=DIRECTION('ref_axis',(-1.65331725969844E-15,-0.707106781186479,0.707106781186616)) ;
#41454=DIRECTION('',(2.1716102378779E-15,-3.66854633798134E-28,-1.)) ;
#41455=DIRECTION('center_axis',(2.1716102378779E-15,-3.83815143260386E-28,
-1.)) ;
#41456=DIRECTION('ref_axis',(0.707106781186552,0.707106781186543,1.53556032529733E-15)) ;
#41457=DIRECTION('',(-2.1716102378779E-15,3.83815143260386E-28,1.)) ;
#41458=DIRECTION('center_axis',(2.1716102378779E-15,-3.83815143260386E-28,
-1.)) ;
#41459=DIRECTION('ref_axis',(0.707106781186582,0.707106781186513,1.5355603252974E-15)) ;
#41460=DIRECTION('center_axis',(1.66533453692966E-16,1.,-3.83386399937507E-28)) ;
#41461=DIRECTION('ref_axis',(2.1716102378779E-15,-3.83748045690496E-28,
-1.)) ;
#41462=DIRECTION('',(2.17161023787787E-15,-3.83815143260382E-28,-1.)) ;
#41463=DIRECTION('',(1.,-1.66533453692966E-16,2.1716102378779E-15)) ;
#41464=DIRECTION('center_axis',(1.,-1.66533453692966E-16,-4.54195640846217E-14)) ;
#41465=DIRECTION('ref_axis',(3.19987248283774E-14,-0.707106781186434,0.707106781186661)) ;
#41466=DIRECTION('center_axis',(1.,0.,0.)) ;
#41467=DIRECTION('ref_axis',(0.,0.,1.)) ;
#41468=DIRECTION('',(1.,-1.66533453692966E-16,-4.54195640846217E-14)) ;
#41469=DIRECTION('center_axis',(-1.,0.,0.)) ;
#41470=DIRECTION('ref_axis',(0.,-1.,0.)) ;
#41471=DIRECTION('',(1.,-1.66533453692966E-16,-4.54195640846217E-14)) ;
#41472=DIRECTION('center_axis',(-4.54195640846217E-14,1.66321791214601E-16,
-1.)) ;
#41473=DIRECTION('ref_axis',(-1.,0.,4.54747350886464E-14)) ;
#41474=DIRECTION('center_axis',(0.,1.,0.)) ;
#41475=DIRECTION('ref_axis',(-1.,0.,5.32907051820105E-14)) ;
#41476=DIRECTION('center_axis',(4.54195640846217E-14,-1.66321791214601E-16,
1.)) ;
#41477=DIRECTION('ref_axis',(-1.,5.55236256206829E-46,4.54195640846217E-14)) ;
#41478=DIRECTION('center_axis',(2.1716102378779E-15,-3.83815143260386E-28,
-1.)) ;
#41479=DIRECTION('ref_axis',(0.707106781186552,0.707106781186543,1.53556032529733E-15)) ;
#41480=DIRECTION('center_axis',(-1.66533453692965E-16,-1.,-1.66321791214593E-16)) ;
#41481=DIRECTION('ref_axis',(-0.707106781186535,1.4966797377543E-19,0.70710678118656)) ;
#41482=DIRECTION('center_axis',(0.,1.,0.)) ;
#41483=DIRECTION('ref_axis',(-1.,0.,0.)) ;
#41484=DIRECTION('',(-1.66533453692965E-16,-1.,-1.66321791214593E-16)) ;
#41485=DIRECTION('',(-1.66533453692965E-16,-1.,-1.66321791214593E-16)) ;
#41486=DIRECTION('center_axis',(-4.54195640846217E-14,1.66321791214601E-16,
-1.)) ;
#41487=DIRECTION('ref_axis',(-1.,0.,4.54747350886464E-14)) ;
#41488=DIRECTION('center_axis',(1.,2.84217094304056E-13,0.)) ;
#41489=DIRECTION('ref_axis',(-2.84217094304056E-13,1.,0.)) ;
#41490=DIRECTION('center_axis',(4.54195640846217E-14,-1.66321791214601E-16,
1.)) ;
#41491=DIRECTION('ref_axis',(-1.,5.55236256206829E-46,4.54195640846217E-14)) ;
#41492=DIRECTION('center_axis',(-2.1716102378779E-15,3.83420712807775E-28,
1.)) ;
#41493=DIRECTION('ref_axis',(0.707106781186643,-0.707106781186452,1.53556032529807E-15)) ;
#41494=DIRECTION('center_axis',(-1.,1.66533453692587E-16,4.54195640846217E-14)) ;
#41495=DIRECTION('ref_axis',(3.22342386971791E-14,0.707106781186422,0.707106781186673)) ;
#41496=DIRECTION('center_axis',(1.,0.,0.)) ;
#41497=DIRECTION('ref_axis',(0.,1.,0.)) ;
#41498=DIRECTION('',(-1.,1.66533453692587E-16,4.54195640846217E-14)) ;
#41499=DIRECTION('',(-1.,1.66533453692587E-16,4.54195640846217E-14)) ;
#41500=DIRECTION('center_axis',(-4.54195640846217E-14,1.66321791214601E-16,
-1.)) ;
#41501=DIRECTION('ref_axis',(-1.,0.,4.54747350886464E-14)) ;
#41502=DIRECTION('center_axis',(0.,-1.,0.)) ;
#41503=DIRECTION('ref_axis',(1.,0.,-5.32907051820105E-14)) ;
#41504=DIRECTION('center_axis',(4.54195640846217E-14,-1.66321791214601E-16,
1.)) ;
#41505=DIRECTION('ref_axis',(-1.,5.55236256206829E-46,4.54195640846217E-14)) ;
#41506=DIRECTION('center_axis',(2.17161023787787E-15,-3.83420712807771E-28,
-1.)) ;
#41507=DIRECTION('ref_axis',(-0.707106781186552,-0.707106781186543,-1.53556032529731E-15)) ;
#41508=DIRECTION('center_axis',(8.32667268460786E-17,1.,1.66321791214597E-16)) ;
#41509=DIRECTION('ref_axis',(0.707106781186522,-1.76485733627007E-16,0.707106781186573)) ;
#41510=DIRECTION('center_axis',(0.,-1.,0.)) ;
#41511=DIRECTION('ref_axis',(1.,0.,1.77635683940035E-14)) ;
#41512=DIRECTION('',(8.32667268460786E-17,1.,1.66321791214597E-16)) ;
#41513=DIRECTION('center_axis',(-4.54195640846217E-14,1.66321791214601E-16,
-1.)) ;
#41514=DIRECTION('ref_axis',(-1.,0.,4.54747350886464E-14)) ;
#41515=DIRECTION('center_axis',(4.54195640846217E-14,-1.66321791214601E-16,
1.)) ;
#41516=DIRECTION('ref_axis',(-1.,5.55236256206829E-46,4.54195640846217E-14)) ;
#41517=DIRECTION('center_axis',(-2.17161023787787E-15,3.83815143260382E-28,
1.)) ;
#41518=DIRECTION('ref_axis',(-0.707106781186643,0.707106781186452,-1.53556032529805E-15)) ;
#41519=DIRECTION('center_axis',(-2.1716102378779E-15,3.83420712807775E-28,
1.)) ;
#41520=DIRECTION('ref_axis',(0.707106781186643,-0.707106781186452,1.53556032529807E-15)) ;
#41521=DIRECTION('',(-2.1716102378779E-15,3.83420712807775E-28,1.)) ;
#41522=DIRECTION('center_axis',(2.1716102378779E-15,-3.83420712807775E-28,
-1.)) ;
#41523=DIRECTION('ref_axis',(0.707106781186656,-0.707106781186439,1.5355603252981E-15)) ;
#41524=DIRECTION('',(-2.1716102378779E-15,3.83322105194623E-28,1.)) ;
#41525=DIRECTION('center_axis',(1.,-1.66533453692966E-16,2.1716102378779E-15)) ;
#41526=DIRECTION('ref_axis',(-1.66533453692966E-16,-1.,3.82783884128008E-28)) ;
#41527=DIRECTION('',(-2.1716102378779E-15,3.66854633798134E-28,1.)) ;
#41528=DIRECTION('center_axis',(1.,-1.66533453692966E-16,2.1716102378779E-15)) ;
#41529=DIRECTION('ref_axis',(-1.41780339089703E-15,0.707106781186483,0.707106781186612)) ;
#41530=DIRECTION('',(-1.66533453692966E-16,-1.,3.83386399937507E-28)) ;
#41531=DIRECTION('',(2.1716102378779E-15,-3.83815143260386E-28,-1.)) ;
#41532=DIRECTION('',(-1.66533453692966E-16,-1.,3.83386399937507E-28)) ;
#41533=DIRECTION('center_axis',(1.,-1.66533453692966E-16,2.1716102378779E-15)) ;
#41534=DIRECTION('ref_axis',(-1.65331725969844E-15,-0.707106781186479,0.707106781186616)) ;
#41535=DIRECTION('',(2.1716102378779E-15,-3.66854633798134E-28,-1.)) ;
#41536=DIRECTION('center_axis',(2.1716102378779E-15,-3.83815143260386E-28,
-1.)) ;
#41537=DIRECTION('ref_axis',(0.707106781186552,0.707106781186543,1.53556032529733E-15)) ;
#41538=DIRECTION('',(-2.1716102378779E-15,3.83815143260386E-28,1.)) ;
#41539=DIRECTION('center_axis',(2.1716102378779E-15,-3.83815143260386E-28,
-1.)) ;
#41540=DIRECTION('ref_axis',(0.707106781186582,0.707106781186513,1.5355603252974E-15)) ;
#41541=DIRECTION('center_axis',(1.66533453692966E-16,1.,-3.83386399937507E-28)) ;
#41542=DIRECTION('ref_axis',(2.1716102378779E-15,-3.83748045690496E-28,
-1.)) ;
#41543=DIRECTION('',(2.17161023787787E-15,-3.83815143260382E-28,-1.)) ;
#41544=DIRECTION('',(1.,-1.66533453692966E-16,2.1716102378779E-15)) ;
#41545=DIRECTION('center_axis',(1.,-1.66533453692966E-16,-4.54195640846217E-14)) ;
#41546=DIRECTION('ref_axis',(3.19987248283774E-14,-0.707106781186434,0.707106781186661)) ;
#41547=DIRECTION('center_axis',(1.,0.,0.)) ;
#41548=DIRECTION('ref_axis',(0.,0.,1.)) ;
#41549=DIRECTION('',(1.,-1.66533453692966E-16,-4.54195640846217E-14)) ;
#41550=DIRECTION('center_axis',(-1.,0.,0.)) ;
#41551=DIRECTION('ref_axis',(0.,-1.,0.)) ;
#41552=DIRECTION('',(1.,-1.66533453692966E-16,-4.54195640846217E-14)) ;
#41553=DIRECTION('center_axis',(-4.54195640846217E-14,1.66321791214601E-16,
-1.)) ;
#41554=DIRECTION('ref_axis',(-1.,0.,4.54747350886464E-14)) ;
#41555=DIRECTION('center_axis',(0.,1.,0.)) ;
#41556=DIRECTION('ref_axis',(-1.,0.,5.32907051820105E-14)) ;
#41557=DIRECTION('center_axis',(4.54195640846217E-14,-1.66321791214601E-16,
1.)) ;
#41558=DIRECTION('ref_axis',(-1.,5.55236256206829E-46,4.54195640846217E-14)) ;
#41559=DIRECTION('center_axis',(2.1716102378779E-15,-3.83815143260386E-28,
-1.)) ;
#41560=DIRECTION('ref_axis',(0.707106781186552,0.707106781186543,1.53556032529733E-15)) ;
#41561=DIRECTION('center_axis',(-1.66533453692965E-16,-1.,-1.66321791214593E-16)) ;
#41562=DIRECTION('ref_axis',(-0.707106781186535,1.4966797377543E-19,0.70710678118656)) ;
#41563=DIRECTION('center_axis',(0.,1.,0.)) ;
#41564=DIRECTION('ref_axis',(-1.,0.,0.)) ;
#41565=DIRECTION('',(-1.66533453692965E-16,-1.,-1.66321791214593E-16)) ;
#41566=DIRECTION('',(-1.66533453692965E-16,-1.,-1.66321791214593E-16)) ;
#41567=DIRECTION('center_axis',(-4.54195640846217E-14,1.66321791214601E-16,
-1.)) ;
#41568=DIRECTION('ref_axis',(-1.,0.,4.54747350886464E-14)) ;
#41569=DIRECTION('center_axis',(1.,2.84217094304056E-13,0.)) ;
#41570=DIRECTION('ref_axis',(-2.84217094304056E-13,1.,0.)) ;
#41571=DIRECTION('center_axis',(4.54195640846217E-14,-1.66321791214601E-16,
1.)) ;
#41572=DIRECTION('ref_axis',(-1.,5.55236256206829E-46,4.54195640846217E-14)) ;
#41573=DIRECTION('center_axis',(-2.1716102378779E-15,3.83420712807775E-28,
1.)) ;
#41574=DIRECTION('ref_axis',(0.707106781186643,-0.707106781186452,1.53556032529807E-15)) ;
#41575=DIRECTION('center_axis',(-1.,1.66533453692587E-16,4.54195640846217E-14)) ;
#41576=DIRECTION('ref_axis',(3.22342386971791E-14,0.707106781186422,0.707106781186673)) ;
#41577=DIRECTION('center_axis',(1.,0.,0.)) ;
#41578=DIRECTION('ref_axis',(0.,1.,0.)) ;
#41579=DIRECTION('',(-1.,1.66533453692587E-16,4.54195640846217E-14)) ;
#41580=DIRECTION('',(-1.,1.66533453692587E-16,4.54195640846217E-14)) ;
#41581=DIRECTION('center_axis',(-4.54195640846217E-14,1.66321791214601E-16,
-1.)) ;
#41582=DIRECTION('ref_axis',(-1.,0.,4.54747350886464E-14)) ;
#41583=DIRECTION('center_axis',(0.,-1.,0.)) ;
#41584=DIRECTION('ref_axis',(1.,0.,-5.32907051820105E-14)) ;
#41585=DIRECTION('center_axis',(4.54195640846217E-14,-1.66321791214601E-16,
1.)) ;
#41586=DIRECTION('ref_axis',(-1.,5.55236256206829E-46,4.54195640846217E-14)) ;
#41587=DIRECTION('center_axis',(2.17161023787787E-15,-3.83420712807771E-28,
-1.)) ;
#41588=DIRECTION('ref_axis',(-0.707106781186552,-0.707106781186543,-1.53556032529731E-15)) ;
#41589=DIRECTION('center_axis',(8.32667268460786E-17,1.,1.66321791214597E-16)) ;
#41590=DIRECTION('ref_axis',(0.707106781186522,-1.76485733627007E-16,0.707106781186573)) ;
#41591=DIRECTION('center_axis',(0.,-1.,0.)) ;
#41592=DIRECTION('ref_axis',(1.,0.,1.77635683940035E-14)) ;
#41593=DIRECTION('',(8.32667268460786E-17,1.,1.66321791214597E-16)) ;
#41594=DIRECTION('center_axis',(-4.54195640846217E-14,1.66321791214601E-16,
-1.)) ;
#41595=DIRECTION('ref_axis',(-1.,0.,4.54747350886464E-14)) ;
#41596=DIRECTION('center_axis',(4.54195640846217E-14,-1.66321791214601E-16,
1.)) ;
#41597=DIRECTION('ref_axis',(-1.,5.55236256206829E-46,4.54195640846217E-14)) ;
#41598=DIRECTION('center_axis',(-2.17161023787787E-15,3.83815143260382E-28,
1.)) ;
#41599=DIRECTION('ref_axis',(-0.707106781186643,0.707106781186452,-1.53556032529805E-15)) ;
#41600=DIRECTION('center_axis',(-2.1716102378779E-15,3.83420712807775E-28,
1.)) ;
#41601=DIRECTION('ref_axis',(0.707106781186643,-0.707106781186452,1.53556032529807E-15)) ;
#41602=DIRECTION('',(-2.1716102378779E-15,3.83420712807775E-28,1.)) ;
#41603=DIRECTION('center_axis',(2.1716102378779E-15,-3.83420712807775E-28,
-1.)) ;
#41604=DIRECTION('ref_axis',(0.707106781186656,-0.707106781186439,1.5355603252981E-15)) ;
#41605=DIRECTION('',(-2.1716102378779E-15,3.83322105194623E-28,1.)) ;
#41606=DIRECTION('center_axis',(1.,-1.66533453692966E-16,2.1716102378779E-15)) ;
#41607=DIRECTION('ref_axis',(-1.66533453692966E-16,-1.,3.82783884128008E-28)) ;
#41608=DIRECTION('',(-2.1716102378779E-15,3.66854633798134E-28,1.)) ;
#41609=DIRECTION('center_axis',(1.,-1.66533453692966E-16,2.1716102378779E-15)) ;
#41610=DIRECTION('ref_axis',(-1.41780339089703E-15,0.707106781186483,0.707106781186612)) ;
#41611=DIRECTION('',(-1.66533453692966E-16,-1.,3.83386399937507E-28)) ;
#41612=DIRECTION('',(2.1716102378779E-15,-3.83815143260386E-28,-1.)) ;
#41613=DIRECTION('',(-1.66533453692966E-16,-1.,3.83386399937507E-28)) ;
#41614=DIRECTION('center_axis',(1.,-1.66533453692966E-16,2.1716102378779E-15)) ;
#41615=DIRECTION('ref_axis',(-1.65331725969844E-15,-0.707106781186479,0.707106781186616)) ;
#41616=DIRECTION('',(2.1716102378779E-15,-3.66854633798134E-28,-1.)) ;
#41617=DIRECTION('center_axis',(2.1716102378779E-15,-3.83815143260386E-28,
-1.)) ;
#41618=DIRECTION('ref_axis',(0.707106781186552,0.707106781186543,1.53556032529733E-15)) ;
#41619=DIRECTION('',(-2.1716102378779E-15,3.83815143260386E-28,1.)) ;
#41620=DIRECTION('center_axis',(2.1716102378779E-15,-3.83815143260386E-28,
-1.)) ;
#41621=DIRECTION('ref_axis',(0.707106781186582,0.707106781186513,1.5355603252974E-15)) ;
#41622=DIRECTION('center_axis',(1.66533453692966E-16,1.,-3.83386399937507E-28)) ;
#41623=DIRECTION('ref_axis',(2.1716102378779E-15,-3.83748045690496E-28,
-1.)) ;
#41624=DIRECTION('',(2.17161023787787E-15,-3.83815143260382E-28,-1.)) ;
#41625=DIRECTION('',(1.,-1.66533453692966E-16,2.1716102378779E-15)) ;
#41626=DIRECTION('center_axis',(1.,-1.66533453692966E-16,-4.54195640846217E-14)) ;
#41627=DIRECTION('ref_axis',(3.19987248283774E-14,-0.707106781186434,0.707106781186661)) ;
#41628=DIRECTION('center_axis',(1.,0.,0.)) ;
#41629=DIRECTION('ref_axis',(0.,0.,1.)) ;
#41630=DIRECTION('',(1.,-1.66533453692966E-16,-4.54195640846217E-14)) ;
#41631=DIRECTION('center_axis',(-1.,0.,0.)) ;
#41632=DIRECTION('ref_axis',(0.,-1.,0.)) ;
#41633=DIRECTION('',(-1.,1.66533453692966E-16,4.54195640846217E-14)) ;
#41634=DIRECTION('center_axis',(-4.54195640846217E-14,1.66321791214601E-16,
-1.)) ;
#41635=DIRECTION('ref_axis',(-1.,0.,4.54747350886464E-14)) ;
#41636=DIRECTION('center_axis',(0.,1.,0.)) ;
#41637=DIRECTION('ref_axis',(-1.,0.,5.32907051820105E-14)) ;
#41638=DIRECTION('center_axis',(4.54195640846217E-14,-1.66321791214601E-16,
1.)) ;
#41639=DIRECTION('ref_axis',(0.707106781186502,0.707106781186593,-3.1998874496344E-14)) ;
#41640=DIRECTION('center_axis',(-4.54195640846217E-14,1.66321791214601E-16,
-1.)) ;
#41641=DIRECTION('ref_axis',(0.707106781186502,0.707106781186593,-3.1998874496344E-14)) ;
#41642=DIRECTION('center_axis',(-8.32667268460786E-17,-1.,-1.66321791214597E-16)) ;
#41643=DIRECTION('ref_axis',(-0.707106781186535,-5.87287992268677E-17,0.70710678118656)) ;
#41644=DIRECTION('center_axis',(0.,1.,0.)) ;
#41645=DIRECTION('ref_axis',(-1.,0.,0.)) ;
#41646=DIRECTION('',(8.32667268460786E-17,1.,1.66321791214597E-16)) ;
#41647=DIRECTION('',(-8.32667268460786E-17,-1.,-1.66321791214597E-16)) ;
#41648=DIRECTION('center_axis',(-4.54195640846217E-14,1.66321791214601E-16,
-1.)) ;
#41649=DIRECTION('ref_axis',(-1.,0.,4.54747350886464E-14)) ;
#41650=DIRECTION('center_axis',(1.,2.84217094304056E-13,0.)) ;
#41651=DIRECTION('ref_axis',(-2.84217094304056E-13,1.,0.)) ;
#41652=DIRECTION('center_axis',(4.54195640846217E-14,-1.66321791214601E-16,
1.)) ;
#41653=DIRECTION('ref_axis',(0.707106781186502,-0.707106781186593,-3.22340890291979E-14)) ;
#41654=DIRECTION('center_axis',(-4.54195640846217E-14,1.66321791214601E-16,
-1.)) ;
#41655=DIRECTION('ref_axis',(0.707106781186502,-0.707106781186593,-3.22340890291979E-14)) ;
#41656=DIRECTION('center_axis',(-1.,1.66533453692587E-16,4.54195640846217E-14)) ;
#41657=DIRECTION('ref_axis',(3.22342386971791E-14,0.707106781186422,0.707106781186673)) ;
#41658=DIRECTION('center_axis',(1.,0.,0.)) ;
#41659=DIRECTION('ref_axis',(0.,1.,0.)) ;
#41660=DIRECTION('',(1.,-1.66533453692587E-16,-4.54195640846217E-14)) ;
#41661=DIRECTION('',(-1.,1.66533453692587E-16,4.54195640846217E-14)) ;
#41662=DIRECTION('center_axis',(-4.54195640846217E-14,1.66321791214601E-16,
-1.)) ;
#41663=DIRECTION('ref_axis',(-1.,0.,4.54747350886464E-14)) ;
#41664=DIRECTION('center_axis',(0.,-1.,0.)) ;
#41665=DIRECTION('ref_axis',(1.,0.,-5.32907051820105E-14)) ;
#41666=DIRECTION('center_axis',(4.54195640846217E-14,-1.66321791214601E-16,
1.)) ;
#41667=DIRECTION('ref_axis',(-0.707106781186593,-0.707106781186502,3.19988744963481E-14)) ;
#41668=DIRECTION('center_axis',(-4.54195640846217E-14,1.66321791214601E-16,
-1.)) ;
#41669=DIRECTION('ref_axis',(-0.707106781186593,-0.707106781186502,3.19988744963481E-14)) ;
#41670=DIRECTION('center_axis',(1.66533453692965E-16,1.,1.66321791214593E-16)) ;
#41671=DIRECTION('ref_axis',(0.707106781186535,-2.35364200827643E-16,0.70710678118656)) ;
#41672=DIRECTION('center_axis',(0.,-1.,0.)) ;
#41673=DIRECTION('ref_axis',(1.,0.,0.)) ;
#41674=DIRECTION('',(-1.66533453692965E-16,-1.,-1.66321791214593E-16)) ;
#41675=DIRECTION('',(1.66533453692965E-16,1.,1.66321791214593E-16)) ;
#41676=DIRECTION('center_axis',(-4.54195640846217E-14,1.66321791214601E-16,
-1.)) ;
#41677=DIRECTION('ref_axis',(-1.,0.,4.54747350886464E-14)) ;
#41678=DIRECTION('center_axis',(4.54195640846217E-14,-1.66321791214601E-16,
1.)) ;
#41679=DIRECTION('ref_axis',(-0.707106781186735,0.70710678118636,3.22340890292084E-14)) ;
#41680=DIRECTION('center_axis',(-4.54195640846217E-14,1.66321791214601E-16,
-1.)) ;
#41681=DIRECTION('ref_axis',(-0.707106781186735,0.70710678118636,3.22340890292084E-14)) ;
#41682=DIRECTION('center_axis',(-2.17161023787787E-15,3.83420712807771E-28,
1.)) ;
#41683=DIRECTION('ref_axis',(0.707106781186543,-0.707106781186552,1.53556032529783E-15)) ;
#41684=DIRECTION('',(-2.17161023787787E-15,3.83420712807771E-28,1.)) ;
#41685=DIRECTION('center_axis',(2.17161023787792E-15,-2.90739654573749E-15,
-1.)) ;
#41686=DIRECTION('ref_axis',(1.35627620245787E-13,-1.,2.90739654573778E-15)) ;
#41687=DIRECTION('',(2.17161023787787E-15,-3.83420712807771E-28,-1.)) ;
#41688=DIRECTION('center_axis',(1.,-8.32667268460789E-17,2.17161023787787E-15)) ;
#41689=DIRECTION('ref_axis',(-8.32667268460789E-17,-1.,3.92101138914083E-28)) ;
#41690=DIRECTION('',(2.17161023787787E-15,-3.83815143260382E-28,-1.)) ;
#41691=DIRECTION('',(-8.32667268460789E-17,-1.,3.83780830390118E-28)) ;
#41692=DIRECTION('center_axis',(2.17161023787787E-15,-3.83815143260382E-28,
-1.)) ;
#41693=DIRECTION('ref_axis',(0.707106781186452,0.707106781186643,1.53556032529709E-15)) ;
#41694=DIRECTION('',(-2.17161023787787E-15,3.83815143260382E-28,1.)) ;
#41695=DIRECTION('center_axis',(2.17161023787746E-15,-7.39616701217516E-14,
-1.)) ;
#41696=DIRECTION('ref_axis',(1.,-6.48092690624108E-15,2.17161023787794E-15)) ;
#41697=DIRECTION('center_axis',(1.66533453692966E-16,1.,-3.83386399937507E-28)) ;
#41698=DIRECTION('ref_axis',(2.1716102378779E-15,-3.83748045690496E-28,
-1.)) ;
#41699=DIRECTION('',(2.1716102378779E-15,-3.83815143260386E-28,-1.)) ;
#41700=DIRECTION('',(1.,-1.66533453692966E-16,2.1716102378779E-15)) ;
#41701=DIRECTION('center_axis',(4.54195640846217E-14,-1.66321791214601E-16,
1.)) ;
#41702=DIRECTION('ref_axis',(1.75658099177411E-13,1.,1.66321791206623E-16)) ;
#41703=DIRECTION('',(-1.,1.75658099177411E-13,4.54195640846217E-14)) ;
#41704=DIRECTION('',(1.75658099177411E-13,1.,1.66321791206623E-16)) ;
#41705=DIRECTION('',(1.,-1.75658099177411E-13,-4.54195640846217E-14)) ;
#41706=DIRECTION('',(-1.75658099177411E-13,-1.,-1.66321791206623E-16)) ;
#41707=DIRECTION('',(-1.,1.66533453692966E-16,4.54195640846217E-14)) ;
#41708=DIRECTION('center_axis',(4.54195640846217E-14,-1.66321791214601E-16,
1.)) ;
#41709=DIRECTION('ref_axis',(0.707106781186502,0.707106781186593,-3.1998874496344E-14)) ;
#41710=DIRECTION('',(1.66533453692965E-16,1.,1.66321791214593E-16)) ;
#41711=DIRECTION('center_axis',(4.54195640846217E-14,-1.66321791214601E-16,
1.)) ;
#41712=DIRECTION('ref_axis',(0.707106781186644,-0.707106781186451,-3.22340890292043E-14)) ;
#41713=DIRECTION('',(1.,-1.66533453692587E-16,-4.54195640846217E-14)) ;
#41714=DIRECTION('center_axis',(4.54195640846217E-14,-1.66321791214601E-16,
1.)) ;
#41715=DIRECTION('ref_axis',(-0.707106781186593,-0.707106781186502,3.19988744963481E-14)) ;
#41716=DIRECTION('',(-8.32667268460786E-17,-1.,-1.66321791214597E-16)) ;
#41717=DIRECTION('center_axis',(4.54195640846217E-14,-1.66321791214601E-16,
1.)) ;
#41718=DIRECTION('ref_axis',(-0.707106781186735,0.70710678118636,3.22340890292084E-14)) ;
#41719=DIRECTION('center_axis',(-2.16239769233719E-14,8.31608956071042E-17,
-1.)) ;
#41720=DIRECTION('ref_axis',(1.,-9.64599832246215E-47,-2.16239769233719E-14)) ;
#41721=DIRECTION('center_axis',(1.,-1.66533453692966E-16,-4.54195640846217E-14)) ;
#41722=DIRECTION('ref_axis',(3.19987248283774E-14,-0.707106781186434,0.707106781186661)) ;
#41723=DIRECTION('center_axis',(1.,0.,0.)) ;
#41724=DIRECTION('ref_axis',(0.,0.,1.)) ;
#41725=DIRECTION('',(1.,-1.66533453692966E-16,-4.54195640846217E-14)) ;
#41726=DIRECTION('center_axis',(-1.,0.,0.)) ;
#41727=DIRECTION('ref_axis',(0.,-1.,0.)) ;
#41728=DIRECTION('center_axis',(-4.54195640846217E-14,1.66321791214601E-16,
-1.)) ;
#41729=DIRECTION('ref_axis',(-1.,0.,4.54747350886464E-14)) ;
#41730=DIRECTION('center_axis',(0.,1.,0.)) ;
#41731=DIRECTION('ref_axis',(-1.,0.,5.32907051820105E-14)) ;
#41732=DIRECTION('center_axis',(-4.54195640846217E-14,1.66321791214601E-16,
-1.)) ;
#41733=DIRECTION('ref_axis',(0.707106781186502,0.707106781186593,-3.1998874496344E-14)) ;
#41734=DIRECTION('center_axis',(-1.66533453692965E-16,-1.,-1.66321791214593E-16)) ;
#41735=DIRECTION('ref_axis',(-0.707106781186535,1.4966797377543E-19,0.70710678118656)) ;
#41736=DIRECTION('center_axis',(0.,1.,0.)) ;
#41737=DIRECTION('ref_axis',(-1.,0.,0.)) ;
#41738=DIRECTION('',(-1.66533453692965E-16,-1.,-1.66321791214593E-16)) ;
#41739=DIRECTION('center_axis',(-4.54195640846217E-14,1.66321791214601E-16,
-1.)) ;
#41740=DIRECTION('ref_axis',(-1.,0.,4.54747350886464E-14)) ;
#41741=DIRECTION('center_axis',(1.,2.84217094304056E-13,0.)) ;
#41742=DIRECTION('ref_axis',(-2.84217094304056E-13,1.,0.)) ;
#41743=DIRECTION('center_axis',(-4.54195640846217E-14,1.66321791214601E-16,
-1.)) ;
#41744=DIRECTION('ref_axis',(0.707106781186644,-0.707106781186451,-3.22340890292043E-14)) ;
#41745=DIRECTION('center_axis',(-1.,1.66533453692587E-16,4.54195640846217E-14)) ;
#41746=DIRECTION('ref_axis',(3.22342386971791E-14,0.707106781186422,0.707106781186673)) ;
#41747=DIRECTION('center_axis',(1.,0.,0.)) ;
#41748=DIRECTION('ref_axis',(0.,1.,0.)) ;
#41749=DIRECTION('',(-1.,1.66533453692587E-16,4.54195640846217E-14)) ;
#41750=DIRECTION('center_axis',(-4.54195640846217E-14,1.66321791214601E-16,
-1.)) ;
#41751=DIRECTION('ref_axis',(-1.,0.,4.54747350886464E-14)) ;
#41752=DIRECTION('center_axis',(0.,-1.,0.)) ;
#41753=DIRECTION('ref_axis',(1.,0.,-5.32907051820105E-14)) ;
#41754=DIRECTION('center_axis',(-4.54195640846217E-14,1.66321791214601E-16,
-1.)) ;
#41755=DIRECTION('ref_axis',(-0.707106781186593,-0.707106781186502,3.19988744963481E-14)) ;
#41756=DIRECTION('center_axis',(8.32667268460786E-17,1.,1.66321791214597E-16)) ;
#41757=DIRECTION('ref_axis',(0.707106781186522,-1.76485733627007E-16,0.707106781186573)) ;
#41758=DIRECTION('center_axis',(0.,-1.,0.)) ;
#41759=DIRECTION('ref_axis',(1.,0.,1.77635683940035E-14)) ;
#41760=DIRECTION('center_axis',(-4.54195640846217E-14,1.66321791214601E-16,
-1.)) ;
#41761=DIRECTION('ref_axis',(-1.,0.,4.54747350886464E-14)) ;
#41762=DIRECTION('center_axis',(-4.54195640846217E-14,1.66321791214601E-16,
-1.)) ;
#41763=DIRECTION('ref_axis',(-0.707106781186735,0.70710678118636,3.22340890292084E-14)) ;
#41764=DIRECTION('center_axis',(-2.1716102378779E-15,3.83420712807775E-28,
1.)) ;
#41765=DIRECTION('ref_axis',(0.707106781186643,-0.707106781186452,1.53556032529807E-15)) ;
#41766=DIRECTION('',(-2.1716102378779E-15,3.83420712807775E-28,1.)) ;
#41767=DIRECTION('center_axis',(2.1716102378779E-15,-3.83420712807775E-28,
-1.)) ;
#41768=DIRECTION('ref_axis',(0.707106781186656,-0.707106781186439,1.5355603252981E-15)) ;
#41769=DIRECTION('',(-2.1716102378779E-15,3.83322105194623E-28,1.)) ;
#41770=DIRECTION('center_axis',(1.,-1.66533453692966E-16,2.1716102378779E-15)) ;
#41771=DIRECTION('ref_axis',(-1.66533453692966E-16,-1.,3.82783884128008E-28)) ;
#41772=DIRECTION('',(2.1716102378779E-15,-3.83815143260386E-28,-1.)) ;
#41773=DIRECTION('',(-1.66533453692966E-16,-1.,3.83386399937507E-28)) ;
#41774=DIRECTION('center_axis',(1.,-1.66533453692966E-16,2.1716102378779E-15)) ;
#41775=DIRECTION('ref_axis',(-1.65331725969844E-15,-0.707106781186479,0.707106781186616)) ;
#41776=DIRECTION('',(2.1716102378779E-15,-3.66854633798134E-28,-1.)) ;
#41777=DIRECTION('',(-2.1716102378779E-15,3.66854633798134E-28,1.)) ;
#41778=DIRECTION('center_axis',(1.,-1.66533453692966E-16,2.1716102378779E-15)) ;
#41779=DIRECTION('ref_axis',(-1.41780339089703E-15,0.707106781186483,0.707106781186612)) ;
#41780=DIRECTION('',(-1.66533453692966E-16,-1.,3.83386399937507E-28)) ;
#41781=DIRECTION('center_axis',(2.1716102378779E-15,-3.83815143260386E-28,
-1.)) ;
#41782=DIRECTION('ref_axis',(0.707106781186552,0.707106781186543,1.53556032529733E-15)) ;
#41783=DIRECTION('',(2.1716102378779E-15,-3.83815143260386E-28,-1.)) ;
#41784=DIRECTION('center_axis',(2.1716102378779E-15,-3.83815143260386E-28,
-1.)) ;
#41785=DIRECTION('ref_axis',(0.707106781186582,0.707106781186513,1.5355603252974E-15)) ;
#41786=DIRECTION('center_axis',(1.66533453692966E-16,1.,-3.83386399937507E-28)) ;
#41787=DIRECTION('ref_axis',(2.1716102378779E-15,-3.83748045690496E-28,
-1.)) ;
#41788=DIRECTION('',(2.17161023787787E-15,-3.83815143260382E-28,-1.)) ;
#41789=DIRECTION('',(1.,-1.66533453692966E-16,2.1716102378779E-15)) ;
#41790=DIRECTION('center_axis',(-1.66533453692587E-16,-1.,3.82991969484897E-28)) ;
#41791=DIRECTION('ref_axis',(2.1716102378779E-15,-3.83353615237885E-28,
-1.)) ;
#41792=DIRECTION('',(-1.,1.66533453692587E-16,-2.1716102378779E-15)) ;
#41793=DIRECTION('',(-2.17161023787787E-15,3.83420712807771E-28,1.)) ;
#41794=DIRECTION('center_axis',(2.17161023787787E-15,-3.83420712807771E-28,
-1.)) ;
#41795=DIRECTION('ref_axis',(-0.707106781186552,-0.707106781186543,-1.53556032529731E-15)) ;
#41796=DIRECTION('center_axis',(2.17161023787787E-15,-3.83420712807771E-28,
-1.)) ;
#41797=DIRECTION('ref_axis',(-0.707106781186582,-0.707106781186513,-1.53556032529738E-15)) ;
#41798=DIRECTION('center_axis',(-2.17161023787787E-15,3.83815143260382E-28,
1.)) ;
#41799=DIRECTION('ref_axis',(-0.707106781186643,0.707106781186452,-1.53556032529805E-15)) ;
#41800=DIRECTION('center_axis',(2.17161023787787E-15,-3.83815143260382E-28,
-1.)) ;
#41801=DIRECTION('ref_axis',(-0.707106781186656,0.707106781186439,-1.53556032529808E-15)) ;
#41802=DIRECTION('center_axis',(-1.66533453692587E-16,-1.,3.82991969484897E-28)) ;
#41803=DIRECTION('ref_axis',(2.1716102378779E-15,-3.83353615237885E-28,
-1.)) ;
#41804=DIRECTION('',(-1.,1.66533453692587E-16,-2.1716102378779E-15)) ;
#41805=DIRECTION('',(-2.1716102378779E-15,3.83420712807775E-28,1.)) ;
#41806=DIRECTION('center_axis',(2.1716102378779E-15,-3.83420712807775E-28,
-1.)) ;
#41807=DIRECTION('ref_axis',(-0.707106781186452,-0.707106781186643,-1.53556032529712E-15)) ;
#41808=DIRECTION('center_axis',(2.1716102378779E-15,-3.83420712807775E-28,
-1.)) ;
#41809=DIRECTION('ref_axis',(-0.70710678118651,-0.707106781186585,-1.53556032529724E-15)) ;
#41810=DIRECTION('',(2.1716102378779E-15,-3.83420712807775E-28,-1.)) ;
#41811=DIRECTION('center_axis',(-2.1716102378779E-15,3.83815143260386E-28,
1.)) ;
#41812=DIRECTION('ref_axis',(-0.707106781186643,0.707106781186452,-1.53556032529807E-15)) ;
#41813=DIRECTION('',(-2.1716102378779E-15,3.83815143260386E-28,1.)) ;
#41814=DIRECTION('center_axis',(2.1716102378779E-15,-3.83815143260386E-28,
-1.)) ;
#41815=DIRECTION('ref_axis',(-0.707106781186656,0.707106781186439,-1.5355603252981E-15)) ;
#41816=DIRECTION('center_axis',(-1.,1.66533453692966E-16,-2.1716102378779E-15)) ;
#41817=DIRECTION('ref_axis',(1.66533453692966E-16,1.,-3.82783884128008E-28)) ;
#41818=DIRECTION('',(1.66533453692966E-16,1.,-3.83386399937507E-28)) ;
#41819=DIRECTION('center_axis',(2.1716102378779E-15,-3.83815143260386E-28,
-1.)) ;
#41820=DIRECTION('ref_axis',(1.,-1.66533453692941E-16,2.1716102378779E-15)) ;
#41821=DIRECTION('center_axis',(-2.1716102378779E-15,3.83815143260386E-28,
1.)) ;
#41822=DIRECTION('ref_axis',(-1.,-7.33033736753389E-16,-2.1716102378779E-15)) ;
#41823=DIRECTION('center_axis',(-2.1716102378779E-15,3.66854633798134E-28,
1.)) ;
#41824=DIRECTION('ref_axis',(0.707106781186452,0.707106781186643,1.53556032529713E-15)) ;
#41825=DIRECTION('center_axis',(1.88526971141291E-28,-2.90739654573716E-15,
-1.)) ;
#41826=DIRECTION('ref_axis',(-1.35627620245787E-13,1.,-2.90739654573716E-15)) ;
#41827=DIRECTION('center_axis',(1.,-1.66533453692587E-16,2.1716102378779E-15)) ;
#41828=DIRECTION('ref_axis',(1.41780339089714E-15,-0.70710678118655,-0.707106781186545)) ;
#41829=DIRECTION('center_axis',(1.,1.35627620245787E-13,-2.05796303467862E-28)) ;
#41830=DIRECTION('ref_axis',(1.35627620245787E-13,-1.,2.90739654573716E-15)) ;
#41831=DIRECTION('center_axis',(-1.,-1.35627620245747E-13,2.05796303467745E-28)) ;
#41832=DIRECTION('ref_axis',(1.88526971141291E-28,-2.90739654573716E-15,
-1.)) ;
#41833=DIRECTION('',(1.,-1.66533453692587E-16,2.1716102378779E-15)) ;
#41834=DIRECTION('center_axis',(-1.,6.48092690624107E-15,-2.07369595641671E-28)) ;
#41835=DIRECTION('ref_axis',(0.,-1.,0.)) ;
#41836=DIRECTION('center_axis',(-1.,7.08071943160919E-13,-2.24717289282075E-27)) ;
#41837=DIRECTION('ref_axis',(-1.88526971141296E-28,2.90739654573716E-15,
1.)) ;
#41838=DIRECTION('center_axis',(6.48092690624107E-15,1.,-2.90739654573716E-15)) ;
#41839=DIRECTION('ref_axis',(1.,-6.48092690624107E-15,2.07369595641671E-28)) ;
#41840=DIRECTION('center_axis',(-1.66533453692966E-16,-1.,3.83386399937507E-28)) ;
#41841=DIRECTION('ref_axis',(0.707106781186648,-1.17756934401E-16,-0.707106781186447)) ;
#41842=DIRECTION('center_axis',(-6.48092690624107E-15,-1.,2.90739654573716E-15)) ;
#41843=DIRECTION('ref_axis',(1.88526971141291E-28,-2.90739654573716E-15,
-1.)) ;
#41844=DIRECTION('',(1.66533453692966E-16,1.,-3.83386399937507E-28)) ;
#41845=DIRECTION('center_axis',(1.,-6.48092690624107E-15,2.07369595641671E-28)) ;
#41846=DIRECTION('ref_axis',(0.,1.,0.)) ;
#41847=DIRECTION('center_axis',(1.,-1.48589474058271E-13,-5.59482469102492E-13)) ;
#41848=DIRECTION('ref_axis',(-1.48589474058269E-13,-1.,2.90739654573716E-15)) ;
#41849=DIRECTION('center_axis',(6.48092690624107E-15,1.,-2.90739654573716E-15)) ;
#41850=DIRECTION('ref_axis',(1.88526971141291E-28,-2.90739654573716E-15,
-1.)) ;
#41851=DIRECTION('center_axis',(-1.,6.48092690624107E-15,-2.07369595641671E-28)) ;
#41852=DIRECTION('ref_axis',(0.,-1.,0.)) ;
#41853=DIRECTION('center_axis',(-1.,1.48589474058269E-13,-6.20535494751205E-28)) ;
#41854=DIRECTION('ref_axis',(1.48589474058269E-13,1.,-2.90739654573716E-15)) ;
#41855=DIRECTION('center_axis',(-6.48092690624107E-15,-1.,2.90739654573716E-15)) ;
#41856=DIRECTION('ref_axis',(1.88526971141291E-28,-2.90739654573716E-15,
-1.)) ;
#41857=DIRECTION('center_axis',(1.88526971141291E-28,-2.90739654573716E-15,
-1.)) ;
#41858=DIRECTION('ref_axis',(1.,-6.48092690624108E-15,2.07369595641671E-28)) ;
#41859=DIRECTION('center_axis',(2.1716102378779E-15,-3.66854633798134E-28,
-1.)) ;
#41860=DIRECTION('ref_axis',(0.707106781186543,-0.707106781186552,1.53556032529784E-15)) ;
#41861=DIRECTION('',(2.1716102378779E-15,-3.66854633798134E-28,-1.)) ;
#41862=DIRECTION('center_axis',(-1.66533453692966E-16,-1.,3.83386399937507E-28)) ;
#41863=DIRECTION('ref_axis',(0.707106781186648,-1.17756934401E-16,-0.707106781186447)) ;
#41864=DIRECTION('center_axis',(6.48092690628146E-15,1.,-2.90739654573716E-15)) ;
#41865=DIRECTION('ref_axis',(1.,-6.48092690628146E-15,2.07369595641789E-28)) ;
#41866=DIRECTION('',(1.66533453692966E-16,1.,-3.83386399937507E-28)) ;
#41867=DIRECTION('center_axis',(1.,-6.48092690624107E-15,2.07369595641671E-28)) ;
#41868=DIRECTION('ref_axis',(0.,1.,0.)) ;
#41869=DIRECTION('center_axis',(1.,-1.48589474058269E-13,6.20535494751205E-28)) ;
#41870=DIRECTION('ref_axis',(-1.88526971141292E-28,2.90739654573716E-15,
1.)) ;
#41871=DIRECTION('center_axis',(-6.48092690624107E-15,-1.,2.90739654573716E-15)) ;
#41872=DIRECTION('ref_axis',(-1.,6.48092690624107E-15,-2.07369595641671E-28)) ;
#41873=DIRECTION('center_axis',(8.32667268460789E-17,1.,-3.83780830390118E-28)) ;
#41874=DIRECTION('ref_axis',(-0.707106781186447,5.88784671997906E-17,-0.707106781186648)) ;
#41875=DIRECTION('center_axis',(6.48092690624107E-15,1.,-2.90739654573716E-15)) ;
#41876=DIRECTION('ref_axis',(1.88526971141291E-28,-2.90739654573716E-15,
-1.)) ;
#41877=DIRECTION('',(-8.32667268460789E-17,-1.,3.83780830390118E-28)) ;
#41878=DIRECTION('center_axis',(-1.,3.33066907386739E-16,-2.1716102378779E-15)) ;
#41879=DIRECTION('ref_axis',(-1.30004645649559E-15,0.70710678118655,0.707106781186545)) ;
#41880=DIRECTION('',(-1.,3.33066907386739E-16,-2.1716102378779E-15)) ;
#41881=DIRECTION('',(1.,-3.33066907386739E-16,2.1716102378779E-15)) ;
#41882=DIRECTION('center_axis',(8.32667268460789E-17,1.,-3.83780830390118E-28)) ;
#41883=DIRECTION('ref_axis',(-0.707106781186447,5.88784671997906E-17,-0.707106781186648)) ;
#41884=DIRECTION('center_axis',(-6.48092690624107E-15,-1.,2.90739654573716E-15)) ;
#41885=DIRECTION('ref_axis',(-1.,6.48092690624107E-15,-2.07369595641671E-28)) ;
#41886=DIRECTION('',(-8.32667268460789E-17,-1.,3.83780830390118E-28)) ;
#41887=DIRECTION('center_axis',(1.,-3.33066907386739E-16,2.1716102378779E-15)) ;
#41888=DIRECTION('ref_axis',(-1.77107419409959E-15,-0.707106781186545,0.70710678118655)) ;
#41889=DIRECTION('',(1.,-3.33066907386739E-16,2.1716102378779E-15)) ;
#41890=DIRECTION('center_axis',(-0.81649658092765,0.408248290464166,0.408248290463711)) ;
#41891=DIRECTION('ref_axis',(-0.577350269189702,-0.577350269189929,-0.577350269189247)) ;
#41892=DIRECTION('center_axis',(-0.40824829046392,0.408248290464147,-0.816496580927556)) ;
#41893=DIRECTION('ref_axis',(0.577350269189076,-0.577350269189986,-0.577350269189815)) ;
#41894=DIRECTION('center_axis',(1.,-1.66533453692966E-16,2.1716102378779E-15)) ;
#41895=DIRECTION('ref_axis',(1.65331725969831E-15,0.707106781186545,-0.70710678118655)) ;
#41896=DIRECTION('center_axis',(1.,1.35627620245787E-13,-2.05796303467862E-28)) ;
#41897=DIRECTION('ref_axis',(1.8852697114129E-28,-2.90739654573716E-15,
-1.)) ;
#41898=DIRECTION('',(-1.,1.66533453692966E-16,-2.1716102378779E-15)) ;
#41899=DIRECTION('center_axis',(-1.,-1.35627620245787E-13,2.05796303467862E-28)) ;
#41900=DIRECTION('ref_axis',(-1.35627620245787E-13,1.,-2.90739654573716E-15)) ;
#41901=DIRECTION('center_axis',(0.40824829046392,-0.408248290464147,-0.816496580927556)) ;
#41902=DIRECTION('ref_axis',(-0.577350269189834,0.577350269189152,-0.577350269189891)) ;
#41903=DIRECTION('center_axis',(-0.81649658092765,0.408248290464166,-0.408248290463711)) ;
#41904=DIRECTION('ref_axis',(0.577350269189702,0.577350269189929,-0.577350269189247)) ;
#41905=DIRECTION('center_axis',(-3.33066907386739E-16,-1.,3.66031460022645E-28)) ;
#41906=DIRECTION('ref_axis',(-2.17161023787795E-15,3.66754751528624E-28,
1.)) ;
#41907=DIRECTION('center_axis',(2.1716102378779E-15,-3.83815143260386E-28,
-1.)) ;
#41908=DIRECTION('ref_axis',(1.,-1.66533453692941E-16,2.1716102378779E-15)) ;
#41909=DIRECTION('center_axis',(2.1716102378779E-15,-3.83815143260386E-28,
-1.)) ;
#41910=DIRECTION('ref_axis',(1.,-1.66533453692941E-16,2.1716102378779E-15)) ;
#41911=DIRECTION('center_axis',(2.1716102378779E-15,-3.83815143260386E-28,
-1.)) ;
#41912=DIRECTION('ref_axis',(1.,-1.66533453692941E-16,2.1716102378779E-15)) ;
#41913=DIRECTION('',(-1.66533453692966E-16,-1.,3.83386399937507E-28)) ;
#41914=DIRECTION('',(1.,-1.66533453692587E-16,2.1716102378779E-15)) ;
#41915=DIRECTION('',(8.32667268460789E-17,1.,-3.83780830390118E-28)) ;
#41916=DIRECTION('',(-1.,1.66533453692966E-16,-2.1716102378779E-15)) ;
#41917=DIRECTION('center_axis',(-0.816496580927764,0.408248290464109,0.408248290463541)) ;
#41918=DIRECTION('ref_axis',(-0.577350269189531,-0.577350269189986,-0.57735026918936)) ;
#41919=DIRECTION('center_axis',(1.,1.35627620245787E-13,2.17161023787752E-15)) ;
#41920=DIRECTION('ref_axis',(1.35627620245787E-13,-1.,2.90739654573778E-15)) ;
#41921=DIRECTION('center_axis',(6.48092690624107E-15,1.,-2.90739654573747E-15)) ;
#41922=DIRECTION('ref_axis',(2.17161023787792E-15,-2.90739654573748E-15,
-1.)) ;
#41923=DIRECTION('center_axis',(0.40824829046392,-0.408248290464147,-0.816496580927556)) ;
#41924=DIRECTION('ref_axis',(-0.577350269189986,0.577350269189076,-0.577350269189815)) ;
#41925=DIRECTION('center_axis',(-6.48092690624107E-15,-1.,2.90739654573747E-15)) ;
#41926=DIRECTION('ref_axis',(-1.,6.48092690624106E-15,-2.17161023787794E-15)) ;
#41927=DIRECTION('center_axis',(1.,1.35627620245787E-13,2.17161023787752E-15)) ;
#41928=DIRECTION('ref_axis',(2.17161023787791E-15,-2.90739654573749E-15,
-1.)) ;
#41929=DIRECTION('center_axis',(1.66533453692966E-16,1.,-3.83386399937507E-28)) ;
#41930=DIRECTION('ref_axis',(-0.707106781186596,1.17756934400449E-16,-0.707106781186499)) ;
#41931=DIRECTION('center_axis',(1.,-1.66533453692966E-16,2.1716102378779E-15)) ;
#41932=DIRECTION('ref_axis',(1.65331725969841E-15,0.707106781186495,-0.7071067811866)) ;
#41933=DIRECTION('center_axis',(1.,1.35627620245787E-13,2.17161023787752E-15)) ;
#41934=DIRECTION('ref_axis',(-1.35627620245787E-13,1.,-2.90739654573778E-15)) ;
#41935=DIRECTION('center_axis',(-1.,1.66533453692587E-16,-2.1716102378779E-15)) ;
#41936=DIRECTION('ref_axis',(1.41780339089726E-15,-0.707106781186499,-0.707106781186596)) ;
#41937=DIRECTION('center_axis',(1.,1.35627620245787E-13,2.17161023787752E-15)) ;
#41938=DIRECTION('ref_axis',(2.17161023787792E-15,-2.90739654573749E-15,
-1.)) ;
#41939=DIRECTION('center_axis',(-8.32667268460789E-17,-1.,3.83780830390118E-28)) ;
#41940=DIRECTION('ref_axis',(0.707106781186599,-5.8878467200346E-17,-0.707106781186496)) ;
#41941=DIRECTION('center_axis',(-6.48092690624107E-15,-1.,2.90739654573747E-15)) ;
#41942=DIRECTION('ref_axis',(1.,-6.48092690624106E-15,2.17161023787794E-15)) ;
#41943=DIRECTION('center_axis',(6.48092690624107E-15,1.,-2.90739654573747E-15)) ;
#41944=DIRECTION('ref_axis',(2.17161023787792E-15,-2.90739654573748E-15,
-1.)) ;
#41945=DIRECTION('center_axis',(-0.408248290463939,0.408248290464166,-0.816496580927537)) ;
#41946=DIRECTION('ref_axis',(0.577350269189076,-0.577350269189986,-0.577350269189815)) ;
#41947=DIRECTION('center_axis',(0.408248290463948,-0.816496580927442,-0.408248290464346)) ;
#41948=DIRECTION('ref_axis',(0.577350269189304,0.577350269189986,-0.577350269189588)) ;
#41949=DIRECTION('center_axis',(-2.1716102378779E-15,3.66854633798134E-28,
1.)) ;
#41950=DIRECTION('ref_axis',(0.707106781186452,0.707106781186643,1.53556032529713E-15)) ;
#41951=DIRECTION('center_axis',(1.88526971141291E-28,-2.90739654573716E-15,
-1.)) ;
#41952=DIRECTION('ref_axis',(-1.35627620245787E-13,1.,-2.90739654573716E-15)) ;
#41953=DIRECTION('center_axis',(1.,-1.66533453692587E-16,2.1716102378779E-15)) ;
#41954=DIRECTION('ref_axis',(1.41780339089714E-15,-0.70710678118655,-0.707106781186545)) ;
#41955=DIRECTION('center_axis',(1.,1.35627620245787E-13,-2.05796303467862E-28)) ;
#41956=DIRECTION('ref_axis',(1.35627620245787E-13,-1.,2.90739654573716E-15)) ;
#41957=DIRECTION('',(-1.,1.66533453692587E-16,-2.1716102378779E-15)) ;
#41958=DIRECTION('center_axis',(-1.,-1.35627620245747E-13,2.05796303467745E-28)) ;
#41959=DIRECTION('ref_axis',(1.88526971141291E-28,-2.90739654573716E-15,
-1.)) ;
#41960=DIRECTION('',(1.,-1.66533453692587E-16,2.1716102378779E-15)) ;
#41961=DIRECTION('center_axis',(-1.,6.48092690624107E-15,-2.07369595641671E-28)) ;
#41962=DIRECTION('ref_axis',(0.,-1.,0.)) ;
#41963=DIRECTION('center_axis',(-1.,7.08071943160919E-13,-2.24717289282075E-27)) ;
#41964=DIRECTION('ref_axis',(-1.88526971141296E-28,2.90739654573716E-15,
1.)) ;
#41965=DIRECTION('center_axis',(6.48092690624107E-15,1.,-2.90739654573716E-15)) ;
#41966=DIRECTION('ref_axis',(1.,-6.48092690624107E-15,2.07369595641671E-28)) ;
#41967=DIRECTION('center_axis',(-1.66533453692966E-16,-1.,3.83386399937507E-28)) ;
#41968=DIRECTION('ref_axis',(0.707106781186648,-1.17756934401E-16,-0.707106781186447)) ;
#41969=DIRECTION('center_axis',(-6.48092690624107E-15,-1.,2.90739654573716E-15)) ;
#41970=DIRECTION('ref_axis',(1.88526971141291E-28,-2.90739654573716E-15,
-1.)) ;
#41971=DIRECTION('',(1.66533453692966E-16,1.,-3.83386399937507E-28)) ;
#41972=DIRECTION('center_axis',(1.,-6.48092690624107E-15,2.07369595641671E-28)) ;
#41973=DIRECTION('ref_axis',(0.,1.,0.)) ;
#41974=DIRECTION('center_axis',(1.,-1.48589474058271E-13,-5.59482469102492E-13)) ;
#41975=DIRECTION('ref_axis',(-1.48589474058269E-13,-1.,2.90739654573716E-15)) ;
#41976=DIRECTION('center_axis',(6.48092690624107E-15,1.,-2.90739654573716E-15)) ;
#41977=DIRECTION('ref_axis',(1.88526971141291E-28,-2.90739654573716E-15,
-1.)) ;
#41978=DIRECTION('center_axis',(-1.,6.48092690624107E-15,-2.07369595641671E-28)) ;
#41979=DIRECTION('ref_axis',(0.,-1.,0.)) ;
#41980=DIRECTION('center_axis',(-1.,1.48589474058269E-13,-6.20535494751205E-28)) ;
#41981=DIRECTION('ref_axis',(1.48589474058269E-13,1.,-2.90739654573716E-15)) ;
#41982=DIRECTION('center_axis',(-6.48092690624107E-15,-1.,2.90739654573716E-15)) ;
#41983=DIRECTION('ref_axis',(1.88526971141291E-28,-2.90739654573716E-15,
-1.)) ;
#41984=DIRECTION('center_axis',(1.88526971141291E-28,-2.90739654573716E-15,
-1.)) ;
#41985=DIRECTION('ref_axis',(1.,-6.48092690624108E-15,2.07369595641671E-28)) ;
#41986=DIRECTION('center_axis',(2.1716102378779E-15,-3.66854633798134E-28,
-1.)) ;
#41987=DIRECTION('ref_axis',(0.707106781186543,-0.707106781186552,1.53556032529784E-15)) ;
#41988=DIRECTION('',(2.1716102378779E-15,-3.66854633798134E-28,-1.)) ;
#41989=DIRECTION('center_axis',(-1.66533453692966E-16,-1.,3.83386399937507E-28)) ;
#41990=DIRECTION('ref_axis',(0.707106781186648,-1.17756934401E-16,-0.707106781186447)) ;
#41991=DIRECTION('center_axis',(6.48092690628146E-15,1.,-2.90739654573716E-15)) ;
#41992=DIRECTION('ref_axis',(1.,-6.48092690628146E-15,2.07369595641789E-28)) ;
#41993=DIRECTION('',(1.66533453692966E-16,1.,-3.83386399937507E-28)) ;
#41994=DIRECTION('center_axis',(1.,-6.48092690624107E-15,2.07369595641671E-28)) ;
#41995=DIRECTION('ref_axis',(0.,1.,0.)) ;
#41996=DIRECTION('center_axis',(1.,-1.48589474058269E-13,6.20535494751205E-28)) ;
#41997=DIRECTION('ref_axis',(-1.88526971141292E-28,2.90739654573716E-15,
1.)) ;
#41998=DIRECTION('center_axis',(-6.48092690624107E-15,-1.,2.90739654573716E-15)) ;
#41999=DIRECTION('ref_axis',(-1.,6.48092690624107E-15,-2.07369595641671E-28)) ;
#42000=DIRECTION('center_axis',(8.32667268460789E-17,1.,-3.83780830390118E-28)) ;
#42001=DIRECTION('ref_axis',(-0.707106781186447,5.88784671997906E-17,-0.707106781186648)) ;
#42002=DIRECTION('center_axis',(6.48092690624107E-15,1.,-2.90739654573716E-15)) ;
#42003=DIRECTION('ref_axis',(1.88526971141291E-28,-2.90739654573716E-15,
-1.)) ;
#42004=DIRECTION('',(-8.32667268460789E-17,-1.,3.83780830390118E-28)) ;
#42005=DIRECTION('center_axis',(-1.,3.33066907386739E-16,-2.1716102378779E-15)) ;
#42006=DIRECTION('ref_axis',(-1.30004645649559E-15,0.70710678118655,0.707106781186545)) ;
#42007=DIRECTION('',(-1.,3.33066907386739E-16,-2.1716102378779E-15)) ;
#42008=DIRECTION('',(1.,-3.33066907386739E-16,2.1716102378779E-15)) ;
#42009=DIRECTION('center_axis',(8.32667268460789E-17,1.,-3.83780830390118E-28)) ;
#42010=DIRECTION('ref_axis',(-0.707106781186447,5.88784671997906E-17,-0.707106781186648)) ;
#42011=DIRECTION('center_axis',(-6.48092690624107E-15,-1.,2.90739654573716E-15)) ;
#42012=DIRECTION('ref_axis',(-1.,6.48092690624107E-15,-2.07369595641671E-28)) ;
#42013=DIRECTION('',(-8.32667268460789E-17,-1.,3.83780830390118E-28)) ;
#42014=DIRECTION('center_axis',(1.,-3.33066907386739E-16,2.1716102378779E-15)) ;
#42015=DIRECTION('ref_axis',(-1.77107419409959E-15,-0.707106781186545,0.70710678118655)) ;
#42016=DIRECTION('',(1.,-3.33066907386739E-16,2.1716102378779E-15)) ;
#42017=DIRECTION('center_axis',(-0.81649658092765,0.408248290464166,0.408248290463711)) ;
#42018=DIRECTION('ref_axis',(-0.577350269189702,-0.577350269189929,-0.577350269189247)) ;
#42019=DIRECTION('center_axis',(2.17161023787787E-15,-3.83420712807771E-28,
-1.)) ;
#42020=DIRECTION('ref_axis',(-0.707106781186582,-0.707106781186513,-1.53556032529738E-15)) ;
#42021=DIRECTION('center_axis',(-0.40824829046392,0.408248290464147,-0.816496580927556)) ;
#42022=DIRECTION('ref_axis',(0.577350269189076,-0.577350269189986,-0.577350269189815)) ;
#42023=DIRECTION('center_axis',(1.,-1.66533453692966E-16,2.1716102378779E-15)) ;
#42024=DIRECTION('ref_axis',(1.65331725969831E-15,0.707106781186545,-0.70710678118655)) ;
#42025=DIRECTION('center_axis',(1.,1.35627620245787E-13,-2.05796303467862E-28)) ;
#42026=DIRECTION('ref_axis',(1.8852697114129E-28,-2.90739654573716E-15,
-1.)) ;
#42027=DIRECTION('',(-1.,1.66533453692966E-16,-2.1716102378779E-15)) ;
#42028=DIRECTION('center_axis',(-1.,-1.35627620245787E-13,2.05796303467862E-28)) ;
#42029=DIRECTION('ref_axis',(-1.35627620245787E-13,1.,-2.90739654573716E-15)) ;
#42030=DIRECTION('center_axis',(0.40824829046392,-0.408248290464147,-0.816496580927556)) ;
#42031=DIRECTION('ref_axis',(-0.577350269189834,0.577350269189152,-0.577350269189891)) ;
#42032=DIRECTION('center_axis',(2.17161023787787E-15,-3.83815143260382E-28,
-1.)) ;
#42033=DIRECTION('ref_axis',(-0.707106781186656,0.707106781186439,-1.53556032529808E-15)) ;
#42034=DIRECTION('center_axis',(-0.81649658092765,0.408248290464166,-0.408248290463711)) ;
#42035=DIRECTION('ref_axis',(0.577350269189702,0.577350269189929,-0.577350269189247)) ;
#42036=DIRECTION('center_axis',(-3.33066907386739E-16,-1.,3.66031460022645E-28)) ;
#42037=DIRECTION('ref_axis',(-2.17161023787795E-15,3.66754751528624E-28,
1.)) ;
#42038=DIRECTION('center_axis',(2.1716102378779E-15,-3.83815143260386E-28,
-1.)) ;
#42039=DIRECTION('ref_axis',(1.,-1.66533453692941E-16,2.1716102378779E-15)) ;
#42040=DIRECTION('center_axis',(2.1716102378779E-15,-3.83815143260386E-28,
-1.)) ;
#42041=DIRECTION('ref_axis',(1.,-1.66533453692941E-16,2.1716102378779E-15)) ;
#42042=DIRECTION('center_axis',(2.1716102378779E-15,-3.83815143260386E-28,
-1.)) ;
#42043=DIRECTION('ref_axis',(1.,-1.66533453692941E-16,2.1716102378779E-15)) ;
#42044=DIRECTION('',(-1.66533453692966E-16,-1.,3.83386399937507E-28)) ;
#42045=DIRECTION('',(1.,-1.66533453692587E-16,2.1716102378779E-15)) ;
#42046=DIRECTION('',(8.32667268460789E-17,1.,-3.83780830390118E-28)) ;
#42047=DIRECTION('',(-1.,1.66533453692966E-16,-2.1716102378779E-15)) ;
#42048=DIRECTION('center_axis',(-0.816496580927764,0.408248290464109,0.408248290463541)) ;
#42049=DIRECTION('ref_axis',(-0.577350269189531,-0.577350269189986,-0.57735026918936)) ;
#42050=DIRECTION('center_axis',(1.,1.35627620245787E-13,2.17161023787752E-15)) ;
#42051=DIRECTION('ref_axis',(1.35627620245787E-13,-1.,2.90739654573778E-15)) ;
#42052=DIRECTION('center_axis',(6.48092690624107E-15,1.,-2.90739654573747E-15)) ;
#42053=DIRECTION('ref_axis',(2.17161023787792E-15,-2.90739654573748E-15,
-1.)) ;
#42054=DIRECTION('center_axis',(2.1716102378779E-15,-3.83420712807775E-28,
-1.)) ;
#42055=DIRECTION('ref_axis',(-0.70710678118651,-0.707106781186585,-1.53556032529724E-15)) ;
#42056=DIRECTION('center_axis',(0.40824829046392,-0.408248290464147,-0.816496580927556)) ;
#42057=DIRECTION('ref_axis',(-0.577350269189986,0.577350269189076,-0.577350269189815)) ;
#42058=DIRECTION('center_axis',(-6.48092690624107E-15,-1.,2.90739654573747E-15)) ;
#42059=DIRECTION('ref_axis',(-1.,6.48092690624106E-15,-2.17161023787794E-15)) ;
#42060=DIRECTION('center_axis',(1.,1.35627620245787E-13,2.17161023787752E-15)) ;
#42061=DIRECTION('ref_axis',(2.17161023787791E-15,-2.90739654573749E-15,
-1.)) ;
#42062=DIRECTION('center_axis',(2.1716102378779E-15,-3.83815143260386E-28,
-1.)) ;
#42063=DIRECTION('ref_axis',(-0.707106781186656,0.707106781186439,-1.5355603252981E-15)) ;
#42064=DIRECTION('center_axis',(1.66533453692966E-16,1.,-3.83386399937507E-28)) ;
#42065=DIRECTION('ref_axis',(-0.707106781186596,1.17756934400449E-16,-0.707106781186499)) ;
#42066=DIRECTION('',(1.66533453692966E-16,1.,-3.83386399937507E-28)) ;
#42067=DIRECTION('center_axis',(1.,-1.66533453692966E-16,2.1716102378779E-15)) ;
#42068=DIRECTION('ref_axis',(1.65331725969841E-15,0.707106781186495,-0.7071067811866)) ;
#42069=DIRECTION('center_axis',(1.,1.35627620245787E-13,2.17161023787752E-15)) ;
#42070=DIRECTION('ref_axis',(-1.35627620245787E-13,1.,-2.90739654573778E-15)) ;
#42071=DIRECTION('center_axis',(-1.,1.66533453692587E-16,-2.1716102378779E-15)) ;
#42072=DIRECTION('ref_axis',(1.41780339089726E-15,-0.707106781186499,-0.707106781186596)) ;
#42073=DIRECTION('',(-1.,1.66533453692587E-16,-2.1716102378779E-15)) ;
#42074=DIRECTION('center_axis',(1.,1.35627620245787E-13,2.17161023787752E-15)) ;
#42075=DIRECTION('ref_axis',(2.17161023787792E-15,-2.90739654573749E-15,
-1.)) ;
#42076=DIRECTION('center_axis',(-8.32667268460789E-17,-1.,3.83780830390118E-28)) ;
#42077=DIRECTION('ref_axis',(0.707106781186599,-5.8878467200346E-17,-0.707106781186496)) ;
#42078=DIRECTION('center_axis',(-6.48092690624107E-15,-1.,2.90739654573747E-15)) ;
#42079=DIRECTION('ref_axis',(1.,-6.48092690624106E-15,2.17161023787794E-15)) ;
#42080=DIRECTION('center_axis',(6.48092690624107E-15,1.,-2.90739654573747E-15)) ;
#42081=DIRECTION('ref_axis',(2.17161023787792E-15,-2.90739654573748E-15,
-1.)) ;
#42082=DIRECTION('center_axis',(-0.408248290463939,0.408248290464166,-0.816496580927537)) ;
#42083=DIRECTION('ref_axis',(0.577350269189076,-0.577350269189986,-0.577350269189815)) ;
#42084=DIRECTION('center_axis',(0.408248290463948,-0.816496580927442,-0.408248290464346)) ;
#42085=DIRECTION('ref_axis',(0.577350269189304,0.577350269189986,-0.577350269189588)) ;
#42086=DIRECTION('center_axis',(-2.1716102378779E-15,3.66854633798134E-28,
1.)) ;
#42087=DIRECTION('ref_axis',(0.707106781186452,0.707106781186643,1.53556032529713E-15)) ;
#42088=DIRECTION('center_axis',(1.88526971141291E-28,-2.90739654573716E-15,
-1.)) ;
#42089=DIRECTION('ref_axis',(-1.35627620245787E-13,1.,-2.90739654573716E-15)) ;
#42090=DIRECTION('center_axis',(1.,-1.66533453692587E-16,2.1716102378779E-15)) ;
#42091=DIRECTION('ref_axis',(1.41780339089714E-15,-0.70710678118655,-0.707106781186545)) ;
#42092=DIRECTION('center_axis',(1.,1.35627620245787E-13,-2.05796303467862E-28)) ;
#42093=DIRECTION('ref_axis',(1.35627620245787E-13,-1.,2.90739654573716E-15)) ;
#42094=DIRECTION('',(-1.,1.66533453692587E-16,-2.1716102378779E-15)) ;
#42095=DIRECTION('center_axis',(-1.,-1.35627620245747E-13,2.05796303467745E-28)) ;
#42096=DIRECTION('ref_axis',(1.88526971141291E-28,-2.90739654573716E-15,
-1.)) ;
#42097=DIRECTION('',(1.,-1.66533453692587E-16,2.1716102378779E-15)) ;
#42098=DIRECTION('center_axis',(-1.,6.48092690624107E-15,-2.07369595641671E-28)) ;
#42099=DIRECTION('ref_axis',(0.,-1.,0.)) ;
#42100=DIRECTION('center_axis',(-1.,7.08071943160919E-13,-2.24717289282075E-27)) ;
#42101=DIRECTION('ref_axis',(-1.88526971141296E-28,2.90739654573716E-15,
1.)) ;
#42102=DIRECTION('center_axis',(6.48092690624107E-15,1.,-2.90739654573716E-15)) ;
#42103=DIRECTION('ref_axis',(1.,-6.48092690624107E-15,2.07369595641671E-28)) ;
#42104=DIRECTION('center_axis',(-1.66533453692966E-16,-1.,3.83386399937507E-28)) ;
#42105=DIRECTION('ref_axis',(0.707106781186648,-1.17756934401E-16,-0.707106781186447)) ;
#42106=DIRECTION('center_axis',(-6.48092690624107E-15,-1.,2.90739654573716E-15)) ;
#42107=DIRECTION('ref_axis',(1.88526971141291E-28,-2.90739654573716E-15,
-1.)) ;
#42108=DIRECTION('',(1.66533453692966E-16,1.,-3.83386399937507E-28)) ;
#42109=DIRECTION('center_axis',(1.,-6.48092690624107E-15,2.07369595641671E-28)) ;
#42110=DIRECTION('ref_axis',(0.,1.,0.)) ;
#42111=DIRECTION('center_axis',(1.,-1.48589474058271E-13,-5.59482469102492E-13)) ;
#42112=DIRECTION('ref_axis',(-1.48589474058269E-13,-1.,2.90739654573716E-15)) ;
#42113=DIRECTION('center_axis',(6.48092690624107E-15,1.,-2.90739654573716E-15)) ;
#42114=DIRECTION('ref_axis',(1.88526971141291E-28,-2.90739654573716E-15,
-1.)) ;
#42115=DIRECTION('center_axis',(-1.,6.48092690624107E-15,-2.07369595641671E-28)) ;
#42116=DIRECTION('ref_axis',(0.,-1.,0.)) ;
#42117=DIRECTION('center_axis',(-1.,1.48589474058269E-13,-6.20535494751205E-28)) ;
#42118=DIRECTION('ref_axis',(1.48589474058269E-13,1.,-2.90739654573716E-15)) ;
#42119=DIRECTION('center_axis',(-6.48092690624107E-15,-1.,2.90739654573716E-15)) ;
#42120=DIRECTION('ref_axis',(1.88526971141291E-28,-2.90739654573716E-15,
-1.)) ;
#42121=DIRECTION('center_axis',(1.88526971141291E-28,-2.90739654573716E-15,
-1.)) ;
#42122=DIRECTION('ref_axis',(1.,-6.48092690624108E-15,2.07369595641671E-28)) ;
#42123=DIRECTION('center_axis',(2.1716102378779E-15,-3.66854633798134E-28,
-1.)) ;
#42124=DIRECTION('ref_axis',(0.707106781186543,-0.707106781186552,1.53556032529784E-15)) ;
#42125=DIRECTION('',(2.1716102378779E-15,-3.66854633798134E-28,-1.)) ;
#42126=DIRECTION('center_axis',(-1.66533453692966E-16,-1.,3.83386399937507E-28)) ;
#42127=DIRECTION('ref_axis',(0.707106781186648,-1.17756934401E-16,-0.707106781186447)) ;
#42128=DIRECTION('center_axis',(6.48092690628146E-15,1.,-2.90739654573716E-15)) ;
#42129=DIRECTION('ref_axis',(1.,-6.48092690628146E-15,2.07369595641789E-28)) ;
#42130=DIRECTION('',(1.66533453692966E-16,1.,-3.83386399937507E-28)) ;
#42131=DIRECTION('center_axis',(1.,-6.48092690624107E-15,2.07369595641671E-28)) ;
#42132=DIRECTION('ref_axis',(0.,1.,0.)) ;
#42133=DIRECTION('center_axis',(1.,-1.48589474058269E-13,6.20535494751205E-28)) ;
#42134=DIRECTION('ref_axis',(-1.88526971141292E-28,2.90739654573716E-15,
1.)) ;
#42135=DIRECTION('center_axis',(-6.48092690624107E-15,-1.,2.90739654573716E-15)) ;
#42136=DIRECTION('ref_axis',(-1.,6.48092690624107E-15,-2.07369595641671E-28)) ;
#42137=DIRECTION('center_axis',(8.32667268460789E-17,1.,-3.83780830390118E-28)) ;
#42138=DIRECTION('ref_axis',(-0.707106781186447,5.88784671997906E-17,-0.707106781186648)) ;
#42139=DIRECTION('center_axis',(6.48092690624107E-15,1.,-2.90739654573716E-15)) ;
#42140=DIRECTION('ref_axis',(1.88526971141291E-28,-2.90739654573716E-15,
-1.)) ;
#42141=DIRECTION('',(-8.32667268460789E-17,-1.,3.83780830390118E-28)) ;
#42142=DIRECTION('center_axis',(-1.,3.33066907386739E-16,-2.1716102378779E-15)) ;
#42143=DIRECTION('ref_axis',(-1.30004645649559E-15,0.70710678118655,0.707106781186545)) ;
#42144=DIRECTION('',(-1.,3.33066907386739E-16,-2.1716102378779E-15)) ;
#42145=DIRECTION('',(1.,-3.33066907386739E-16,2.1716102378779E-15)) ;
#42146=DIRECTION('center_axis',(8.32667268460789E-17,1.,-3.83780830390118E-28)) ;
#42147=DIRECTION('ref_axis',(-0.707106781186447,5.88784671997906E-17,-0.707106781186648)) ;
#42148=DIRECTION('center_axis',(-6.48092690624107E-15,-1.,2.90739654573716E-15)) ;
#42149=DIRECTION('ref_axis',(-1.,6.48092690624107E-15,-2.07369595641671E-28)) ;
#42150=DIRECTION('',(-8.32667268460789E-17,-1.,3.83780830390118E-28)) ;
#42151=DIRECTION('center_axis',(1.,-3.33066907386739E-16,2.1716102378779E-15)) ;
#42152=DIRECTION('ref_axis',(-1.77107419409959E-15,-0.707106781186545,0.70710678118655)) ;
#42153=DIRECTION('',(1.,-3.33066907386739E-16,2.1716102378779E-15)) ;
#42154=DIRECTION('center_axis',(-0.81649658092765,0.408248290464166,0.408248290463711)) ;
#42155=DIRECTION('ref_axis',(-0.577350269189702,-0.577350269189929,-0.577350269189247)) ;
#42156=DIRECTION('center_axis',(2.17161023787787E-15,-3.83420712807771E-28,
-1.)) ;
#42157=DIRECTION('ref_axis',(-0.707106781186582,-0.707106781186513,-1.53556032529738E-15)) ;
#42158=DIRECTION('center_axis',(-0.40824829046392,0.408248290464147,-0.816496580927556)) ;
#42159=DIRECTION('ref_axis',(0.577350269189076,-0.577350269189986,-0.577350269189815)) ;
#42160=DIRECTION('center_axis',(1.,-1.66533453692966E-16,2.1716102378779E-15)) ;
#42161=DIRECTION('ref_axis',(1.65331725969831E-15,0.707106781186545,-0.70710678118655)) ;
#42162=DIRECTION('center_axis',(1.,1.35627620245787E-13,-2.05796303467862E-28)) ;
#42163=DIRECTION('ref_axis',(1.8852697114129E-28,-2.90739654573716E-15,
-1.)) ;
#42164=DIRECTION('',(-1.,1.66533453692966E-16,-2.1716102378779E-15)) ;
#42165=DIRECTION('center_axis',(-1.,-1.35627620245787E-13,2.05796303467862E-28)) ;
#42166=DIRECTION('ref_axis',(-1.35627620245787E-13,1.,-2.90739654573716E-15)) ;
#42167=DIRECTION('center_axis',(0.40824829046392,-0.408248290464147,-0.816496580927556)) ;
#42168=DIRECTION('ref_axis',(-0.577350269189834,0.577350269189152,-0.577350269189891)) ;
#42169=DIRECTION('center_axis',(2.17161023787787E-15,-3.83815143260382E-28,
-1.)) ;
#42170=DIRECTION('ref_axis',(-0.707106781186656,0.707106781186439,-1.53556032529808E-15)) ;
#42171=DIRECTION('center_axis',(-0.81649658092765,0.408248290464166,-0.408248290463711)) ;
#42172=DIRECTION('ref_axis',(0.577350269189702,0.577350269189929,-0.577350269189247)) ;
#42173=DIRECTION('center_axis',(-3.33066907386739E-16,-1.,3.66031460022645E-28)) ;
#42174=DIRECTION('ref_axis',(-2.17161023787795E-15,3.66754751528624E-28,
1.)) ;
#42175=DIRECTION('center_axis',(2.1716102378779E-15,-3.83815143260386E-28,
-1.)) ;
#42176=DIRECTION('ref_axis',(1.,-1.66533453692941E-16,2.1716102378779E-15)) ;
#42177=DIRECTION('center_axis',(2.1716102378779E-15,-3.83815143260386E-28,
-1.)) ;
#42178=DIRECTION('ref_axis',(1.,-1.66533453692941E-16,2.1716102378779E-15)) ;
#42179=DIRECTION('center_axis',(2.1716102378779E-15,-3.83815143260386E-28,
-1.)) ;
#42180=DIRECTION('ref_axis',(1.,-1.66533453692941E-16,2.1716102378779E-15)) ;
#42181=DIRECTION('',(-1.66533453692966E-16,-1.,3.83386399937507E-28)) ;
#42182=DIRECTION('',(1.,-1.66533453692587E-16,2.1716102378779E-15)) ;
#42183=DIRECTION('',(8.32667268460789E-17,1.,-3.83780830390118E-28)) ;
#42184=DIRECTION('',(-1.,1.66533453692966E-16,-2.1716102378779E-15)) ;
#42185=DIRECTION('center_axis',(-0.816496580927764,0.408248290464109,0.408248290463541)) ;
#42186=DIRECTION('ref_axis',(-0.577350269189531,-0.577350269189986,-0.57735026918936)) ;
#42187=DIRECTION('center_axis',(1.,1.35627620245787E-13,2.17161023787752E-15)) ;
#42188=DIRECTION('ref_axis',(1.35627620245787E-13,-1.,2.90739654573778E-15)) ;
#42189=DIRECTION('center_axis',(6.48092690624107E-15,1.,-2.90739654573747E-15)) ;
#42190=DIRECTION('ref_axis',(2.17161023787792E-15,-2.90739654573748E-15,
-1.)) ;
#42191=DIRECTION('center_axis',(2.1716102378779E-15,-3.83420712807775E-28,
-1.)) ;
#42192=DIRECTION('ref_axis',(-0.70710678118651,-0.707106781186585,-1.53556032529724E-15)) ;
#42193=DIRECTION('center_axis',(0.40824829046392,-0.408248290464147,-0.816496580927556)) ;
#42194=DIRECTION('ref_axis',(-0.577350269189986,0.577350269189076,-0.577350269189815)) ;
#42195=DIRECTION('center_axis',(-6.48092690624107E-15,-1.,2.90739654573747E-15)) ;
#42196=DIRECTION('ref_axis',(-1.,6.48092690624106E-15,-2.17161023787794E-15)) ;
#42197=DIRECTION('center_axis',(1.,1.35627620245787E-13,2.17161023787752E-15)) ;
#42198=DIRECTION('ref_axis',(2.17161023787791E-15,-2.90739654573749E-15,
-1.)) ;
#42199=DIRECTION('center_axis',(2.1716102378779E-15,-3.83815143260386E-28,
-1.)) ;
#42200=DIRECTION('ref_axis',(-0.707106781186656,0.707106781186439,-1.5355603252981E-15)) ;
#42201=DIRECTION('center_axis',(1.66533453692966E-16,1.,-3.83386399937507E-28)) ;
#42202=DIRECTION('ref_axis',(-0.707106781186596,1.17756934400449E-16,-0.707106781186499)) ;
#42203=DIRECTION('',(1.66533453692966E-16,1.,-3.83386399937507E-28)) ;
#42204=DIRECTION('center_axis',(1.,-1.66533453692966E-16,2.1716102378779E-15)) ;
#42205=DIRECTION('ref_axis',(1.65331725969841E-15,0.707106781186495,-0.7071067811866)) ;
#42206=DIRECTION('center_axis',(1.,1.35627620245787E-13,2.17161023787752E-15)) ;
#42207=DIRECTION('ref_axis',(-1.35627620245787E-13,1.,-2.90739654573778E-15)) ;
#42208=DIRECTION('center_axis',(-1.,1.66533453692587E-16,-2.1716102378779E-15)) ;
#42209=DIRECTION('ref_axis',(1.41780339089726E-15,-0.707106781186499,-0.707106781186596)) ;
#42210=DIRECTION('',(-1.,1.66533453692587E-16,-2.1716102378779E-15)) ;
#42211=DIRECTION('center_axis',(1.,1.35627620245787E-13,2.17161023787752E-15)) ;
#42212=DIRECTION('ref_axis',(2.17161023787792E-15,-2.90739654573749E-15,
-1.)) ;
#42213=DIRECTION('center_axis',(-8.32667268460789E-17,-1.,3.83780830390118E-28)) ;
#42214=DIRECTION('ref_axis',(0.707106781186599,-5.8878467200346E-17,-0.707106781186496)) ;
#42215=DIRECTION('center_axis',(-6.48092690624107E-15,-1.,2.90739654573747E-15)) ;
#42216=DIRECTION('ref_axis',(1.,-6.48092690624106E-15,2.17161023787794E-15)) ;
#42217=DIRECTION('center_axis',(6.48092690624107E-15,1.,-2.90739654573747E-15)) ;
#42218=DIRECTION('ref_axis',(2.17161023787792E-15,-2.90739654573748E-15,
-1.)) ;
#42219=DIRECTION('center_axis',(-0.408248290463939,0.408248290464166,-0.816496580927537)) ;
#42220=DIRECTION('ref_axis',(0.577350269189076,-0.577350269189986,-0.577350269189815)) ;
#42221=DIRECTION('center_axis',(0.408248290463948,-0.816496580927442,-0.408248290464346)) ;
#42222=DIRECTION('ref_axis',(0.577350269189304,0.577350269189986,-0.577350269189588)) ;
#42223=DIRECTION('center_axis',(-2.1716102378779E-15,3.66854633798134E-28,
1.)) ;
#42224=DIRECTION('ref_axis',(0.707106781186452,0.707106781186643,1.53556032529713E-15)) ;
#42225=DIRECTION('center_axis',(1.88526971141291E-28,-2.90739654573716E-15,
-1.)) ;
#42226=DIRECTION('ref_axis',(-1.35627620245787E-13,1.,-2.90739654573716E-15)) ;
#42227=DIRECTION('center_axis',(1.,-1.66533453692587E-16,2.1716102378779E-15)) ;
#42228=DIRECTION('ref_axis',(1.41780339089714E-15,-0.70710678118655,-0.707106781186545)) ;
#42229=DIRECTION('center_axis',(1.,1.35627620245787E-13,-2.05796303467862E-28)) ;
#42230=DIRECTION('ref_axis',(1.35627620245787E-13,-1.,2.90739654573716E-15)) ;
#42231=DIRECTION('',(-1.,1.66533453692587E-16,-2.1716102378779E-15)) ;
#42232=DIRECTION('center_axis',(-1.,-1.35627620245747E-13,2.05796303467745E-28)) ;
#42233=DIRECTION('ref_axis',(1.88526971141291E-28,-2.90739654573716E-15,
-1.)) ;
#42234=DIRECTION('',(1.,-1.66533453692587E-16,2.1716102378779E-15)) ;
#42235=DIRECTION('center_axis',(-1.,6.48092690624107E-15,-2.07369595641671E-28)) ;
#42236=DIRECTION('ref_axis',(0.,-1.,0.)) ;
#42237=DIRECTION('center_axis',(-1.,7.08071943160919E-13,-2.24717289282075E-27)) ;
#42238=DIRECTION('ref_axis',(-1.88526971141296E-28,2.90739654573716E-15,
1.)) ;
#42239=DIRECTION('center_axis',(6.48092690624107E-15,1.,-2.90739654573716E-15)) ;
#42240=DIRECTION('ref_axis',(1.,-6.48092690624107E-15,2.07369595641671E-28)) ;
#42241=DIRECTION('center_axis',(-1.66533453692966E-16,-1.,3.83386399937507E-28)) ;
#42242=DIRECTION('ref_axis',(0.707106781186648,-1.17756934401E-16,-0.707106781186447)) ;
#42243=DIRECTION('center_axis',(-6.48092690624107E-15,-1.,2.90739654573716E-15)) ;
#42244=DIRECTION('ref_axis',(1.88526971141291E-28,-2.90739654573716E-15,
-1.)) ;
#42245=DIRECTION('',(1.66533453692966E-16,1.,-3.83386399937507E-28)) ;
#42246=DIRECTION('center_axis',(1.,-6.48092690624107E-15,2.07369595641671E-28)) ;
#42247=DIRECTION('ref_axis',(0.,1.,0.)) ;
#42248=DIRECTION('center_axis',(1.,-1.48589474058271E-13,-5.59482469102492E-13)) ;
#42249=DIRECTION('ref_axis',(-1.48589474058269E-13,-1.,2.90739654573716E-15)) ;
#42250=DIRECTION('center_axis',(6.48092690624107E-15,1.,-2.90739654573716E-15)) ;
#42251=DIRECTION('ref_axis',(1.88526971141291E-28,-2.90739654573716E-15,
-1.)) ;
#42252=DIRECTION('center_axis',(-1.,6.48092690624107E-15,-2.07369595641671E-28)) ;
#42253=DIRECTION('ref_axis',(0.,-1.,0.)) ;
#42254=DIRECTION('center_axis',(-1.,1.48589474058269E-13,-6.20535494751205E-28)) ;
#42255=DIRECTION('ref_axis',(1.48589474058269E-13,1.,-2.90739654573716E-15)) ;
#42256=DIRECTION('center_axis',(-6.48092690624107E-15,-1.,2.90739654573716E-15)) ;
#42257=DIRECTION('ref_axis',(1.88526971141291E-28,-2.90739654573716E-15,
-1.)) ;
#42258=DIRECTION('center_axis',(1.88526971141291E-28,-2.90739654573716E-15,
-1.)) ;
#42259=DIRECTION('ref_axis',(1.,-6.48092690624108E-15,2.07369595641671E-28)) ;
#42260=DIRECTION('center_axis',(2.1716102378779E-15,-3.66854633798134E-28,
-1.)) ;
#42261=DIRECTION('ref_axis',(0.707106781186543,-0.707106781186552,1.53556032529784E-15)) ;
#42262=DIRECTION('',(2.1716102378779E-15,-3.66854633798134E-28,-1.)) ;
#42263=DIRECTION('center_axis',(-1.66533453692966E-16,-1.,3.83386399937507E-28)) ;
#42264=DIRECTION('ref_axis',(0.707106781186648,-1.17756934401E-16,-0.707106781186447)) ;
#42265=DIRECTION('center_axis',(6.48092690628146E-15,1.,-2.90739654573716E-15)) ;
#42266=DIRECTION('ref_axis',(1.,-6.48092690628146E-15,2.07369595641789E-28)) ;
#42267=DIRECTION('',(1.66533453692966E-16,1.,-3.83386399937507E-28)) ;
#42268=DIRECTION('center_axis',(1.,-6.48092690624107E-15,2.07369595641671E-28)) ;
#42269=DIRECTION('ref_axis',(0.,1.,0.)) ;
#42270=DIRECTION('center_axis',(1.,-1.48589474058269E-13,6.20535494751205E-28)) ;
#42271=DIRECTION('ref_axis',(-1.88526971141292E-28,2.90739654573716E-15,
1.)) ;
#42272=DIRECTION('center_axis',(-6.48092690624107E-15,-1.,2.90739654573716E-15)) ;
#42273=DIRECTION('ref_axis',(-1.,6.48092690624107E-15,-2.07369595641671E-28)) ;
#42274=DIRECTION('center_axis',(8.32667268460789E-17,1.,-3.83780830390118E-28)) ;
#42275=DIRECTION('ref_axis',(-0.707106781186447,5.88784671997906E-17,-0.707106781186648)) ;
#42276=DIRECTION('center_axis',(6.48092690624107E-15,1.,-2.90739654573716E-15)) ;
#42277=DIRECTION('ref_axis',(1.88526971141291E-28,-2.90739654573716E-15,
-1.)) ;
#42278=DIRECTION('',(-8.32667268460789E-17,-1.,3.83780830390118E-28)) ;
#42279=DIRECTION('center_axis',(-1.,3.33066907386739E-16,-2.1716102378779E-15)) ;
#42280=DIRECTION('ref_axis',(-1.30004645649559E-15,0.70710678118655,0.707106781186545)) ;
#42281=DIRECTION('',(-1.,3.33066907386739E-16,-2.1716102378779E-15)) ;
#42282=DIRECTION('',(1.,-3.33066907386739E-16,2.1716102378779E-15)) ;
#42283=DIRECTION('center_axis',(8.32667268460789E-17,1.,-3.83780830390118E-28)) ;
#42284=DIRECTION('ref_axis',(-0.707106781186447,5.88784671997906E-17,-0.707106781186648)) ;
#42285=DIRECTION('center_axis',(-6.48092690624107E-15,-1.,2.90739654573716E-15)) ;
#42286=DIRECTION('ref_axis',(-1.,6.48092690624107E-15,-2.07369595641671E-28)) ;
#42287=DIRECTION('',(-8.32667268460789E-17,-1.,3.83780830390118E-28)) ;
#42288=DIRECTION('center_axis',(1.,-3.33066907386739E-16,2.1716102378779E-15)) ;
#42289=DIRECTION('ref_axis',(-1.77107419409959E-15,-0.707106781186545,0.70710678118655)) ;
#42290=DIRECTION('',(1.,-3.33066907386739E-16,2.1716102378779E-15)) ;
#42291=DIRECTION('center_axis',(-0.81649658092765,0.408248290464166,0.408248290463711)) ;
#42292=DIRECTION('ref_axis',(-0.577350269189702,-0.577350269189929,-0.577350269189247)) ;
#42293=DIRECTION('center_axis',(2.17161023787787E-15,-3.83420712807771E-28,
-1.)) ;
#42294=DIRECTION('ref_axis',(-0.707106781186582,-0.707106781186513,-1.53556032529738E-15)) ;
#42295=DIRECTION('center_axis',(-0.40824829046392,0.408248290464147,-0.816496580927556)) ;
#42296=DIRECTION('ref_axis',(0.577350269189076,-0.577350269189986,-0.577350269189815)) ;
#42297=DIRECTION('center_axis',(1.,-1.66533453692966E-16,2.1716102378779E-15)) ;
#42298=DIRECTION('ref_axis',(1.65331725969831E-15,0.707106781186545,-0.70710678118655)) ;
#42299=DIRECTION('center_axis',(1.,1.35627620245787E-13,-2.05796303467862E-28)) ;
#42300=DIRECTION('ref_axis',(1.8852697114129E-28,-2.90739654573716E-15,
-1.)) ;
#42301=DIRECTION('',(-1.,1.66533453692966E-16,-2.1716102378779E-15)) ;
#42302=DIRECTION('center_axis',(-1.,-1.35627620245787E-13,2.05796303467862E-28)) ;
#42303=DIRECTION('ref_axis',(-1.35627620245787E-13,1.,-2.90739654573716E-15)) ;
#42304=DIRECTION('center_axis',(0.40824829046392,-0.408248290464147,-0.816496580927556)) ;
#42305=DIRECTION('ref_axis',(-0.577350269189834,0.577350269189152,-0.577350269189891)) ;
#42306=DIRECTION('center_axis',(2.17161023787787E-15,-3.83815143260382E-28,
-1.)) ;
#42307=DIRECTION('ref_axis',(-0.707106781186656,0.707106781186439,-1.53556032529808E-15)) ;
#42308=DIRECTION('center_axis',(-0.81649658092765,0.408248290464166,-0.408248290463711)) ;
#42309=DIRECTION('ref_axis',(0.577350269189702,0.577350269189929,-0.577350269189247)) ;
#42310=DIRECTION('center_axis',(-3.33066907386739E-16,-1.,3.66031460022645E-28)) ;
#42311=DIRECTION('ref_axis',(-2.17161023787795E-15,3.66754751528624E-28,
1.)) ;
#42312=DIRECTION('center_axis',(2.1716102378779E-15,-3.83815143260386E-28,
-1.)) ;
#42313=DIRECTION('ref_axis',(1.,-1.66533453692941E-16,2.1716102378779E-15)) ;
#42314=DIRECTION('center_axis',(2.1716102378779E-15,-3.83815143260386E-28,
-1.)) ;
#42315=DIRECTION('ref_axis',(1.,-1.66533453692941E-16,2.1716102378779E-15)) ;
#42316=DIRECTION('center_axis',(2.1716102378779E-15,-3.83815143260386E-28,
-1.)) ;
#42317=DIRECTION('ref_axis',(1.,-1.66533453692941E-16,2.1716102378779E-15)) ;
#42318=DIRECTION('',(-1.66533453692966E-16,-1.,3.83386399937507E-28)) ;
#42319=DIRECTION('',(1.,-1.66533453692587E-16,2.1716102378779E-15)) ;
#42320=DIRECTION('',(8.32667268460789E-17,1.,-3.83780830390118E-28)) ;
#42321=DIRECTION('',(-1.,1.66533453692966E-16,-2.1716102378779E-15)) ;
#42322=DIRECTION('center_axis',(-0.816496580927764,0.408248290464109,0.408248290463541)) ;
#42323=DIRECTION('ref_axis',(-0.577350269189531,-0.577350269189986,-0.57735026918936)) ;
#42324=DIRECTION('center_axis',(1.,1.35627620245787E-13,2.17161023787752E-15)) ;
#42325=DIRECTION('ref_axis',(1.35627620245787E-13,-1.,2.90739654573778E-15)) ;
#42326=DIRECTION('center_axis',(6.48092690624107E-15,1.,-2.90739654573747E-15)) ;
#42327=DIRECTION('ref_axis',(2.17161023787792E-15,-2.90739654573748E-15,
-1.)) ;
#42328=DIRECTION('center_axis',(2.1716102378779E-15,-3.83420712807775E-28,
-1.)) ;
#42329=DIRECTION('ref_axis',(-0.70710678118651,-0.707106781186585,-1.53556032529724E-15)) ;
#42330=DIRECTION('center_axis',(0.40824829046392,-0.408248290464147,-0.816496580927556)) ;
#42331=DIRECTION('ref_axis',(-0.577350269189986,0.577350269189076,-0.577350269189815)) ;
#42332=DIRECTION('center_axis',(-6.48092690624107E-15,-1.,2.90739654573747E-15)) ;
#42333=DIRECTION('ref_axis',(-1.,6.48092690624106E-15,-2.17161023787794E-15)) ;
#42334=DIRECTION('center_axis',(1.,1.35627620245787E-13,2.17161023787752E-15)) ;
#42335=DIRECTION('ref_axis',(2.17161023787791E-15,-2.90739654573749E-15,
-1.)) ;
#42336=DIRECTION('center_axis',(2.1716102378779E-15,-3.83815143260386E-28,
-1.)) ;
#42337=DIRECTION('ref_axis',(-0.707106781186656,0.707106781186439,-1.5355603252981E-15)) ;
#42338=DIRECTION('center_axis',(1.66533453692966E-16,1.,-3.83386399937507E-28)) ;
#42339=DIRECTION('ref_axis',(-0.707106781186596,1.17756934400449E-16,-0.707106781186499)) ;
#42340=DIRECTION('',(1.66533453692966E-16,1.,-3.83386399937507E-28)) ;
#42341=DIRECTION('center_axis',(1.,-1.66533453692966E-16,2.1716102378779E-15)) ;
#42342=DIRECTION('ref_axis',(1.65331725969841E-15,0.707106781186495,-0.7071067811866)) ;
#42343=DIRECTION('center_axis',(1.,1.35627620245787E-13,2.17161023787752E-15)) ;
#42344=DIRECTION('ref_axis',(-1.35627620245787E-13,1.,-2.90739654573778E-15)) ;
#42345=DIRECTION('center_axis',(-1.,1.66533453692587E-16,-2.1716102378779E-15)) ;
#42346=DIRECTION('ref_axis',(1.41780339089726E-15,-0.707106781186499,-0.707106781186596)) ;
#42347=DIRECTION('',(-1.,1.66533453692587E-16,-2.1716102378779E-15)) ;
#42348=DIRECTION('center_axis',(1.,1.35627620245787E-13,2.17161023787752E-15)) ;
#42349=DIRECTION('ref_axis',(2.17161023787792E-15,-2.90739654573749E-15,
-1.)) ;
#42350=DIRECTION('center_axis',(-8.32667268460789E-17,-1.,3.83780830390118E-28)) ;
#42351=DIRECTION('ref_axis',(0.707106781186599,-5.8878467200346E-17,-0.707106781186496)) ;
#42352=DIRECTION('center_axis',(-6.48092690624107E-15,-1.,2.90739654573747E-15)) ;
#42353=DIRECTION('ref_axis',(1.,-6.48092690624106E-15,2.17161023787794E-15)) ;
#42354=DIRECTION('center_axis',(6.48092690624107E-15,1.,-2.90739654573747E-15)) ;
#42355=DIRECTION('ref_axis',(2.17161023787792E-15,-2.90739654573748E-15,
-1.)) ;
#42356=DIRECTION('center_axis',(-0.408248290463939,0.408248290464166,-0.816496580927537)) ;
#42357=DIRECTION('ref_axis',(0.577350269189076,-0.577350269189986,-0.577350269189815)) ;
#42358=DIRECTION('center_axis',(0.408248290463948,-0.816496580927442,-0.408248290464346)) ;
#42359=DIRECTION('ref_axis',(0.577350269189304,0.577350269189986,-0.577350269189588)) ;
#42360=DIRECTION('center_axis',(-2.1716102378779E-15,3.66854633798134E-28,
1.)) ;
#42361=DIRECTION('ref_axis',(0.707106781186452,0.707106781186643,1.53556032529713E-15)) ;
#42362=DIRECTION('center_axis',(1.88526971141291E-28,-2.90739654573716E-15,
-1.)) ;
#42363=DIRECTION('ref_axis',(-1.35627620245787E-13,1.,-2.90739654573716E-15)) ;
#42364=DIRECTION('center_axis',(1.,-1.66533453692587E-16,2.1716102378779E-15)) ;
#42365=DIRECTION('ref_axis',(1.41780339089714E-15,-0.70710678118655,-0.707106781186545)) ;
#42366=DIRECTION('center_axis',(1.,1.35627620245787E-13,-2.05796303467862E-28)) ;
#42367=DIRECTION('ref_axis',(1.35627620245787E-13,-1.,2.90739654573716E-15)) ;
#42368=DIRECTION('',(-1.,1.66533453692587E-16,-2.1716102378779E-15)) ;
#42369=DIRECTION('center_axis',(-1.,-1.35627620245747E-13,2.05796303467745E-28)) ;
#42370=DIRECTION('ref_axis',(1.88526971141291E-28,-2.90739654573716E-15,
-1.)) ;
#42371=DIRECTION('',(1.,-1.66533453692587E-16,2.1716102378779E-15)) ;
#42372=DIRECTION('center_axis',(-1.,6.48092690624107E-15,-2.07369595641671E-28)) ;
#42373=DIRECTION('ref_axis',(0.,-1.,0.)) ;
#42374=DIRECTION('center_axis',(-1.,7.08071943160919E-13,-2.24717289282075E-27)) ;
#42375=DIRECTION('ref_axis',(-1.88526971141296E-28,2.90739654573716E-15,
1.)) ;
#42376=DIRECTION('center_axis',(6.48092690624107E-15,1.,-2.90739654573716E-15)) ;
#42377=DIRECTION('ref_axis',(1.,-6.48092690624107E-15,2.07369595641671E-28)) ;
#42378=DIRECTION('center_axis',(-1.66533453692966E-16,-1.,3.83386399937507E-28)) ;
#42379=DIRECTION('ref_axis',(0.707106781186648,-1.17756934401E-16,-0.707106781186447)) ;
#42380=DIRECTION('center_axis',(-6.48092690624107E-15,-1.,2.90739654573716E-15)) ;
#42381=DIRECTION('ref_axis',(1.88526971141291E-28,-2.90739654573716E-15,
-1.)) ;
#42382=DIRECTION('',(1.66533453692966E-16,1.,-3.83386399937507E-28)) ;
#42383=DIRECTION('center_axis',(1.,-6.48092690624107E-15,2.07369595641671E-28)) ;
#42384=DIRECTION('ref_axis',(0.,1.,0.)) ;
#42385=DIRECTION('center_axis',(1.,-1.48589474058271E-13,-5.59482469102492E-13)) ;
#42386=DIRECTION('ref_axis',(-1.48589474058269E-13,-1.,2.90739654573716E-15)) ;
#42387=DIRECTION('center_axis',(6.48092690624107E-15,1.,-2.90739654573716E-15)) ;
#42388=DIRECTION('ref_axis',(1.88526971141291E-28,-2.90739654573716E-15,
-1.)) ;
#42389=DIRECTION('center_axis',(-1.,6.48092690624107E-15,-2.07369595641671E-28)) ;
#42390=DIRECTION('ref_axis',(0.,-1.,0.)) ;
#42391=DIRECTION('center_axis',(-1.,1.48589474058269E-13,-6.20535494751205E-28)) ;
#42392=DIRECTION('ref_axis',(1.48589474058269E-13,1.,-2.90739654573716E-15)) ;
#42393=DIRECTION('center_axis',(-6.48092690624107E-15,-1.,2.90739654573716E-15)) ;
#42394=DIRECTION('ref_axis',(1.88526971141291E-28,-2.90739654573716E-15,
-1.)) ;
#42395=DIRECTION('center_axis',(1.88526971141291E-28,-2.90739654573716E-15,
-1.)) ;
#42396=DIRECTION('ref_axis',(1.,-6.48092690624108E-15,2.07369595641671E-28)) ;
#42397=DIRECTION('center_axis',(2.1716102378779E-15,-3.66854633798134E-28,
-1.)) ;
#42398=DIRECTION('ref_axis',(0.707106781186543,-0.707106781186552,1.53556032529784E-15)) ;
#42399=DIRECTION('',(2.1716102378779E-15,-3.66854633798134E-28,-1.)) ;
#42400=DIRECTION('center_axis',(-1.66533453692966E-16,-1.,3.83386399937507E-28)) ;
#42401=DIRECTION('ref_axis',(0.707106781186648,-1.17756934401E-16,-0.707106781186447)) ;
#42402=DIRECTION('center_axis',(6.48092690628146E-15,1.,-2.90739654573716E-15)) ;
#42403=DIRECTION('ref_axis',(1.,-6.48092690628146E-15,2.07369595641789E-28)) ;
#42404=DIRECTION('',(1.66533453692966E-16,1.,-3.83386399937507E-28)) ;
#42405=DIRECTION('center_axis',(1.,-6.48092690624107E-15,2.07369595641671E-28)) ;
#42406=DIRECTION('ref_axis',(0.,1.,0.)) ;
#42407=DIRECTION('center_axis',(1.,-1.48589474058269E-13,6.20535494751205E-28)) ;
#42408=DIRECTION('ref_axis',(-1.88526971141292E-28,2.90739654573716E-15,
1.)) ;
#42409=DIRECTION('center_axis',(-6.48092690624107E-15,-1.,2.90739654573716E-15)) ;
#42410=DIRECTION('ref_axis',(-1.,6.48092690624107E-15,-2.07369595641671E-28)) ;
#42411=DIRECTION('center_axis',(8.32667268460789E-17,1.,-3.83780830390118E-28)) ;
#42412=DIRECTION('ref_axis',(-0.707106781186447,5.88784671997906E-17,-0.707106781186648)) ;
#42413=DIRECTION('center_axis',(6.48092690624107E-15,1.,-2.90739654573716E-15)) ;
#42414=DIRECTION('ref_axis',(1.88526971141291E-28,-2.90739654573716E-15,
-1.)) ;
#42415=DIRECTION('',(-8.32667268460789E-17,-1.,3.83780830390118E-28)) ;
#42416=DIRECTION('center_axis',(-1.,3.33066907386739E-16,-2.1716102378779E-15)) ;
#42417=DIRECTION('ref_axis',(-1.30004645649559E-15,0.70710678118655,0.707106781186545)) ;
#42418=DIRECTION('',(-1.,3.33066907386739E-16,-2.1716102378779E-15)) ;
#42419=DIRECTION('',(1.,-3.33066907386739E-16,2.1716102378779E-15)) ;
#42420=DIRECTION('center_axis',(8.32667268460789E-17,1.,-3.83780830390118E-28)) ;
#42421=DIRECTION('ref_axis',(-0.707106781186447,5.88784671997906E-17,-0.707106781186648)) ;
#42422=DIRECTION('center_axis',(-6.48092690624107E-15,-1.,2.90739654573716E-15)) ;
#42423=DIRECTION('ref_axis',(-1.,6.48092690624107E-15,-2.07369595641671E-28)) ;
#42424=DIRECTION('',(-8.32667268460789E-17,-1.,3.83780830390118E-28)) ;
#42425=DIRECTION('center_axis',(1.,-3.33066907386739E-16,2.1716102378779E-15)) ;
#42426=DIRECTION('ref_axis',(-1.77107419409959E-15,-0.707106781186545,0.70710678118655)) ;
#42427=DIRECTION('',(1.,-3.33066907386739E-16,2.1716102378779E-15)) ;
#42428=DIRECTION('center_axis',(-0.81649658092765,0.408248290464166,0.408248290463711)) ;
#42429=DIRECTION('ref_axis',(-0.577350269189702,-0.577350269189929,-0.577350269189247)) ;
#42430=DIRECTION('center_axis',(2.17161023787787E-15,-3.83420712807771E-28,
-1.)) ;
#42431=DIRECTION('ref_axis',(-0.707106781186582,-0.707106781186513,-1.53556032529738E-15)) ;
#42432=DIRECTION('center_axis',(-0.40824829046392,0.408248290464147,-0.816496580927556)) ;
#42433=DIRECTION('ref_axis',(0.577350269189076,-0.577350269189986,-0.577350269189815)) ;
#42434=DIRECTION('center_axis',(1.,-1.66533453692966E-16,2.1716102378779E-15)) ;
#42435=DIRECTION('ref_axis',(1.65331725969831E-15,0.707106781186545,-0.70710678118655)) ;
#42436=DIRECTION('center_axis',(1.,1.35627620245787E-13,-2.05796303467862E-28)) ;
#42437=DIRECTION('ref_axis',(1.8852697114129E-28,-2.90739654573716E-15,
-1.)) ;
#42438=DIRECTION('',(-1.,1.66533453692966E-16,-2.1716102378779E-15)) ;
#42439=DIRECTION('center_axis',(-1.,-1.35627620245787E-13,2.05796303467862E-28)) ;
#42440=DIRECTION('ref_axis',(-1.35627620245787E-13,1.,-2.90739654573716E-15)) ;
#42441=DIRECTION('center_axis',(0.40824829046392,-0.408248290464147,-0.816496580927556)) ;
#42442=DIRECTION('ref_axis',(-0.577350269189834,0.577350269189152,-0.577350269189891)) ;
#42443=DIRECTION('center_axis',(2.17161023787787E-15,-3.83815143260382E-28,
-1.)) ;
#42444=DIRECTION('ref_axis',(-0.707106781186656,0.707106781186439,-1.53556032529808E-15)) ;
#42445=DIRECTION('center_axis',(-0.81649658092765,0.408248290464166,-0.408248290463711)) ;
#42446=DIRECTION('ref_axis',(0.577350269189702,0.577350269189929,-0.577350269189247)) ;
#42447=DIRECTION('center_axis',(-3.33066907386739E-16,-1.,3.66031460022645E-28)) ;
#42448=DIRECTION('ref_axis',(-2.17161023787795E-15,3.66754751528624E-28,
1.)) ;
#42449=DIRECTION('center_axis',(2.1716102378779E-15,-3.83815143260386E-28,
-1.)) ;
#42450=DIRECTION('ref_axis',(1.,-1.66533453692941E-16,2.1716102378779E-15)) ;
#42451=DIRECTION('center_axis',(2.1716102378779E-15,-3.83815143260386E-28,
-1.)) ;
#42452=DIRECTION('ref_axis',(1.,-1.66533453692941E-16,2.1716102378779E-15)) ;
#42453=DIRECTION('center_axis',(2.1716102378779E-15,-3.83815143260386E-28,
-1.)) ;
#42454=DIRECTION('ref_axis',(1.,-1.66533453692941E-16,2.1716102378779E-15)) ;
#42455=DIRECTION('',(-1.66533453692966E-16,-1.,3.83386399937507E-28)) ;
#42456=DIRECTION('',(1.,-1.66533453692587E-16,2.1716102378779E-15)) ;
#42457=DIRECTION('',(8.32667268460789E-17,1.,-3.83780830390118E-28)) ;
#42458=DIRECTION('',(-1.,1.66533453692966E-16,-2.1716102378779E-15)) ;
#42459=DIRECTION('center_axis',(-0.816496580927764,0.408248290464109,0.408248290463541)) ;
#42460=DIRECTION('ref_axis',(-0.577350269189531,-0.577350269189986,-0.57735026918936)) ;
#42461=DIRECTION('center_axis',(1.,1.35627620245787E-13,2.17161023787752E-15)) ;
#42462=DIRECTION('ref_axis',(1.35627620245787E-13,-1.,2.90739654573778E-15)) ;
#42463=DIRECTION('center_axis',(6.48092690624107E-15,1.,-2.90739654573747E-15)) ;
#42464=DIRECTION('ref_axis',(2.17161023787792E-15,-2.90739654573748E-15,
-1.)) ;
#42465=DIRECTION('center_axis',(2.1716102378779E-15,-3.83420712807775E-28,
-1.)) ;
#42466=DIRECTION('ref_axis',(-0.70710678118651,-0.707106781186585,-1.53556032529724E-15)) ;
#42467=DIRECTION('center_axis',(0.40824829046392,-0.408248290464147,-0.816496580927556)) ;
#42468=DIRECTION('ref_axis',(-0.577350269189986,0.577350269189076,-0.577350269189815)) ;
#42469=DIRECTION('center_axis',(-6.48092690624107E-15,-1.,2.90739654573747E-15)) ;
#42470=DIRECTION('ref_axis',(-1.,6.48092690624106E-15,-2.17161023787794E-15)) ;
#42471=DIRECTION('center_axis',(1.,1.35627620245787E-13,2.17161023787752E-15)) ;
#42472=DIRECTION('ref_axis',(2.17161023787791E-15,-2.90739654573749E-15,
-1.)) ;
#42473=DIRECTION('center_axis',(2.1716102378779E-15,-3.83815143260386E-28,
-1.)) ;
#42474=DIRECTION('ref_axis',(-0.707106781186656,0.707106781186439,-1.5355603252981E-15)) ;
#42475=DIRECTION('center_axis',(1.66533453692966E-16,1.,-3.83386399937507E-28)) ;
#42476=DIRECTION('ref_axis',(-0.707106781186596,1.17756934400449E-16,-0.707106781186499)) ;
#42477=DIRECTION('',(1.66533453692966E-16,1.,-3.83386399937507E-28)) ;
#42478=DIRECTION('center_axis',(1.,-1.66533453692966E-16,2.1716102378779E-15)) ;
#42479=DIRECTION('ref_axis',(1.65331725969841E-15,0.707106781186495,-0.7071067811866)) ;
#42480=DIRECTION('center_axis',(1.,1.35627620245787E-13,2.17161023787752E-15)) ;
#42481=DIRECTION('ref_axis',(-1.35627620245787E-13,1.,-2.90739654573778E-15)) ;
#42482=DIRECTION('center_axis',(-1.,1.66533453692587E-16,-2.1716102378779E-15)) ;
#42483=DIRECTION('ref_axis',(1.41780339089726E-15,-0.707106781186499,-0.707106781186596)) ;
#42484=DIRECTION('',(-1.,1.66533453692587E-16,-2.1716102378779E-15)) ;
#42485=DIRECTION('center_axis',(1.,1.35627620245787E-13,2.17161023787752E-15)) ;
#42486=DIRECTION('ref_axis',(2.17161023787792E-15,-2.90739654573749E-15,
-1.)) ;
#42487=DIRECTION('center_axis',(-8.32667268460789E-17,-1.,3.83780830390118E-28)) ;
#42488=DIRECTION('ref_axis',(0.707106781186599,-5.8878467200346E-17,-0.707106781186496)) ;
#42489=DIRECTION('center_axis',(-6.48092690624107E-15,-1.,2.90739654573747E-15)) ;
#42490=DIRECTION('ref_axis',(1.,-6.48092690624106E-15,2.17161023787794E-15)) ;
#42491=DIRECTION('center_axis',(6.48092690624107E-15,1.,-2.90739654573747E-15)) ;
#42492=DIRECTION('ref_axis',(2.17161023787792E-15,-2.90739654573748E-15,
-1.)) ;
#42493=DIRECTION('center_axis',(-0.408248290463939,0.408248290464166,-0.816496580927537)) ;
#42494=DIRECTION('ref_axis',(0.577350269189076,-0.577350269189986,-0.577350269189815)) ;
#42495=DIRECTION('center_axis',(0.408248290463948,-0.816496580927442,-0.408248290464346)) ;
#42496=DIRECTION('ref_axis',(0.577350269189304,0.577350269189986,-0.577350269189588)) ;
#42497=DIRECTION('center_axis',(-2.1716102378779E-15,3.66854633798134E-28,
1.)) ;
#42498=DIRECTION('ref_axis',(0.707106781186452,0.707106781186643,1.53556032529713E-15)) ;
#42499=DIRECTION('center_axis',(1.88526971141291E-28,-2.90739654573716E-15,
-1.)) ;
#42500=DIRECTION('ref_axis',(-1.35627620245787E-13,1.,-2.90739654573716E-15)) ;
#42501=DIRECTION('center_axis',(1.,-1.66533453692587E-16,2.1716102378779E-15)) ;
#42502=DIRECTION('ref_axis',(1.41780339089714E-15,-0.70710678118655,-0.707106781186545)) ;
#42503=DIRECTION('center_axis',(1.,1.35627620245787E-13,-2.05796303467862E-28)) ;
#42504=DIRECTION('ref_axis',(1.35627620245787E-13,-1.,2.90739654573716E-15)) ;
#42505=DIRECTION('',(-1.,1.66533453692587E-16,-2.1716102378779E-15)) ;
#42506=DIRECTION('center_axis',(-1.,-1.35627620245747E-13,2.05796303467745E-28)) ;
#42507=DIRECTION('ref_axis',(1.88526971141291E-28,-2.90739654573716E-15,
-1.)) ;
#42508=DIRECTION('',(1.,-1.66533453692587E-16,2.1716102378779E-15)) ;
#42509=DIRECTION('center_axis',(-1.,6.48092690624107E-15,-2.07369595641671E-28)) ;
#42510=DIRECTION('ref_axis',(0.,-1.,0.)) ;
#42511=DIRECTION('center_axis',(-1.,7.08071943160919E-13,-2.24717289282075E-27)) ;
#42512=DIRECTION('ref_axis',(-1.88526971141296E-28,2.90739654573716E-15,
1.)) ;
#42513=DIRECTION('center_axis',(6.48092690624107E-15,1.,-2.90739654573716E-15)) ;
#42514=DIRECTION('ref_axis',(1.,-6.48092690624107E-15,2.07369595641671E-28)) ;
#42515=DIRECTION('center_axis',(-1.66533453692966E-16,-1.,3.83386399937507E-28)) ;
#42516=DIRECTION('ref_axis',(0.707106781186648,-1.17756934401E-16,-0.707106781186447)) ;
#42517=DIRECTION('center_axis',(-6.48092690624107E-15,-1.,2.90739654573716E-15)) ;
#42518=DIRECTION('ref_axis',(1.88526971141291E-28,-2.90739654573716E-15,
-1.)) ;
#42519=DIRECTION('',(1.66533453692966E-16,1.,-3.83386399937507E-28)) ;
#42520=DIRECTION('center_axis',(1.,-6.48092690624107E-15,2.07369595641671E-28)) ;
#42521=DIRECTION('ref_axis',(0.,1.,0.)) ;
#42522=DIRECTION('center_axis',(1.,-1.48589474058271E-13,-5.59482469102492E-13)) ;
#42523=DIRECTION('ref_axis',(-1.48589474058269E-13,-1.,2.90739654573716E-15)) ;
#42524=DIRECTION('center_axis',(6.48092690624107E-15,1.,-2.90739654573716E-15)) ;
#42525=DIRECTION('ref_axis',(1.88526971141291E-28,-2.90739654573716E-15,
-1.)) ;
#42526=DIRECTION('center_axis',(-1.,6.48092690624107E-15,-2.07369595641671E-28)) ;
#42527=DIRECTION('ref_axis',(0.,-1.,0.)) ;
#42528=DIRECTION('center_axis',(-1.,1.48589474058269E-13,-6.20535494751205E-28)) ;
#42529=DIRECTION('ref_axis',(1.48589474058269E-13,1.,-2.90739654573716E-15)) ;
#42530=DIRECTION('center_axis',(-6.48092690624107E-15,-1.,2.90739654573716E-15)) ;
#42531=DIRECTION('ref_axis',(1.88526971141291E-28,-2.90739654573716E-15,
-1.)) ;
#42532=DIRECTION('center_axis',(1.88526971141291E-28,-2.90739654573716E-15,
-1.)) ;
#42533=DIRECTION('ref_axis',(1.,-6.48092690624108E-15,2.07369595641671E-28)) ;
#42534=DIRECTION('center_axis',(2.1716102378779E-15,-3.66854633798134E-28,
-1.)) ;
#42535=DIRECTION('ref_axis',(0.707106781186543,-0.707106781186552,1.53556032529784E-15)) ;
#42536=DIRECTION('',(2.1716102378779E-15,-3.66854633798134E-28,-1.)) ;
#42537=DIRECTION('center_axis',(-1.66533453692966E-16,-1.,3.83386399937507E-28)) ;
#42538=DIRECTION('ref_axis',(0.707106781186648,-1.17756934401E-16,-0.707106781186447)) ;
#42539=DIRECTION('center_axis',(6.48092690628146E-15,1.,-2.90739654573716E-15)) ;
#42540=DIRECTION('ref_axis',(1.,-6.48092690628146E-15,2.07369595641789E-28)) ;
#42541=DIRECTION('',(1.66533453692966E-16,1.,-3.83386399937507E-28)) ;
#42542=DIRECTION('center_axis',(1.,-6.48092690624107E-15,2.07369595641671E-28)) ;
#42543=DIRECTION('ref_axis',(0.,1.,0.)) ;
#42544=DIRECTION('center_axis',(1.,-1.48589474058269E-13,6.20535494751205E-28)) ;
#42545=DIRECTION('ref_axis',(-1.88526971141292E-28,2.90739654573716E-15,
1.)) ;
#42546=DIRECTION('center_axis',(-6.48092690624107E-15,-1.,2.90739654573716E-15)) ;
#42547=DIRECTION('ref_axis',(-1.,6.48092690624107E-15,-2.07369595641671E-28)) ;
#42548=DIRECTION('center_axis',(8.32667268460789E-17,1.,-3.83780830390118E-28)) ;
#42549=DIRECTION('ref_axis',(-0.707106781186447,5.88784671997906E-17,-0.707106781186648)) ;
#42550=DIRECTION('center_axis',(6.48092690624107E-15,1.,-2.90739654573716E-15)) ;
#42551=DIRECTION('ref_axis',(1.88526971141291E-28,-2.90739654573716E-15,
-1.)) ;
#42552=DIRECTION('',(-8.32667268460789E-17,-1.,3.83780830390118E-28)) ;
#42553=DIRECTION('center_axis',(-1.,3.33066907386739E-16,-2.1716102378779E-15)) ;
#42554=DIRECTION('ref_axis',(-1.30004645649559E-15,0.70710678118655,0.707106781186545)) ;
#42555=DIRECTION('',(-1.,3.33066907386739E-16,-2.1716102378779E-15)) ;
#42556=DIRECTION('',(1.,-3.33066907386739E-16,2.1716102378779E-15)) ;
#42557=DIRECTION('center_axis',(8.32667268460789E-17,1.,-3.83780830390118E-28)) ;
#42558=DIRECTION('ref_axis',(-0.707106781186447,5.88784671997906E-17,-0.707106781186648)) ;
#42559=DIRECTION('center_axis',(-6.48092690624107E-15,-1.,2.90739654573716E-15)) ;
#42560=DIRECTION('ref_axis',(-1.,6.48092690624107E-15,-2.07369595641671E-28)) ;
#42561=DIRECTION('',(-8.32667268460789E-17,-1.,3.83780830390118E-28)) ;
#42562=DIRECTION('center_axis',(1.,-3.33066907386739E-16,2.1716102378779E-15)) ;
#42563=DIRECTION('ref_axis',(-1.77107419409959E-15,-0.707106781186545,0.70710678118655)) ;
#42564=DIRECTION('',(1.,-3.33066907386739E-16,2.1716102378779E-15)) ;
#42565=DIRECTION('center_axis',(-0.81649658092765,0.408248290464166,0.408248290463711)) ;
#42566=DIRECTION('ref_axis',(-0.577350269189702,-0.577350269189929,-0.577350269189247)) ;
#42567=DIRECTION('center_axis',(2.17161023787787E-15,-3.83420712807771E-28,
-1.)) ;
#42568=DIRECTION('ref_axis',(-0.707106781186582,-0.707106781186513,-1.53556032529738E-15)) ;
#42569=DIRECTION('center_axis',(-0.40824829046392,0.408248290464147,-0.816496580927556)) ;
#42570=DIRECTION('ref_axis',(0.577350269189076,-0.577350269189986,-0.577350269189815)) ;
#42571=DIRECTION('center_axis',(1.,-1.66533453692966E-16,2.1716102378779E-15)) ;
#42572=DIRECTION('ref_axis',(1.65331725969831E-15,0.707106781186545,-0.70710678118655)) ;
#42573=DIRECTION('center_axis',(1.,1.35627620245787E-13,-2.05796303467862E-28)) ;
#42574=DIRECTION('ref_axis',(1.8852697114129E-28,-2.90739654573716E-15,
-1.)) ;
#42575=DIRECTION('',(-1.,1.66533453692966E-16,-2.1716102378779E-15)) ;
#42576=DIRECTION('center_axis',(-1.,-1.35627620245787E-13,2.05796303467862E-28)) ;
#42577=DIRECTION('ref_axis',(-1.35627620245787E-13,1.,-2.90739654573716E-15)) ;
#42578=DIRECTION('center_axis',(0.40824829046392,-0.408248290464147,-0.816496580927556)) ;
#42579=DIRECTION('ref_axis',(-0.577350269189834,0.577350269189152,-0.577350269189891)) ;
#42580=DIRECTION('center_axis',(2.17161023787787E-15,-3.83815143260382E-28,
-1.)) ;
#42581=DIRECTION('ref_axis',(-0.707106781186656,0.707106781186439,-1.53556032529808E-15)) ;
#42582=DIRECTION('center_axis',(-0.81649658092765,0.408248290464166,-0.408248290463711)) ;
#42583=DIRECTION('ref_axis',(0.577350269189702,0.577350269189929,-0.577350269189247)) ;
#42584=DIRECTION('center_axis',(-3.33066907386739E-16,-1.,3.66031460022645E-28)) ;
#42585=DIRECTION('ref_axis',(-2.17161023787795E-15,3.66754751528624E-28,
1.)) ;
#42586=DIRECTION('center_axis',(2.1716102378779E-15,-3.83815143260386E-28,
-1.)) ;
#42587=DIRECTION('ref_axis',(1.,-1.66533453692941E-16,2.1716102378779E-15)) ;
#42588=DIRECTION('center_axis',(2.1716102378779E-15,-3.83815143260386E-28,
-1.)) ;
#42589=DIRECTION('ref_axis',(1.,-1.66533453692941E-16,2.1716102378779E-15)) ;
#42590=DIRECTION('center_axis',(2.1716102378779E-15,-3.83815143260386E-28,
-1.)) ;
#42591=DIRECTION('ref_axis',(1.,-1.66533453692941E-16,2.1716102378779E-15)) ;
#42592=DIRECTION('',(-1.66533453692966E-16,-1.,3.83386399937507E-28)) ;
#42593=DIRECTION('',(1.,-1.66533453692587E-16,2.1716102378779E-15)) ;
#42594=DIRECTION('',(8.32667268460789E-17,1.,-3.83780830390118E-28)) ;
#42595=DIRECTION('',(-1.,1.66533453692966E-16,-2.1716102378779E-15)) ;
#42596=DIRECTION('center_axis',(-0.816496580927764,0.408248290464109,0.408248290463541)) ;
#42597=DIRECTION('ref_axis',(-0.577350269189531,-0.577350269189986,-0.57735026918936)) ;
#42598=DIRECTION('center_axis',(1.,1.35627620245787E-13,2.17161023787752E-15)) ;
#42599=DIRECTION('ref_axis',(1.35627620245787E-13,-1.,2.90739654573778E-15)) ;
#42600=DIRECTION('center_axis',(6.48092690624107E-15,1.,-2.90739654573747E-15)) ;
#42601=DIRECTION('ref_axis',(2.17161023787792E-15,-2.90739654573748E-15,
-1.)) ;
#42602=DIRECTION('center_axis',(2.1716102378779E-15,-3.83420712807775E-28,
-1.)) ;
#42603=DIRECTION('ref_axis',(-0.70710678118651,-0.707106781186585,-1.53556032529724E-15)) ;
#42604=DIRECTION('center_axis',(0.40824829046392,-0.408248290464147,-0.816496580927556)) ;
#42605=DIRECTION('ref_axis',(-0.577350269189986,0.577350269189076,-0.577350269189815)) ;
#42606=DIRECTION('center_axis',(-6.48092690624107E-15,-1.,2.90739654573747E-15)) ;
#42607=DIRECTION('ref_axis',(-1.,6.48092690624106E-15,-2.17161023787794E-15)) ;
#42608=DIRECTION('center_axis',(1.,1.35627620245787E-13,2.17161023787752E-15)) ;
#42609=DIRECTION('ref_axis',(2.17161023787791E-15,-2.90739654573749E-15,
-1.)) ;
#42610=DIRECTION('center_axis',(2.1716102378779E-15,-3.83815143260386E-28,
-1.)) ;
#42611=DIRECTION('ref_axis',(-0.707106781186656,0.707106781186439,-1.5355603252981E-15)) ;
#42612=DIRECTION('center_axis',(1.66533453692966E-16,1.,-3.83386399937507E-28)) ;
#42613=DIRECTION('ref_axis',(-0.707106781186596,1.17756934400449E-16,-0.707106781186499)) ;
#42614=DIRECTION('',(1.66533453692966E-16,1.,-3.83386399937507E-28)) ;
#42615=DIRECTION('center_axis',(1.,-1.66533453692966E-16,2.1716102378779E-15)) ;
#42616=DIRECTION('ref_axis',(1.65331725969841E-15,0.707106781186495,-0.7071067811866)) ;
#42617=DIRECTION('center_axis',(1.,1.35627620245787E-13,2.17161023787752E-15)) ;
#42618=DIRECTION('ref_axis',(-1.35627620245787E-13,1.,-2.90739654573778E-15)) ;
#42619=DIRECTION('center_axis',(-1.,1.66533453692587E-16,-2.1716102378779E-15)) ;
#42620=DIRECTION('ref_axis',(1.41780339089726E-15,-0.707106781186499,-0.707106781186596)) ;
#42621=DIRECTION('',(-1.,1.66533453692587E-16,-2.1716102378779E-15)) ;
#42622=DIRECTION('center_axis',(1.,1.35627620245787E-13,2.17161023787752E-15)) ;
#42623=DIRECTION('ref_axis',(2.17161023787792E-15,-2.90739654573749E-15,
-1.)) ;
#42624=DIRECTION('center_axis',(-8.32667268460789E-17,-1.,3.83780830390118E-28)) ;
#42625=DIRECTION('ref_axis',(0.707106781186599,-5.8878467200346E-17,-0.707106781186496)) ;
#42626=DIRECTION('center_axis',(-6.48092690624107E-15,-1.,2.90739654573747E-15)) ;
#42627=DIRECTION('ref_axis',(1.,-6.48092690624106E-15,2.17161023787794E-15)) ;
#42628=DIRECTION('center_axis',(6.48092690624107E-15,1.,-2.90739654573747E-15)) ;
#42629=DIRECTION('ref_axis',(2.17161023787792E-15,-2.90739654573748E-15,
-1.)) ;
#42630=DIRECTION('center_axis',(-0.408248290463939,0.408248290464166,-0.816496580927537)) ;
#42631=DIRECTION('ref_axis',(0.577350269189076,-0.577350269189986,-0.577350269189815)) ;
#42632=DIRECTION('center_axis',(0.408248290463948,-0.816496580927442,-0.408248290464346)) ;
#42633=DIRECTION('ref_axis',(0.577350269189304,0.577350269189986,-0.577350269189588)) ;
#42634=DIRECTION('center_axis',(-2.1716102378779E-15,3.66854633798134E-28,
1.)) ;
#42635=DIRECTION('ref_axis',(0.707106781186452,0.707106781186643,1.53556032529713E-15)) ;
#42636=DIRECTION('center_axis',(1.88526971141291E-28,-2.90739654573716E-15,
-1.)) ;
#42637=DIRECTION('ref_axis',(-1.35627620245787E-13,1.,-2.90739654573716E-15)) ;
#42638=DIRECTION('center_axis',(1.,-1.66533453692587E-16,2.1716102378779E-15)) ;
#42639=DIRECTION('ref_axis',(1.41780339089714E-15,-0.70710678118655,-0.707106781186545)) ;
#42640=DIRECTION('center_axis',(1.,1.35627620245787E-13,-2.05796303467862E-28)) ;
#42641=DIRECTION('ref_axis',(1.35627620245787E-13,-1.,2.90739654573716E-15)) ;
#42642=DIRECTION('',(-1.,1.66533453692587E-16,-2.1716102378779E-15)) ;
#42643=DIRECTION('center_axis',(-1.,-1.35627620245747E-13,2.05796303467745E-28)) ;
#42644=DIRECTION('ref_axis',(1.88526971141291E-28,-2.90739654573716E-15,
-1.)) ;
#42645=DIRECTION('',(1.,-1.66533453692587E-16,2.1716102378779E-15)) ;
#42646=DIRECTION('center_axis',(-1.,6.48092690624107E-15,-2.07369595641671E-28)) ;
#42647=DIRECTION('ref_axis',(0.,-1.,0.)) ;
#42648=DIRECTION('center_axis',(-1.,7.08071943160919E-13,-2.24717289282075E-27)) ;
#42649=DIRECTION('ref_axis',(-1.88526971141296E-28,2.90739654573716E-15,
1.)) ;
#42650=DIRECTION('center_axis',(6.48092690624107E-15,1.,-2.90739654573716E-15)) ;
#42651=DIRECTION('ref_axis',(1.,-6.48092690624107E-15,2.07369595641671E-28)) ;
#42652=DIRECTION('center_axis',(-1.66533453692966E-16,-1.,3.83386399937507E-28)) ;
#42653=DIRECTION('ref_axis',(0.707106781186648,-1.17756934401E-16,-0.707106781186447)) ;
#42654=DIRECTION('center_axis',(-6.48092690624107E-15,-1.,2.90739654573716E-15)) ;
#42655=DIRECTION('ref_axis',(1.88526971141291E-28,-2.90739654573716E-15,
-1.)) ;
#42656=DIRECTION('',(1.66533453692966E-16,1.,-3.83386399937507E-28)) ;
#42657=DIRECTION('center_axis',(1.,-6.48092690624107E-15,2.07369595641671E-28)) ;
#42658=DIRECTION('ref_axis',(0.,1.,0.)) ;
#42659=DIRECTION('center_axis',(1.,-1.48589474058271E-13,-5.59482469102492E-13)) ;
#42660=DIRECTION('ref_axis',(-1.48589474058269E-13,-1.,2.90739654573716E-15)) ;
#42661=DIRECTION('center_axis',(6.48092690624107E-15,1.,-2.90739654573716E-15)) ;
#42662=DIRECTION('ref_axis',(1.88526971141291E-28,-2.90739654573716E-15,
-1.)) ;
#42663=DIRECTION('center_axis',(-1.,6.48092690624107E-15,-2.07369595641671E-28)) ;
#42664=DIRECTION('ref_axis',(0.,-1.,0.)) ;
#42665=DIRECTION('center_axis',(-1.,1.48589474058269E-13,-6.20535494751205E-28)) ;
#42666=DIRECTION('ref_axis',(1.48589474058269E-13,1.,-2.90739654573716E-15)) ;
#42667=DIRECTION('center_axis',(-6.48092690624107E-15,-1.,2.90739654573716E-15)) ;
#42668=DIRECTION('ref_axis',(1.88526971141291E-28,-2.90739654573716E-15,
-1.)) ;
#42669=DIRECTION('center_axis',(1.88526971141291E-28,-2.90739654573716E-15,
-1.)) ;
#42670=DIRECTION('ref_axis',(1.,-6.48092690624108E-15,2.07369595641671E-28)) ;
#42671=DIRECTION('center_axis',(2.1716102378779E-15,-3.66854633798134E-28,
-1.)) ;
#42672=DIRECTION('ref_axis',(0.707106781186543,-0.707106781186552,1.53556032529784E-15)) ;
#42673=DIRECTION('',(2.1716102378779E-15,-3.66854633798134E-28,-1.)) ;
#42674=DIRECTION('center_axis',(-1.66533453692966E-16,-1.,3.83386399937507E-28)) ;
#42675=DIRECTION('ref_axis',(0.707106781186648,-1.17756934401E-16,-0.707106781186447)) ;
#42676=DIRECTION('center_axis',(6.48092690628146E-15,1.,-2.90739654573716E-15)) ;
#42677=DIRECTION('ref_axis',(1.,-6.48092690628146E-15,2.07369595641789E-28)) ;
#42678=DIRECTION('',(1.66533453692966E-16,1.,-3.83386399937507E-28)) ;
#42679=DIRECTION('center_axis',(1.,-6.48092690624107E-15,2.07369595641671E-28)) ;
#42680=DIRECTION('ref_axis',(0.,1.,0.)) ;
#42681=DIRECTION('center_axis',(1.,-1.48589474058269E-13,6.20535494751205E-28)) ;
#42682=DIRECTION('ref_axis',(-1.88526971141292E-28,2.90739654573716E-15,
1.)) ;
#42683=DIRECTION('center_axis',(-6.48092690624107E-15,-1.,2.90739654573716E-15)) ;
#42684=DIRECTION('ref_axis',(-1.,6.48092690624107E-15,-2.07369595641671E-28)) ;
#42685=DIRECTION('center_axis',(8.32667268460789E-17,1.,-3.83780830390118E-28)) ;
#42686=DIRECTION('ref_axis',(-0.707106781186447,5.88784671997906E-17,-0.707106781186648)) ;
#42687=DIRECTION('center_axis',(6.48092690624107E-15,1.,-2.90739654573716E-15)) ;
#42688=DIRECTION('ref_axis',(1.88526971141291E-28,-2.90739654573716E-15,
-1.)) ;
#42689=DIRECTION('',(-8.32667268460789E-17,-1.,3.83780830390118E-28)) ;
#42690=DIRECTION('center_axis',(-1.,3.33066907386739E-16,-2.1716102378779E-15)) ;
#42691=DIRECTION('ref_axis',(-1.30004645649559E-15,0.70710678118655,0.707106781186545)) ;
#42692=DIRECTION('',(-1.,3.33066907386739E-16,-2.1716102378779E-15)) ;
#42693=DIRECTION('',(1.,-3.33066907386739E-16,2.1716102378779E-15)) ;
#42694=DIRECTION('center_axis',(8.32667268460789E-17,1.,-3.83780830390118E-28)) ;
#42695=DIRECTION('ref_axis',(-0.707106781186447,5.88784671997906E-17,-0.707106781186648)) ;
#42696=DIRECTION('center_axis',(-6.48092690624107E-15,-1.,2.90739654573716E-15)) ;
#42697=DIRECTION('ref_axis',(-1.,6.48092690624107E-15,-2.07369595641671E-28)) ;
#42698=DIRECTION('',(-8.32667268460789E-17,-1.,3.83780830390118E-28)) ;
#42699=DIRECTION('center_axis',(1.,-3.33066907386739E-16,2.1716102378779E-15)) ;
#42700=DIRECTION('ref_axis',(-1.77107419409959E-15,-0.707106781186545,0.70710678118655)) ;
#42701=DIRECTION('',(1.,-3.33066907386739E-16,2.1716102378779E-15)) ;
#42702=DIRECTION('center_axis',(-0.81649658092765,0.408248290464166,0.408248290463711)) ;
#42703=DIRECTION('ref_axis',(-0.577350269189702,-0.577350269189929,-0.577350269189247)) ;
#42704=DIRECTION('center_axis',(2.17161023787787E-15,-3.83420712807771E-28,
-1.)) ;
#42705=DIRECTION('ref_axis',(-0.707106781186582,-0.707106781186513,-1.53556032529738E-15)) ;
#42706=DIRECTION('center_axis',(-0.40824829046392,0.408248290464147,-0.816496580927556)) ;
#42707=DIRECTION('ref_axis',(0.577350269189076,-0.577350269189986,-0.577350269189815)) ;
#42708=DIRECTION('center_axis',(1.,-1.66533453692966E-16,2.1716102378779E-15)) ;
#42709=DIRECTION('ref_axis',(1.65331725969831E-15,0.707106781186545,-0.70710678118655)) ;
#42710=DIRECTION('center_axis',(1.,1.35627620245787E-13,-2.05796303467862E-28)) ;
#42711=DIRECTION('ref_axis',(1.8852697114129E-28,-2.90739654573716E-15,
-1.)) ;
#42712=DIRECTION('',(-1.,1.66533453692966E-16,-2.1716102378779E-15)) ;
#42713=DIRECTION('center_axis',(-1.,-1.35627620245787E-13,2.05796303467862E-28)) ;
#42714=DIRECTION('ref_axis',(-1.35627620245787E-13,1.,-2.90739654573716E-15)) ;
#42715=DIRECTION('center_axis',(0.40824829046392,-0.408248290464147,-0.816496580927556)) ;
#42716=DIRECTION('ref_axis',(-0.577350269189834,0.577350269189152,-0.577350269189891)) ;
#42717=DIRECTION('center_axis',(2.17161023787787E-15,-3.83815143260382E-28,
-1.)) ;
#42718=DIRECTION('ref_axis',(-0.707106781186656,0.707106781186439,-1.53556032529808E-15)) ;
#42719=DIRECTION('center_axis',(-0.81649658092765,0.408248290464166,-0.408248290463711)) ;
#42720=DIRECTION('ref_axis',(0.577350269189702,0.577350269189929,-0.577350269189247)) ;
#42721=DIRECTION('center_axis',(-3.33066907386739E-16,-1.,3.66031460022645E-28)) ;
#42722=DIRECTION('ref_axis',(-2.17161023787795E-15,3.66754751528624E-28,
1.)) ;
#42723=DIRECTION('center_axis',(2.1716102378779E-15,-3.83815143260386E-28,
-1.)) ;
#42724=DIRECTION('ref_axis',(1.,-1.66533453692941E-16,2.1716102378779E-15)) ;
#42725=DIRECTION('center_axis',(2.1716102378779E-15,-3.83815143260386E-28,
-1.)) ;
#42726=DIRECTION('ref_axis',(1.,-1.66533453692941E-16,2.1716102378779E-15)) ;
#42727=DIRECTION('center_axis',(2.1716102378779E-15,-3.83815143260386E-28,
-1.)) ;
#42728=DIRECTION('ref_axis',(1.,-1.66533453692941E-16,2.1716102378779E-15)) ;
#42729=DIRECTION('',(-1.66533453692966E-16,-1.,3.83386399937507E-28)) ;
#42730=DIRECTION('',(1.,-1.66533453692587E-16,2.1716102378779E-15)) ;
#42731=DIRECTION('',(8.32667268460789E-17,1.,-3.83780830390118E-28)) ;
#42732=DIRECTION('',(-1.,1.66533453692966E-16,-2.1716102378779E-15)) ;
#42733=DIRECTION('center_axis',(-0.816496580927764,0.408248290464109,0.408248290463541)) ;
#42734=DIRECTION('ref_axis',(-0.577350269189531,-0.577350269189986,-0.57735026918936)) ;
#42735=DIRECTION('center_axis',(1.,1.35627620245787E-13,2.17161023787752E-15)) ;
#42736=DIRECTION('ref_axis',(1.35627620245787E-13,-1.,2.90739654573778E-15)) ;
#42737=DIRECTION('center_axis',(6.48092690624107E-15,1.,-2.90739654573747E-15)) ;
#42738=DIRECTION('ref_axis',(2.17161023787792E-15,-2.90739654573748E-15,
-1.)) ;
#42739=DIRECTION('center_axis',(2.1716102378779E-15,-3.83420712807775E-28,
-1.)) ;
#42740=DIRECTION('ref_axis',(-0.70710678118651,-0.707106781186585,-1.53556032529724E-15)) ;
#42741=DIRECTION('center_axis',(0.40824829046392,-0.408248290464147,-0.816496580927556)) ;
#42742=DIRECTION('ref_axis',(-0.577350269189986,0.577350269189076,-0.577350269189815)) ;
#42743=DIRECTION('center_axis',(-6.48092690624107E-15,-1.,2.90739654573747E-15)) ;
#42744=DIRECTION('ref_axis',(-1.,6.48092690624106E-15,-2.17161023787794E-15)) ;
#42745=DIRECTION('center_axis',(1.,1.35627620245787E-13,2.17161023787752E-15)) ;
#42746=DIRECTION('ref_axis',(2.17161023787791E-15,-2.90739654573749E-15,
-1.)) ;
#42747=DIRECTION('center_axis',(2.1716102378779E-15,-3.83815143260386E-28,
-1.)) ;
#42748=DIRECTION('ref_axis',(-0.707106781186656,0.707106781186439,-1.5355603252981E-15)) ;
#42749=DIRECTION('center_axis',(1.66533453692966E-16,1.,-3.83386399937507E-28)) ;
#42750=DIRECTION('ref_axis',(-0.707106781186596,1.17756934400449E-16,-0.707106781186499)) ;
#42751=DIRECTION('',(1.66533453692966E-16,1.,-3.83386399937507E-28)) ;
#42752=DIRECTION('center_axis',(1.,-1.66533453692966E-16,2.1716102378779E-15)) ;
#42753=DIRECTION('ref_axis',(1.65331725969841E-15,0.707106781186495,-0.7071067811866)) ;
#42754=DIRECTION('center_axis',(1.,1.35627620245787E-13,2.17161023787752E-15)) ;
#42755=DIRECTION('ref_axis',(-1.35627620245787E-13,1.,-2.90739654573778E-15)) ;
#42756=DIRECTION('center_axis',(-1.,1.66533453692587E-16,-2.1716102378779E-15)) ;
#42757=DIRECTION('ref_axis',(1.41780339089726E-15,-0.707106781186499,-0.707106781186596)) ;
#42758=DIRECTION('',(-1.,1.66533453692587E-16,-2.1716102378779E-15)) ;
#42759=DIRECTION('center_axis',(1.,1.35627620245787E-13,2.17161023787752E-15)) ;
#42760=DIRECTION('ref_axis',(2.17161023787792E-15,-2.90739654573749E-15,
-1.)) ;
#42761=DIRECTION('center_axis',(-8.32667268460789E-17,-1.,3.83780830390118E-28)) ;
#42762=DIRECTION('ref_axis',(0.707106781186599,-5.8878467200346E-17,-0.707106781186496)) ;
#42763=DIRECTION('center_axis',(-6.48092690624107E-15,-1.,2.90739654573747E-15)) ;
#42764=DIRECTION('ref_axis',(1.,-6.48092690624106E-15,2.17161023787794E-15)) ;
#42765=DIRECTION('center_axis',(6.48092690624107E-15,1.,-2.90739654573747E-15)) ;
#42766=DIRECTION('ref_axis',(2.17161023787792E-15,-2.90739654573748E-15,
-1.)) ;
#42767=DIRECTION('center_axis',(-0.408248290463939,0.408248290464166,-0.816496580927537)) ;
#42768=DIRECTION('ref_axis',(0.577350269189076,-0.577350269189986,-0.577350269189815)) ;
#42769=DIRECTION('center_axis',(0.408248290463948,-0.816496580927442,-0.408248290464346)) ;
#42770=DIRECTION('ref_axis',(0.577350269189304,0.577350269189986,-0.577350269189588)) ;
#42771=DIRECTION('center_axis',(-2.1716102378779E-15,3.66854633798134E-28,
1.)) ;
#42772=DIRECTION('ref_axis',(0.707106781186452,0.707106781186643,1.53556032529713E-15)) ;
#42773=DIRECTION('center_axis',(1.88526971141291E-28,-2.90739654573716E-15,
-1.)) ;
#42774=DIRECTION('ref_axis',(-1.35627620245787E-13,1.,-2.90739654573716E-15)) ;
#42775=DIRECTION('center_axis',(1.,-1.66533453692587E-16,2.1716102378779E-15)) ;
#42776=DIRECTION('ref_axis',(1.41780339089714E-15,-0.70710678118655,-0.707106781186545)) ;
#42777=DIRECTION('center_axis',(1.,1.35627620245787E-13,-2.05796303467862E-28)) ;
#42778=DIRECTION('ref_axis',(1.35627620245787E-13,-1.,2.90739654573716E-15)) ;
#42779=DIRECTION('',(-1.,1.66533453692587E-16,-2.1716102378779E-15)) ;
#42780=DIRECTION('center_axis',(-1.,-1.35627620245747E-13,2.05796303467745E-28)) ;
#42781=DIRECTION('ref_axis',(1.88526971141291E-28,-2.90739654573716E-15,
-1.)) ;
#42782=DIRECTION('',(1.,-1.66533453692587E-16,2.1716102378779E-15)) ;
#42783=DIRECTION('center_axis',(-1.,6.48092690624107E-15,-2.07369595641671E-28)) ;
#42784=DIRECTION('ref_axis',(0.,-1.,0.)) ;
#42785=DIRECTION('center_axis',(-1.,7.08071943160919E-13,-2.24717289282075E-27)) ;
#42786=DIRECTION('ref_axis',(-1.88526971141296E-28,2.90739654573716E-15,
1.)) ;
#42787=DIRECTION('center_axis',(6.48092690624107E-15,1.,-2.90739654573716E-15)) ;
#42788=DIRECTION('ref_axis',(1.,-6.48092690624107E-15,2.07369595641671E-28)) ;
#42789=DIRECTION('center_axis',(-1.66533453692966E-16,-1.,3.83386399937507E-28)) ;
#42790=DIRECTION('ref_axis',(0.707106781186648,-1.17756934401E-16,-0.707106781186447)) ;
#42791=DIRECTION('center_axis',(-6.48092690624107E-15,-1.,2.90739654573716E-15)) ;
#42792=DIRECTION('ref_axis',(1.88526971141291E-28,-2.90739654573716E-15,
-1.)) ;
#42793=DIRECTION('',(1.66533453692966E-16,1.,-3.83386399937507E-28)) ;
#42794=DIRECTION('center_axis',(1.,-6.48092690624107E-15,2.07369595641671E-28)) ;
#42795=DIRECTION('ref_axis',(0.,1.,0.)) ;
#42796=DIRECTION('center_axis',(1.,-1.48589474058271E-13,-5.59482469102492E-13)) ;
#42797=DIRECTION('ref_axis',(-1.48589474058269E-13,-1.,2.90739654573716E-15)) ;
#42798=DIRECTION('center_axis',(6.48092690624107E-15,1.,-2.90739654573716E-15)) ;
#42799=DIRECTION('ref_axis',(1.88526971141291E-28,-2.90739654573716E-15,
-1.)) ;
#42800=DIRECTION('center_axis',(-1.,6.48092690624107E-15,-2.07369595641671E-28)) ;
#42801=DIRECTION('ref_axis',(0.,-1.,0.)) ;
#42802=DIRECTION('center_axis',(-1.,1.48589474058269E-13,-6.20535494751205E-28)) ;
#42803=DIRECTION('ref_axis',(1.48589474058269E-13,1.,-2.90739654573716E-15)) ;
#42804=DIRECTION('center_axis',(-6.48092690624107E-15,-1.,2.90739654573716E-15)) ;
#42805=DIRECTION('ref_axis',(1.88526971141291E-28,-2.90739654573716E-15,
-1.)) ;
#42806=DIRECTION('center_axis',(1.88526971141291E-28,-2.90739654573716E-15,
-1.)) ;
#42807=DIRECTION('ref_axis',(1.,-6.48092690624108E-15,2.07369595641671E-28)) ;
#42808=DIRECTION('center_axis',(2.1716102378779E-15,-3.66854633798134E-28,
-1.)) ;
#42809=DIRECTION('ref_axis',(0.707106781186543,-0.707106781186552,1.53556032529784E-15)) ;
#42810=DIRECTION('',(2.1716102378779E-15,-3.66854633798134E-28,-1.)) ;
#42811=DIRECTION('center_axis',(-1.66533453692966E-16,-1.,3.83386399937507E-28)) ;
#42812=DIRECTION('ref_axis',(0.707106781186648,-1.17756934401E-16,-0.707106781186447)) ;
#42813=DIRECTION('center_axis',(6.48092690628146E-15,1.,-2.90739654573716E-15)) ;
#42814=DIRECTION('ref_axis',(1.,-6.48092690628146E-15,2.07369595641789E-28)) ;
#42815=DIRECTION('',(1.66533453692966E-16,1.,-3.83386399937507E-28)) ;
#42816=DIRECTION('center_axis',(1.,-6.48092690624107E-15,2.07369595641671E-28)) ;
#42817=DIRECTION('ref_axis',(0.,1.,0.)) ;
#42818=DIRECTION('center_axis',(1.,-1.48589474058269E-13,6.20535494751205E-28)) ;
#42819=DIRECTION('ref_axis',(-1.88526971141292E-28,2.90739654573716E-15,
1.)) ;
#42820=DIRECTION('center_axis',(-6.48092690624107E-15,-1.,2.90739654573716E-15)) ;
#42821=DIRECTION('ref_axis',(-1.,6.48092690624107E-15,-2.07369595641671E-28)) ;
#42822=DIRECTION('center_axis',(8.32667268460789E-17,1.,-3.83780830390118E-28)) ;
#42823=DIRECTION('ref_axis',(-0.707106781186447,5.88784671997906E-17,-0.707106781186648)) ;
#42824=DIRECTION('center_axis',(6.48092690624107E-15,1.,-2.90739654573716E-15)) ;
#42825=DIRECTION('ref_axis',(1.88526971141291E-28,-2.90739654573716E-15,
-1.)) ;
#42826=DIRECTION('',(-8.32667268460789E-17,-1.,3.83780830390118E-28)) ;
#42827=DIRECTION('center_axis',(-1.,3.33066907386739E-16,-2.1716102378779E-15)) ;
#42828=DIRECTION('ref_axis',(-1.30004645649559E-15,0.70710678118655,0.707106781186545)) ;
#42829=DIRECTION('',(-1.,3.33066907386739E-16,-2.1716102378779E-15)) ;
#42830=DIRECTION('',(1.,-3.33066907386739E-16,2.1716102378779E-15)) ;
#42831=DIRECTION('center_axis',(8.32667268460789E-17,1.,-3.83780830390118E-28)) ;
#42832=DIRECTION('ref_axis',(-0.707106781186447,5.88784671997906E-17,-0.707106781186648)) ;
#42833=DIRECTION('center_axis',(-6.48092690624107E-15,-1.,2.90739654573716E-15)) ;
#42834=DIRECTION('ref_axis',(-1.,6.48092690624107E-15,-2.07369595641671E-28)) ;
#42835=DIRECTION('',(-8.32667268460789E-17,-1.,3.83780830390118E-28)) ;
#42836=DIRECTION('center_axis',(1.,-3.33066907386739E-16,2.1716102378779E-15)) ;
#42837=DIRECTION('ref_axis',(-1.77107419409959E-15,-0.707106781186545,0.70710678118655)) ;
#42838=DIRECTION('',(1.,-3.33066907386739E-16,2.1716102378779E-15)) ;
#42839=DIRECTION('center_axis',(-0.81649658092765,0.408248290464166,0.408248290463711)) ;
#42840=DIRECTION('ref_axis',(-0.577350269189702,-0.577350269189929,-0.577350269189247)) ;
#42841=DIRECTION('center_axis',(2.17161023787787E-15,-3.83420712807771E-28,
-1.)) ;
#42842=DIRECTION('ref_axis',(-0.707106781186582,-0.707106781186513,-1.53556032529738E-15)) ;
#42843=DIRECTION('center_axis',(-0.40824829046392,0.408248290464147,-0.816496580927556)) ;
#42844=DIRECTION('ref_axis',(0.577350269189076,-0.577350269189986,-0.577350269189815)) ;
#42845=DIRECTION('center_axis',(1.,-1.66533453692966E-16,2.1716102378779E-15)) ;
#42846=DIRECTION('ref_axis',(1.65331725969831E-15,0.707106781186545,-0.70710678118655)) ;
#42847=DIRECTION('center_axis',(1.,1.35627620245787E-13,-2.05796303467862E-28)) ;
#42848=DIRECTION('ref_axis',(1.8852697114129E-28,-2.90739654573716E-15,
-1.)) ;
#42849=DIRECTION('',(-1.,1.66533453692966E-16,-2.1716102378779E-15)) ;
#42850=DIRECTION('center_axis',(-1.,-1.35627620245787E-13,2.05796303467862E-28)) ;
#42851=DIRECTION('ref_axis',(-1.35627620245787E-13,1.,-2.90739654573716E-15)) ;
#42852=DIRECTION('center_axis',(0.40824829046392,-0.408248290464147,-0.816496580927556)) ;
#42853=DIRECTION('ref_axis',(-0.577350269189834,0.577350269189152,-0.577350269189891)) ;
#42854=DIRECTION('center_axis',(2.17161023787787E-15,-3.83815143260382E-28,
-1.)) ;
#42855=DIRECTION('ref_axis',(-0.707106781186656,0.707106781186439,-1.53556032529808E-15)) ;
#42856=DIRECTION('center_axis',(-0.81649658092765,0.408248290464166,-0.408248290463711)) ;
#42857=DIRECTION('ref_axis',(0.577350269189702,0.577350269189929,-0.577350269189247)) ;
#42858=DIRECTION('center_axis',(-3.33066907386739E-16,-1.,3.66031460022645E-28)) ;
#42859=DIRECTION('ref_axis',(-2.17161023787795E-15,3.66754751528624E-28,
1.)) ;
#42860=DIRECTION('center_axis',(2.1716102378779E-15,-3.83815143260386E-28,
-1.)) ;
#42861=DIRECTION('ref_axis',(1.,-1.66533453692941E-16,2.1716102378779E-15)) ;
#42862=DIRECTION('center_axis',(2.1716102378779E-15,-3.83815143260386E-28,
-1.)) ;
#42863=DIRECTION('ref_axis',(1.,-1.66533453692941E-16,2.1716102378779E-15)) ;
#42864=DIRECTION('center_axis',(2.1716102378779E-15,-3.83815143260386E-28,
-1.)) ;
#42865=DIRECTION('ref_axis',(1.,-1.66533453692941E-16,2.1716102378779E-15)) ;
#42866=DIRECTION('',(-1.66533453692966E-16,-1.,3.83386399937507E-28)) ;
#42867=DIRECTION('',(1.,-1.66533453692587E-16,2.1716102378779E-15)) ;
#42868=DIRECTION('',(8.32667268460789E-17,1.,-3.83780830390118E-28)) ;
#42869=DIRECTION('',(-1.,1.66533453692966E-16,-2.1716102378779E-15)) ;
#42870=DIRECTION('center_axis',(-0.816496580927764,0.408248290464109,0.408248290463541)) ;
#42871=DIRECTION('ref_axis',(-0.577350269189531,-0.577350269189986,-0.57735026918936)) ;
#42872=DIRECTION('center_axis',(1.,1.35627620245787E-13,2.17161023787752E-15)) ;
#42873=DIRECTION('ref_axis',(1.35627620245787E-13,-1.,2.90739654573778E-15)) ;
#42874=DIRECTION('center_axis',(6.48092690624107E-15,1.,-2.90739654573747E-15)) ;
#42875=DIRECTION('ref_axis',(2.17161023787792E-15,-2.90739654573748E-15,
-1.)) ;
#42876=DIRECTION('center_axis',(2.1716102378779E-15,-3.83420712807775E-28,
-1.)) ;
#42877=DIRECTION('ref_axis',(-0.70710678118651,-0.707106781186585,-1.53556032529724E-15)) ;
#42878=DIRECTION('center_axis',(0.40824829046392,-0.408248290464147,-0.816496580927556)) ;
#42879=DIRECTION('ref_axis',(-0.577350269189986,0.577350269189076,-0.577350269189815)) ;
#42880=DIRECTION('center_axis',(-6.48092690624107E-15,-1.,2.90739654573747E-15)) ;
#42881=DIRECTION('ref_axis',(-1.,6.48092690624106E-15,-2.17161023787794E-15)) ;
#42882=DIRECTION('center_axis',(1.,1.35627620245787E-13,2.17161023787752E-15)) ;
#42883=DIRECTION('ref_axis',(2.17161023787791E-15,-2.90739654573749E-15,
-1.)) ;
#42884=DIRECTION('center_axis',(2.1716102378779E-15,-3.83815143260386E-28,
-1.)) ;
#42885=DIRECTION('ref_axis',(-0.707106781186656,0.707106781186439,-1.5355603252981E-15)) ;
#42886=DIRECTION('center_axis',(1.66533453692966E-16,1.,-3.83386399937507E-28)) ;
#42887=DIRECTION('ref_axis',(-0.707106781186596,1.17756934400449E-16,-0.707106781186499)) ;
#42888=DIRECTION('',(1.66533453692966E-16,1.,-3.83386399937507E-28)) ;
#42889=DIRECTION('center_axis',(1.,-1.66533453692966E-16,2.1716102378779E-15)) ;
#42890=DIRECTION('ref_axis',(1.65331725969841E-15,0.707106781186495,-0.7071067811866)) ;
#42891=DIRECTION('center_axis',(1.,1.35627620245787E-13,2.17161023787752E-15)) ;
#42892=DIRECTION('ref_axis',(-1.35627620245787E-13,1.,-2.90739654573778E-15)) ;
#42893=DIRECTION('center_axis',(-1.,1.66533453692587E-16,-2.1716102378779E-15)) ;
#42894=DIRECTION('ref_axis',(1.41780339089726E-15,-0.707106781186499,-0.707106781186596)) ;
#42895=DIRECTION('',(-1.,1.66533453692587E-16,-2.1716102378779E-15)) ;
#42896=DIRECTION('center_axis',(1.,1.35627620245787E-13,2.17161023787752E-15)) ;
#42897=DIRECTION('ref_axis',(2.17161023787792E-15,-2.90739654573749E-15,
-1.)) ;
#42898=DIRECTION('center_axis',(-8.32667268460789E-17,-1.,3.83780830390118E-28)) ;
#42899=DIRECTION('ref_axis',(0.707106781186599,-5.8878467200346E-17,-0.707106781186496)) ;
#42900=DIRECTION('center_axis',(-6.48092690624107E-15,-1.,2.90739654573747E-15)) ;
#42901=DIRECTION('ref_axis',(1.,-6.48092690624106E-15,2.17161023787794E-15)) ;
#42902=DIRECTION('center_axis',(6.48092690624107E-15,1.,-2.90739654573747E-15)) ;
#42903=DIRECTION('ref_axis',(2.17161023787792E-15,-2.90739654573748E-15,
-1.)) ;
#42904=DIRECTION('center_axis',(-0.408248290463939,0.408248290464166,-0.816496580927537)) ;
#42905=DIRECTION('ref_axis',(0.577350269189076,-0.577350269189986,-0.577350269189815)) ;
#42906=DIRECTION('center_axis',(0.408248290463948,-0.816496580927442,-0.408248290464346)) ;
#42907=DIRECTION('ref_axis',(0.577350269189304,0.577350269189986,-0.577350269189588)) ;
#42908=DIRECTION('center_axis',(-2.1716102378779E-15,3.66854633798134E-28,
1.)) ;
#42909=DIRECTION('ref_axis',(0.707106781186452,0.707106781186643,1.53556032529713E-15)) ;
#42910=DIRECTION('center_axis',(1.88526971141291E-28,-2.90739654573716E-15,
-1.)) ;
#42911=DIRECTION('ref_axis',(-1.35627620245787E-13,1.,-2.90739654573716E-15)) ;
#42912=DIRECTION('center_axis',(1.,-1.66533453692587E-16,2.1716102378779E-15)) ;
#42913=DIRECTION('ref_axis',(1.41780339089714E-15,-0.70710678118655,-0.707106781186545)) ;
#42914=DIRECTION('center_axis',(1.,1.35627620245787E-13,-2.05796303467862E-28)) ;
#42915=DIRECTION('ref_axis',(1.35627620245787E-13,-1.,2.90739654573716E-15)) ;
#42916=DIRECTION('',(-1.,1.66533453692587E-16,-2.1716102378779E-15)) ;
#42917=DIRECTION('center_axis',(-1.,-1.35627620245747E-13,2.05796303467745E-28)) ;
#42918=DIRECTION('ref_axis',(1.88526971141291E-28,-2.90739654573716E-15,
-1.)) ;
#42919=DIRECTION('',(1.,-1.66533453692587E-16,2.1716102378779E-15)) ;
#42920=DIRECTION('center_axis',(-1.,6.48092690624107E-15,-2.07369595641671E-28)) ;
#42921=DIRECTION('ref_axis',(0.,-1.,0.)) ;
#42922=DIRECTION('center_axis',(-1.,7.08071943160919E-13,-2.24717289282075E-27)) ;
#42923=DIRECTION('ref_axis',(-1.88526971141296E-28,2.90739654573716E-15,
1.)) ;
#42924=DIRECTION('center_axis',(6.48092690624107E-15,1.,-2.90739654573716E-15)) ;
#42925=DIRECTION('ref_axis',(1.,-6.48092690624107E-15,2.07369595641671E-28)) ;
#42926=DIRECTION('center_axis',(-1.66533453692966E-16,-1.,3.83386399937507E-28)) ;
#42927=DIRECTION('ref_axis',(0.707106781186648,-1.17756934401E-16,-0.707106781186447)) ;
#42928=DIRECTION('center_axis',(-6.48092690624107E-15,-1.,2.90739654573716E-15)) ;
#42929=DIRECTION('ref_axis',(1.88526971141291E-28,-2.90739654573716E-15,
-1.)) ;
#42930=DIRECTION('',(1.66533453692966E-16,1.,-3.83386399937507E-28)) ;
#42931=DIRECTION('center_axis',(1.,-6.48092690624107E-15,2.07369595641671E-28)) ;
#42932=DIRECTION('ref_axis',(0.,1.,0.)) ;
#42933=DIRECTION('center_axis',(1.,-1.48589474058271E-13,-5.59482469102492E-13)) ;
#42934=DIRECTION('ref_axis',(-1.48589474058269E-13,-1.,2.90739654573716E-15)) ;
#42935=DIRECTION('center_axis',(6.48092690624107E-15,1.,-2.90739654573716E-15)) ;
#42936=DIRECTION('ref_axis',(1.88526971141291E-28,-2.90739654573716E-15,
-1.)) ;
#42937=DIRECTION('center_axis',(-1.,6.48092690624107E-15,-2.07369595641671E-28)) ;
#42938=DIRECTION('ref_axis',(0.,-1.,0.)) ;
#42939=DIRECTION('center_axis',(-1.,1.48589474058269E-13,-6.20535494751205E-28)) ;
#42940=DIRECTION('ref_axis',(1.48589474058269E-13,1.,-2.90739654573716E-15)) ;
#42941=DIRECTION('center_axis',(-6.48092690624107E-15,-1.,2.90739654573716E-15)) ;
#42942=DIRECTION('ref_axis',(1.88526971141291E-28,-2.90739654573716E-15,
-1.)) ;
#42943=DIRECTION('center_axis',(1.88526971141291E-28,-2.90739654573716E-15,
-1.)) ;
#42944=DIRECTION('ref_axis',(1.,-6.48092690624108E-15,2.07369595641671E-28)) ;
#42945=DIRECTION('center_axis',(2.1716102378779E-15,-3.66854633798134E-28,
-1.)) ;
#42946=DIRECTION('ref_axis',(0.707106781186543,-0.707106781186552,1.53556032529784E-15)) ;
#42947=DIRECTION('',(2.1716102378779E-15,-3.66854633798134E-28,-1.)) ;
#42948=DIRECTION('center_axis',(-1.66533453692966E-16,-1.,3.83386399937507E-28)) ;
#42949=DIRECTION('ref_axis',(0.707106781186648,-1.17756934401E-16,-0.707106781186447)) ;
#42950=DIRECTION('center_axis',(6.48092690628146E-15,1.,-2.90739654573716E-15)) ;
#42951=DIRECTION('ref_axis',(1.,-6.48092690628146E-15,2.07369595641789E-28)) ;
#42952=DIRECTION('',(1.66533453692966E-16,1.,-3.83386399937507E-28)) ;
#42953=DIRECTION('center_axis',(1.,-6.48092690624107E-15,2.07369595641671E-28)) ;
#42954=DIRECTION('ref_axis',(0.,1.,0.)) ;
#42955=DIRECTION('center_axis',(1.,-1.48589474058269E-13,6.20535494751205E-28)) ;
#42956=DIRECTION('ref_axis',(-1.88526971141292E-28,2.90739654573716E-15,
1.)) ;
#42957=DIRECTION('center_axis',(-6.48092690624107E-15,-1.,2.90739654573716E-15)) ;
#42958=DIRECTION('ref_axis',(-1.,6.48092690624107E-15,-2.07369595641671E-28)) ;
#42959=DIRECTION('center_axis',(8.32667268460789E-17,1.,-3.83780830390118E-28)) ;
#42960=DIRECTION('ref_axis',(-0.707106781186447,5.88784671997906E-17,-0.707106781186648)) ;
#42961=DIRECTION('center_axis',(6.48092690624107E-15,1.,-2.90739654573716E-15)) ;
#42962=DIRECTION('ref_axis',(1.88526971141291E-28,-2.90739654573716E-15,
-1.)) ;
#42963=DIRECTION('',(-8.32667268460789E-17,-1.,3.83780830390118E-28)) ;
#42964=DIRECTION('center_axis',(-1.,3.33066907386739E-16,-2.1716102378779E-15)) ;
#42965=DIRECTION('ref_axis',(-1.30004645649559E-15,0.70710678118655,0.707106781186545)) ;
#42966=DIRECTION('',(-1.,3.33066907386739E-16,-2.1716102378779E-15)) ;
#42967=DIRECTION('',(1.,-3.33066907386739E-16,2.1716102378779E-15)) ;
#42968=DIRECTION('center_axis',(8.32667268460789E-17,1.,-3.83780830390118E-28)) ;
#42969=DIRECTION('ref_axis',(-0.707106781186447,5.88784671997906E-17,-0.707106781186648)) ;
#42970=DIRECTION('center_axis',(-6.48092690624107E-15,-1.,2.90739654573716E-15)) ;
#42971=DIRECTION('ref_axis',(-1.,6.48092690624107E-15,-2.07369595641671E-28)) ;
#42972=DIRECTION('',(-8.32667268460789E-17,-1.,3.83780830390118E-28)) ;
#42973=DIRECTION('center_axis',(1.,-3.33066907386739E-16,2.1716102378779E-15)) ;
#42974=DIRECTION('ref_axis',(-1.77107419409959E-15,-0.707106781186545,0.70710678118655)) ;
#42975=DIRECTION('',(1.,-3.33066907386739E-16,2.1716102378779E-15)) ;
#42976=DIRECTION('center_axis',(-0.81649658092765,0.408248290464166,0.408248290463711)) ;
#42977=DIRECTION('ref_axis',(-0.577350269189702,-0.577350269189929,-0.577350269189247)) ;
#42978=DIRECTION('center_axis',(2.17161023787787E-15,-3.83420712807771E-28,
-1.)) ;
#42979=DIRECTION('ref_axis',(-0.707106781186582,-0.707106781186513,-1.53556032529738E-15)) ;
#42980=DIRECTION('center_axis',(-0.40824829046392,0.408248290464147,-0.816496580927556)) ;
#42981=DIRECTION('ref_axis',(0.577350269189076,-0.577350269189986,-0.577350269189815)) ;
#42982=DIRECTION('center_axis',(1.,-1.66533453692966E-16,2.1716102378779E-15)) ;
#42983=DIRECTION('ref_axis',(1.65331725969831E-15,0.707106781186545,-0.70710678118655)) ;
#42984=DIRECTION('center_axis',(1.,1.35627620245787E-13,-2.05796303467862E-28)) ;
#42985=DIRECTION('ref_axis',(1.8852697114129E-28,-2.90739654573716E-15,
-1.)) ;
#42986=DIRECTION('',(-1.,1.66533453692966E-16,-2.1716102378779E-15)) ;
#42987=DIRECTION('center_axis',(-1.,-1.35627620245787E-13,2.05796303467862E-28)) ;
#42988=DIRECTION('ref_axis',(-1.35627620245787E-13,1.,-2.90739654573716E-15)) ;
#42989=DIRECTION('center_axis',(0.40824829046392,-0.408248290464147,-0.816496580927556)) ;
#42990=DIRECTION('ref_axis',(-0.577350269189834,0.577350269189152,-0.577350269189891)) ;
#42991=DIRECTION('center_axis',(2.17161023787787E-15,-3.83815143260382E-28,
-1.)) ;
#42992=DIRECTION('ref_axis',(-0.707106781186656,0.707106781186439,-1.53556032529808E-15)) ;
#42993=DIRECTION('center_axis',(-0.81649658092765,0.408248290464166,-0.408248290463711)) ;
#42994=DIRECTION('ref_axis',(0.577350269189702,0.577350269189929,-0.577350269189247)) ;
#42995=DIRECTION('center_axis',(-3.33066907386739E-16,-1.,3.66031460022645E-28)) ;
#42996=DIRECTION('ref_axis',(-2.17161023787795E-15,3.66754751528624E-28,
1.)) ;
#42997=DIRECTION('center_axis',(2.1716102378779E-15,-3.83815143260386E-28,
-1.)) ;
#42998=DIRECTION('ref_axis',(1.,-1.66533453692941E-16,2.1716102378779E-15)) ;
#42999=DIRECTION('center_axis',(2.1716102378779E-15,-3.83815143260386E-28,
-1.)) ;
#43000=DIRECTION('ref_axis',(1.,-1.66533453692941E-16,2.1716102378779E-15)) ;
#43001=DIRECTION('center_axis',(2.1716102378779E-15,-3.83815143260386E-28,
-1.)) ;
#43002=DIRECTION('ref_axis',(1.,-1.66533453692941E-16,2.1716102378779E-15)) ;
#43003=DIRECTION('',(-1.66533453692966E-16,-1.,3.83386399937507E-28)) ;
#43004=DIRECTION('',(1.,-1.66533453692587E-16,2.1716102378779E-15)) ;
#43005=DIRECTION('',(8.32667268460789E-17,1.,-3.83780830390118E-28)) ;
#43006=DIRECTION('',(-1.,1.66533453692966E-16,-2.1716102378779E-15)) ;
#43007=DIRECTION('center_axis',(-0.816496580927764,0.408248290464109,0.408248290463541)) ;
#43008=DIRECTION('ref_axis',(-0.577350269189531,-0.577350269189986,-0.57735026918936)) ;
#43009=DIRECTION('center_axis',(1.,1.35627620245787E-13,2.17161023787752E-15)) ;
#43010=DIRECTION('ref_axis',(1.35627620245787E-13,-1.,2.90739654573778E-15)) ;
#43011=DIRECTION('center_axis',(6.48092690624107E-15,1.,-2.90739654573747E-15)) ;
#43012=DIRECTION('ref_axis',(2.17161023787792E-15,-2.90739654573748E-15,
-1.)) ;
#43013=DIRECTION('center_axis',(2.1716102378779E-15,-3.83420712807775E-28,
-1.)) ;
#43014=DIRECTION('ref_axis',(-0.70710678118651,-0.707106781186585,-1.53556032529724E-15)) ;
#43015=DIRECTION('center_axis',(0.40824829046392,-0.408248290464147,-0.816496580927556)) ;
#43016=DIRECTION('ref_axis',(-0.577350269189986,0.577350269189076,-0.577350269189815)) ;
#43017=DIRECTION('center_axis',(-6.48092690624107E-15,-1.,2.90739654573747E-15)) ;
#43018=DIRECTION('ref_axis',(-1.,6.48092690624106E-15,-2.17161023787794E-15)) ;
#43019=DIRECTION('center_axis',(1.,1.35627620245787E-13,2.17161023787752E-15)) ;
#43020=DIRECTION('ref_axis',(2.17161023787791E-15,-2.90739654573749E-15,
-1.)) ;
#43021=DIRECTION('center_axis',(2.1716102378779E-15,-3.83815143260386E-28,
-1.)) ;
#43022=DIRECTION('ref_axis',(-0.707106781186656,0.707106781186439,-1.5355603252981E-15)) ;
#43023=DIRECTION('center_axis',(1.66533453692966E-16,1.,-3.83386399937507E-28)) ;
#43024=DIRECTION('ref_axis',(-0.707106781186596,1.17756934400449E-16,-0.707106781186499)) ;
#43025=DIRECTION('',(1.66533453692966E-16,1.,-3.83386399937507E-28)) ;
#43026=DIRECTION('center_axis',(1.,-1.66533453692966E-16,2.1716102378779E-15)) ;
#43027=DIRECTION('ref_axis',(1.65331725969841E-15,0.707106781186495,-0.7071067811866)) ;
#43028=DIRECTION('center_axis',(1.,1.35627620245787E-13,2.17161023787752E-15)) ;
#43029=DIRECTION('ref_axis',(-1.35627620245787E-13,1.,-2.90739654573778E-15)) ;
#43030=DIRECTION('center_axis',(-1.,1.66533453692587E-16,-2.1716102378779E-15)) ;
#43031=DIRECTION('ref_axis',(1.41780339089726E-15,-0.707106781186499,-0.707106781186596)) ;
#43032=DIRECTION('',(-1.,1.66533453692587E-16,-2.1716102378779E-15)) ;
#43033=DIRECTION('center_axis',(1.,1.35627620245787E-13,2.17161023787752E-15)) ;
#43034=DIRECTION('ref_axis',(2.17161023787792E-15,-2.90739654573749E-15,
-1.)) ;
#43035=DIRECTION('center_axis',(-8.32667268460789E-17,-1.,3.83780830390118E-28)) ;
#43036=DIRECTION('ref_axis',(0.707106781186599,-5.8878467200346E-17,-0.707106781186496)) ;
#43037=DIRECTION('center_axis',(-6.48092690624107E-15,-1.,2.90739654573747E-15)) ;
#43038=DIRECTION('ref_axis',(1.,-6.48092690624106E-15,2.17161023787794E-15)) ;
#43039=DIRECTION('center_axis',(6.48092690624107E-15,1.,-2.90739654573747E-15)) ;
#43040=DIRECTION('ref_axis',(2.17161023787792E-15,-2.90739654573748E-15,
-1.)) ;
#43041=DIRECTION('center_axis',(-0.408248290463939,0.408248290464166,-0.816496580927537)) ;
#43042=DIRECTION('ref_axis',(0.577350269189076,-0.577350269189986,-0.577350269189815)) ;
#43043=DIRECTION('center_axis',(0.408248290463948,-0.816496580927442,-0.408248290464346)) ;
#43044=DIRECTION('ref_axis',(0.577350269189304,0.577350269189986,-0.577350269189588)) ;
#43045=DIRECTION('center_axis',(-1.,1.75658099177411E-13,4.54195640846217E-14)) ;
#43046=DIRECTION('ref_axis',(-1.75658099177411E-13,-1.,6.26847853931514E-43)) ;
#43047=DIRECTION('',(4.54195640846217E-14,-1.7376849751744E-27,1.)) ;
#43048=DIRECTION('',(-4.54195640846217E-14,1.7376849751744E-27,-1.)) ;
#43049=DIRECTION('center_axis',(-1.,1.75658099177411E-13,4.54195640846217E-14)) ;
#43050=DIRECTION('ref_axis',(-1.75658099177411E-13,-1.,6.26847853931514E-43)) ;
#43051=DIRECTION('',(-4.54195640846217E-14,1.7376849751744E-27,-1.)) ;
#43052=DIRECTION('',(4.54195640846217E-14,-1.7376849751744E-27,1.)) ;
#43053=DIRECTION('center_axis',(-1.,1.75658099177411E-13,4.54195640846217E-14)) ;
#43054=DIRECTION('ref_axis',(-1.75658099177411E-13,-1.,6.26847853931514E-43)) ;
#43055=DIRECTION('',(-4.54195640846217E-14,1.7376849751744E-27,-1.)) ;
#43056=DIRECTION('',(4.54195640846217E-14,-1.7376849751744E-27,1.)) ;
#43057=DIRECTION('center_axis',(-1.,1.75658099177411E-13,4.54195640846217E-14)) ;
#43058=DIRECTION('ref_axis',(-1.75658099177411E-13,-1.,6.26847853931514E-43)) ;
#43059=DIRECTION('',(-4.54195640846217E-14,1.7376849751744E-27,-1.)) ;
#43060=DIRECTION('',(4.54195640846217E-14,-1.7376849751744E-27,1.)) ;
#43061=DIRECTION('center_axis',(-1.,1.75658099177411E-13,4.54195640846217E-14)) ;
#43062=DIRECTION('ref_axis',(-1.75658099177411E-13,-1.,6.26847853931514E-43)) ;
#43063=DIRECTION('',(-4.54195640846217E-14,1.7376849751744E-27,-1.)) ;
#43064=DIRECTION('',(4.54195640846217E-14,-1.7376849751744E-27,1.)) ;
#43065=DIRECTION('center_axis',(-1.,1.75658099177411E-13,4.54195640846217E-14)) ;
#43066=DIRECTION('ref_axis',(-1.75658099177411E-13,-1.,6.26847853931514E-43)) ;
#43067=DIRECTION('',(-4.54195640846217E-14,1.7376849751744E-27,-1.)) ;
#43068=DIRECTION('',(4.54195640846217E-14,-1.7376849751744E-27,1.)) ;
#43069=DIRECTION('center_axis',(-1.,1.75658099177411E-13,4.54195640846217E-14)) ;
#43070=DIRECTION('ref_axis',(-1.75658099177411E-13,-1.,6.26847853931514E-43)) ;
#43071=DIRECTION('',(-4.54195640846217E-14,1.7376849751744E-27,-1.)) ;
#43072=DIRECTION('',(4.54195640846217E-14,-1.7376849751744E-27,1.)) ;
#43073=DIRECTION('center_axis',(-1.,1.75658099177411E-13,4.54195640846217E-14)) ;
#43074=DIRECTION('ref_axis',(-1.75658099177411E-13,-1.,6.26847853931514E-43)) ;
#43075=DIRECTION('',(-4.54195640846217E-14,1.7376849751744E-27,-1.)) ;
#43076=DIRECTION('',(4.54195640846217E-14,-1.7376849751744E-27,1.)) ;
#43077=DIRECTION('center_axis',(-1.,1.75658099177411E-13,4.54195640846217E-14)) ;
#43078=DIRECTION('ref_axis',(-1.75658099177411E-13,-1.,6.26847853931514E-43)) ;
#43079=DIRECTION('',(-4.54195640846217E-14,1.7376849751744E-27,-1.)) ;
#43080=DIRECTION('',(4.54195640846217E-14,-1.7376849751744E-27,1.)) ;
#43081=DIRECTION('center_axis',(-1.75658099177411E-13,-1.,6.24062931739685E-27)) ;
#43082=DIRECTION('ref_axis',(1.,-1.75658099177411E-13,-4.54195640846217E-14)) ;
#43083=DIRECTION('',(4.54195640846217E-14,-1.7376849751744E-27,1.)) ;
#43084=DIRECTION('center_axis',(1.75658099177411E-13,1.,-6.24062931739685E-27)) ;
#43085=DIRECTION('ref_axis',(-1.,1.75658099177411E-13,4.54195640846217E-14)) ;
#43086=DIRECTION('',(-4.54195640846217E-14,1.7376849751744E-27,-1.)) ;
#43087=DIRECTION('center_axis',(1.75658099177411E-13,1.,-6.24062931739685E-27)) ;
#43088=DIRECTION('ref_axis',(-1.,1.75658099177411E-13,4.54195640846217E-14)) ;
#43089=DIRECTION('',(-4.54195640846217E-14,1.7376849751744E-27,-1.)) ;
#43090=DIRECTION('center_axis',(-1.75658099177411E-13,-1.,6.24062931739685E-27)) ;
#43091=DIRECTION('ref_axis',(1.,-1.75658099177411E-13,-4.54195640846217E-14)) ;
#43092=DIRECTION('',(4.54195640846217E-14,-1.7376849751744E-27,1.)) ;
#43093=DIRECTION('center_axis',(1.75658099177411E-13,1.,-6.24062931739685E-27)) ;
#43094=DIRECTION('ref_axis',(-1.,1.75658099177411E-13,4.54195640846217E-14)) ;
#43095=DIRECTION('',(-4.54195640846217E-14,1.7376849751744E-27,-1.)) ;
#43096=DIRECTION('center_axis',(-1.75658099177411E-13,-1.,6.24062931739685E-27)) ;
#43097=DIRECTION('ref_axis',(1.,-1.75658099177411E-13,-4.54195640846217E-14)) ;
#43098=DIRECTION('',(4.54195640846217E-14,-1.7376849751744E-27,1.)) ;
#43099=DIRECTION('center_axis',(-1.75658099177411E-13,-1.,6.24062931739685E-27)) ;
#43100=DIRECTION('ref_axis',(1.,-1.75658099177411E-13,-4.54195640846217E-14)) ;
#43101=DIRECTION('',(4.54195640846217E-14,-1.7376849751744E-27,1.)) ;
#43102=DIRECTION('center_axis',(1.75658099177411E-13,1.,-6.24062931739685E-27)) ;
#43103=DIRECTION('ref_axis',(-1.,1.75658099177411E-13,4.54195640846217E-14)) ;
#43104=DIRECTION('',(-4.54195640846217E-14,1.7376849751744E-27,-1.)) ;
#43105=DIRECTION('center_axis',(-1.75658099177411E-13,-1.,6.24062931739685E-27)) ;
#43106=DIRECTION('ref_axis',(1.,-1.75658099177411E-13,-4.54195640846217E-14)) ;
#43107=DIRECTION('',(4.54195640846217E-14,-1.7376849751744E-27,1.)) ;
#43108=DIRECTION('center_axis',(1.75658099177411E-13,1.,-6.24062931739685E-27)) ;
#43109=DIRECTION('ref_axis',(-1.,1.75658099177411E-13,4.54195640846217E-14)) ;
#43110=DIRECTION('',(-4.54195640846217E-14,1.7376849751744E-27,-1.)) ;
#43111=DIRECTION('center_axis',(1.75658099177411E-13,1.,-6.24062931739685E-27)) ;
#43112=DIRECTION('ref_axis',(-1.,1.75658099177411E-13,4.54195640846217E-14)) ;
#43113=DIRECTION('',(-4.54195640846217E-14,1.7376849751744E-27,-1.)) ;
#43114=DIRECTION('center_axis',(-1.75658099177411E-13,-1.,6.24062931739685E-27)) ;
#43115=DIRECTION('ref_axis',(1.,-1.75658099177411E-13,-4.54195640846217E-14)) ;
#43116=DIRECTION('',(4.54195640846217E-14,-1.7376849751744E-27,1.)) ;
#43117=DIRECTION('center_axis',(1.75658099177411E-13,1.,-6.24062931739685E-27)) ;
#43118=DIRECTION('ref_axis',(-1.,1.75658099177411E-13,4.54195640846217E-14)) ;
#43119=DIRECTION('',(-4.54195640846217E-14,1.7376849751744E-27,-1.)) ;
#43120=DIRECTION('center_axis',(-1.75658099177411E-13,-1.,6.24062931739685E-27)) ;
#43121=DIRECTION('ref_axis',(1.,-1.75658099177411E-13,-4.54195640846217E-14)) ;
#43122=DIRECTION('',(4.54195640846217E-14,-1.7376849751744E-27,1.)) ;
#43123=DIRECTION('center_axis',(1.75658099177411E-13,1.,-6.24062931739685E-27)) ;
#43124=DIRECTION('ref_axis',(-1.,1.75658099177411E-13,4.54195640846217E-14)) ;
#43125=DIRECTION('',(-4.54195640846217E-14,1.7376849751744E-27,-1.)) ;
#43126=DIRECTION('center_axis',(-1.75658099177411E-13,-1.,6.24062931739685E-27)) ;
#43127=DIRECTION('ref_axis',(1.,-1.75658099177411E-13,-4.54195640846217E-14)) ;
#43128=DIRECTION('',(4.54195640846217E-14,-1.7376849751744E-27,1.)) ;
#43129=DIRECTION('center_axis',(-1.75658099177411E-13,-1.,6.24062931739685E-27)) ;
#43130=DIRECTION('ref_axis',(1.,-1.75658099177411E-13,-4.54195640846217E-14)) ;
#43131=DIRECTION('',(4.54195640846217E-14,-1.7376849751744E-27,1.)) ;
#43132=DIRECTION('center_axis',(1.75658099177411E-13,1.,-6.24062931739685E-27)) ;
#43133=DIRECTION('ref_axis',(-1.,1.75658099177411E-13,4.54195640846217E-14)) ;
#43134=DIRECTION('',(-4.54195640846217E-14,1.7376849751744E-27,-1.)) ;
#43135=DIRECTION('center_axis',(-4.54195640846217E-14,1.66321791214601E-16,
-1.)) ;
#43136=DIRECTION('ref_axis',(-1.,1.75658099177411E-13,4.54195640846217E-14)) ;
#43137=DIRECTION('',(1.,-3.03555657665211E-13,-4.54195640846217E-14)) ;
#43138=DIRECTION('',(-5.71613981083074E-11,-1.,-1.66321788618356E-16)) ;
#43139=DIRECTION('',(-1.,1.75658099177411E-13,4.54195640846217E-14)) ;
#43140=DIRECTION('',(-1.75658099177411E-13,-1.,-1.53926195610211E-16)) ;
#43141=DIRECTION('',(1.,-3.04147775991511E-13,-4.54195640846217E-14)) ;
#43142=DIRECTION('',(-5.71613981083074E-11,-1.,-1.66321788618356E-16)) ;
#43143=DIRECTION('',(-1.,1.75658099177411E-13,4.54195640846217E-14)) ;
#43144=DIRECTION('',(-1.75658099177411E-13,-1.,-1.53926195610211E-16)) ;
#43145=DIRECTION('',(1.,-3.03555657665211E-13,-4.54195640846217E-14)) ;
#43146=DIRECTION('',(-5.71613981083074E-11,-1.,-1.66321788618356E-16)) ;
#43147=DIRECTION('',(-1.,1.75658099177411E-13,4.54195640846217E-14)) ;
#43148=DIRECTION('',(-1.75658099177411E-13,-1.,-1.53926195610211E-16)) ;
#43149=DIRECTION('',(1.,-3.04147775991511E-13,-4.54195640846217E-14)) ;
#43150=DIRECTION('',(-5.71613981083074E-11,-1.,-1.66321788618356E-16)) ;
#43151=DIRECTION('',(-1.,1.75658099177411E-13,4.54195640846217E-14)) ;
#43152=DIRECTION('',(-1.75658099177411E-13,-1.,-1.53926195610211E-16)) ;
#43153=DIRECTION('',(1.,-3.03555657665211E-13,-4.54195640846217E-14)) ;
#43154=DIRECTION('',(-5.71613981083074E-11,-1.,-1.66321788618356E-16)) ;
#43155=DIRECTION('',(1.,-4.6576303444911E-14,-4.54195640846217E-14)) ;
#43156=DIRECTION('',(-1.75658099177411E-13,-1.,-1.53926195610211E-16)) ;
#43157=DIRECTION('',(1.,-3.03555657665211E-13,-4.54195640846217E-14)) ;
#43158=DIRECTION('',(-5.71613981083074E-11,-1.,-1.66321788618356E-16)) ;
#43159=DIRECTION('',(1.,-4.77605401030109E-14,-4.54195640846217E-14)) ;
#43160=DIRECTION('',(-1.75658099177411E-13,-1.,-1.53926195610211E-16)) ;
#43161=DIRECTION('',(1.,-3.03555657665211E-13,-4.54195640846217E-14)) ;
#43162=DIRECTION('',(-5.71613981083074E-11,-1.,-1.66321788618356E-16)) ;
#43163=DIRECTION('',(1.,-4.6576303444911E-14,-4.54195640846217E-14)) ;
#43164=DIRECTION('',(-1.75658099177411E-13,-1.,-1.53926195610211E-16)) ;
#43165=DIRECTION('',(1.,-3.03555657665211E-13,-4.54195640846217E-14)) ;
#43166=DIRECTION('',(-5.71613981083074E-11,-1.,-1.66321788618356E-16)) ;
#43167=DIRECTION('',(1.,-4.6576304037011E-14,-4.54195640846217E-14)) ;
#43168=DIRECTION('',(-1.75658099177411E-13,-1.,-1.53926195610211E-16)) ;
#43169=DIRECTION('',(1.,-3.03555657665211E-13,-4.54195640846217E-14)) ;
#43170=DIRECTION('',(-5.71613981083074E-11,-1.,-1.66321788618356E-16)) ;
#43171=DIRECTION('',(-1.,1.73688224296914E-13,4.53957858957841E-14)) ;
#43172=DIRECTION('',(1.75658099177411E-13,1.,1.53926195610211E-16)) ;
#43173=DIRECTION('',(-1.,1.73688224296914E-13,4.53957858957841E-14)) ;
#43174=DIRECTION('',(-5.71613981083074E-11,-1.,-1.66321788618356E-16)) ;
#43175=DIRECTION('',(1.,-1.75658099177411E-13,-4.54195640846217E-14)) ;
#43176=DIRECTION('',(-1.75658099177411E-13,-1.,-1.53926195610211E-16)) ;
#43177=DIRECTION('center_axis',(1.75658099177411E-13,1.,1.66321791206623E-16)) ;
#43178=DIRECTION('ref_axis',(0.707112705703078,-1.24327680069036E-13,0.707100856620378)) ;
#43179=DIRECTION('center_axis',(4.97494589055058E-8,0.999847695517053,-0.0174523857749279)) ;
#43180=DIRECTION('ref_axis',(-1.30137752939697E-5,-0.0174523857728027,-0.999847695432399)) ;
#43181=DIRECTION('',(1.75658099174892E-13,1.,-5.54473693597788E-11)) ;
#43182=DIRECTION('center_axis',(4.97533257450734E-8,-0.999847695517151,
-0.0174523857693158)) ;
#43183=DIRECTION('ref_axis',(1.30102029465389E-5,-0.0174523857671916,0.999847695432543)) ;
#43184=DIRECTION('center_axis',(-1.74838664905478E-13,-0.999847695156391,
0.0174524064372797)) ;
#43185=DIRECTION('ref_axis',(4.84783030058612E-14,0.0174524064372797,0.999847695156391)) ;
#43186=DIRECTION('',(4.84783030059014E-14,0.0174524064375096,0.999847695156387)) ;
#43187=DIRECTION('',(0.707052927141238,-0.0123416547510578,-0.707052927141252)) ;
#43188=DIRECTION('',(-4.84783030058629E-14,-0.0174524064372897,-0.999847695156391)) ;
#43189=DIRECTION('center_axis',(1.75658099177411E-13,1.,1.66321791206623E-16)) ;
#43190=DIRECTION('ref_axis',(0.70711270570306,-1.24327680069032E-13,0.707100856620396)) ;
#43191=DIRECTION('',(1.75658099174892E-13,1.,-5.54473693597788E-11)) ;
#43192=DIRECTION('center_axis',(4.97533257450734E-8,-0.999847695517151,
-0.0174523857693158)) ;
#43193=DIRECTION('ref_axis',(1.30083962602235E-5,-0.0174523857671921,0.999847695432567)) ;
#43194=DIRECTION('center_axis',(4.97494589055058E-8,0.999847695517053,-0.0174523857749279)) ;
#43195=DIRECTION('ref_axis',(-1.30106570826674E-5,-0.0174523857728036,-0.999847695432439)) ;
#43196=DIRECTION('center_axis',(1.75658099177411E-13,1.,1.66321791206623E-16)) ;
#43197=DIRECTION('ref_axis',(0.707112705703065,-1.24327680069033E-13,0.707100856620391)) ;
#43198=DIRECTION('center_axis',(4.97494589055058E-8,0.999847695517053,-0.0174523857749279)) ;
#43199=DIRECTION('ref_axis',(-1.30137786494106E-5,-0.0174523857728027,-0.999847695432399)) ;
#43200=DIRECTION('',(1.75658099174892E-13,1.,-5.54473693597788E-11)) ;
#43201=DIRECTION('center_axis',(4.97533257450734E-8,-0.999847695517151,
-0.0174523857693158)) ;
#43202=DIRECTION('ref_axis',(1.30100135812283E-5,-0.0174523857671916,0.999847695432546)) ;
#43203=DIRECTION('center_axis',(1.75658099177411E-13,1.,1.66321791206623E-16)) ;
#43204=DIRECTION('ref_axis',(0.707112705703077,-1.24327680069035E-13,0.707100856620379)) ;
#43205=DIRECTION('center_axis',(4.97494470609749E-8,0.999847695517053,-0.0174523857749161)) ;
#43206=DIRECTION('ref_axis',(-1.30088130075626E-5,-0.0174523857727923,-0.999847695432464)) ;
#43207=DIRECTION('',(1.75658099174892E-13,1.,-5.54473693597788E-11)) ;
#43208=DIRECTION('center_axis',(4.97533257450734E-8,-0.999847695517151,
-0.0174523857693158)) ;
#43209=DIRECTION('ref_axis',(1.30145516036281E-5,-0.0174523857671904,0.999847695432487)) ;
#43210=DIRECTION('center_axis',(1.75658099177411E-13,1.,1.66321791206623E-16)) ;
#43211=DIRECTION('ref_axis',(0.707112705703066,-1.24327680069033E-13,0.70710085662039)) ;
#43212=DIRECTION('',(1.75658099174892E-13,1.,-5.54473693597788E-11)) ;
#43213=DIRECTION('center_axis',(4.97533257450734E-8,-0.999847695517151,
-0.0174523857693158)) ;
#43214=DIRECTION('ref_axis',(1.30102029465389E-5,-0.0174523857671916,0.999847695432543)) ;
#43215=DIRECTION('center_axis',(4.97400119840491E-8,0.999847695516655,-0.0174523857976883)) ;
#43216=DIRECTION('ref_axis',(-1.30177007513301E-5,-0.0174523857955622,-0.999847695431951)) ;
#43217=DIRECTION('center_axis',(1.75658099177411E-13,1.,1.66321791206623E-16)) ;
#43218=DIRECTION('ref_axis',(0.707112705703067,-1.24327680069034E-13,0.707100856620389)) ;
#43219=DIRECTION('',(1.75658099174892E-13,1.,-5.54473693597788E-11)) ;
#43220=DIRECTION('center_axis',(4.97533090048031E-8,-0.99984769551715,-0.0174523857693562)) ;
#43221=DIRECTION('ref_axis',(1.30090361591441E-5,-0.0174523857672323,0.999847695432558)) ;
#43222=DIRECTION('center_axis',(4.9749430318237E-8,0.999847695517052,-0.0174523857749565)) ;
#43223=DIRECTION('ref_axis',(-1.30139248551185E-5,-0.0174523857728313,-0.999847695432396)) ;
#43224=DIRECTION('center_axis',(1.75658099177411E-13,1.,1.66321791206623E-16)) ;
#43225=DIRECTION('ref_axis',(0.707112705703064,-1.24327680069033E-13,0.707100856620392)) ;
#43226=DIRECTION('',(1.75658099174892E-13,1.,-5.54473693597788E-11)) ;
#43227=DIRECTION('center_axis',(4.97533257450734E-8,-0.999847695517151,
-0.0174523857693158)) ;
#43228=DIRECTION('ref_axis',(1.30096219496208E-5,-0.0174523857671917,0.999847695432551)) ;
#43229=DIRECTION('center_axis',(4.97494017334358E-8,0.999847695517052,-0.0174523857749851)) ;
#43230=DIRECTION('ref_axis',(-1.3016906447811E-5,-0.0174523857728591,-0.999847695432357)) ;
#43231=DIRECTION('center_axis',(1.75658099177411E-13,1.,1.66321791206623E-16)) ;
#43232=DIRECTION('ref_axis',(0.707112705703086,-1.24327680069037E-13,0.70710085662037)) ;
#43233=DIRECTION('center_axis',(4.97494589055058E-8,0.999847695517053,-0.0174523857749279)) ;
#43234=DIRECTION('ref_axis',(-1.30141587811237E-5,-0.0174523857728026,-0.999847695432394)) ;
#43235=DIRECTION('',(1.75658099174892E-13,1.,-5.54473693597788E-11)) ;
#43236=DIRECTION('center_axis',(4.97533090048031E-8,-0.99984769551715,-0.0174523857693562)) ;
#43237=DIRECTION('ref_axis',(1.30078195775241E-5,-0.0174523857672326,0.999847695432574)) ;
#43238=DIRECTION('center_axis',(1.75658099177411E-13,1.,1.66321791206623E-16)) ;
#43239=DIRECTION('ref_axis',(0.707112705703071,-1.24327680069034E-13,0.707100856620385)) ;
#43240=DIRECTION('',(1.75658099174892E-13,1.,-5.54473693597888E-11)) ;
#43241=DIRECTION('center_axis',(4.96835356766386E-8,-0.999847695515933,
-0.0174523858390597)) ;
#43242=DIRECTION('ref_axis',(1.30149063904817E-5,-0.0174523858369351,0.999847695431265)) ;
#43243=DIRECTION('center_axis',(4.97172307340419E-8,0.999847695516491,-0.0174523858071221)) ;
#43244=DIRECTION('ref_axis',(-1.29996074717629E-5,-0.0174523858050013,-0.999847695432021)) ;
#43245=DIRECTION('center_axis',(1.76424026290696E-13,0.999847695156391,
0.01745240643728)) ;
#43246=DIRECTION('ref_axis',(-4.23469899241728E-14,0.01745240643728,-0.999847695156391)) ;
#43247=DIRECTION('center_axis',(4.97533257450734E-8,-0.999847695517151,
-0.0174523857693158)) ;
#43248=DIRECTION('ref_axis',(1.30096219496208E-5,-0.0174523857671917,0.999847695432551)) ;
#43249=DIRECTION('',(4.2346989924171E-14,-0.01745240643729,0.999847695156391)) ;
#43250=DIRECTION('',(-0.707052927141242,-0.0123416547508096,0.707052927141252)) ;
#43251=DIRECTION('',(-4.23469899241322E-14,0.0174524064375099,-0.999847695156387)) ;
#43252=DIRECTION('center_axis',(1.75658099177411E-13,1.,1.66321791206623E-16)) ;
#43253=DIRECTION('ref_axis',(0.707112705703064,-1.24327680069033E-13,0.707100856620392)) ;
#43254=DIRECTION('',(1.75658099174892E-13,1.,-5.54473693597788E-11)) ;
#43255=DIRECTION('center_axis',(4.97494589055058E-8,0.999847695517053,-0.0174523857749279)) ;
#43256=DIRECTION('ref_axis',(-1.30106494130138E-5,-0.0174523857728036,-0.999847695432439)) ;
#43257=DIRECTION('center_axis',(0.707106781186554,-1.24326640365109E-13,
0.707106781186541)) ;
#43258=DIRECTION('ref_axis',(0.707106781186541,-2.04517587165981E-30,-0.707106781186554)) ;
#43259=DIRECTION('',(1.75658099177411E-13,1.,1.66321791206623E-16)) ;
#43260=DIRECTION('center_axis',(0.707106781186548,-1.24326640365108E-13,
0.707106781186548)) ;
#43261=DIRECTION('ref_axis',(0.707106781186548,7.39148474710689E-31,-0.707106781186548)) ;
#43262=DIRECTION('',(-0.707052927141248,-0.0123416547508095,0.707052927141246)) ;
#43263=DIRECTION('',(1.75658099177411E-13,1.,1.66321791206623E-16)) ;
#43264=DIRECTION('',(0.707052927141244,-0.0123416547510577,-0.707052927141246)) ;
#43265=DIRECTION('',(-1.75658099177411E-13,-1.,-1.66321791206623E-16)) ;
#43266=DIRECTION('center_axis',(0.707106781186548,-1.24326640365108E-13,
0.707106781186548)) ;
#43267=DIRECTION('ref_axis',(0.707106781186548,7.39148474710689E-31,-0.707106781186548)) ;
#43268=DIRECTION('',(-0.707052927141248,-0.0123416547508095,0.707052927141246)) ;
#43269=DIRECTION('',(1.75658099177411E-13,1.,1.66321791206623E-16)) ;
#43270=DIRECTION('',(0.707052927141244,-0.0123416547510577,-0.707052927141246)) ;
#43271=DIRECTION('',(-1.75658099177411E-13,-1.,-1.66321791206623E-16)) ;
#43272=DIRECTION('center_axis',(0.707106781186554,-1.24326640365109E-13,
0.707106781186541)) ;
#43273=DIRECTION('ref_axis',(0.707106781186541,-2.04517587165981E-30,-0.707106781186554)) ;
#43274=DIRECTION('',(-0.707052927141242,-0.0123416547508096,0.707052927141252)) ;
#43275=DIRECTION('',(1.75658099177411E-13,1.,1.66321791206623E-16)) ;
#43276=DIRECTION('',(0.707052927141238,-0.0123416547510578,-0.707052927141252)) ;
#43277=DIRECTION('',(-1.75658099177411E-13,-1.,-1.66321791206623E-16)) ;
#43278=DIRECTION('center_axis',(0.707106781186548,-1.24326640365108E-13,
0.707106781186548)) ;
#43279=DIRECTION('ref_axis',(0.707106781186548,7.39148474710689E-31,-0.707106781186548)) ;
#43280=DIRECTION('',(-0.707052927141248,-0.0123416547508095,0.707052927141246)) ;
#43281=DIRECTION('',(1.75658099177411E-13,1.,1.66321791206623E-16)) ;
#43282=DIRECTION('',(0.707052927141244,-0.0123416547510577,-0.707052927141246)) ;
#43283=DIRECTION('',(-1.75658099177411E-13,-1.,-1.66321791206623E-16)) ;
#43284=DIRECTION('center_axis',(0.707106781186548,-1.24326640365108E-13,
0.707106781186548)) ;
#43285=DIRECTION('ref_axis',(0.707106781186548,7.39148474710689E-31,-0.707106781186548)) ;
#43286=DIRECTION('',(-0.707052927141248,-0.0123416547508095,0.707052927141246)) ;
#43287=DIRECTION('',(1.75658099177411E-13,1.,1.66321791206623E-16)) ;
#43288=DIRECTION('',(0.707052927141244,-0.0123416547510577,-0.707052927141246)) ;
#43289=DIRECTION('',(-1.75658099177411E-13,-1.,-1.66321791206623E-16)) ;
#43290=DIRECTION('center_axis',(0.707106781186548,-1.24326640365108E-13,
0.707106781186548)) ;
#43291=DIRECTION('ref_axis',(0.707106781186548,7.39148474710689E-31,-0.707106781186548)) ;
#43292=DIRECTION('',(-0.707052927141248,-0.0123416547508095,0.707052927141246)) ;
#43293=DIRECTION('',(1.75658099177411E-13,1.,1.66321791206623E-16)) ;
#43294=DIRECTION('',(0.707052927141244,-0.0123416547510577,-0.707052927141246)) ;
#43295=DIRECTION('',(-1.75658099177411E-13,-1.,-1.66321791206623E-16)) ;
#43296=DIRECTION('center_axis',(0.707106781186548,-1.24326640365108E-13,
0.707106781186548)) ;
#43297=DIRECTION('ref_axis',(0.707106781186548,7.39148474710689E-31,-0.707106781186548)) ;
#43298=DIRECTION('',(-0.707052927141248,-0.0123416547508095,0.707052927141246)) ;
#43299=DIRECTION('',(1.75658099177411E-13,1.,1.66321791206623E-16)) ;
#43300=DIRECTION('',(0.707052927141244,-0.0123416547510577,-0.707052927141246)) ;
#43301=DIRECTION('',(-1.75658099177411E-13,-1.,-1.66321791206623E-16)) ;
#43302=DIRECTION('center_axis',(0.707106781186554,-1.24326640365109E-13,
0.707106781186541)) ;
#43303=DIRECTION('ref_axis',(0.707106781186541,-2.04517587165981E-30,-0.707106781186554)) ;
#43304=DIRECTION('',(-0.707052927141242,-0.0123416547508096,0.707052927141252)) ;
#43305=DIRECTION('',(1.75658099177411E-13,1.,1.66321791206623E-16)) ;
#43306=DIRECTION('',(0.707052927141238,-0.0123416547510578,-0.707052927141252)) ;
#43307=DIRECTION('',(-1.75658099177411E-13,-1.,-1.66321791206623E-16)) ;
#43308=DIRECTION('center_axis',(-1.74838664905478E-13,-0.999847695156391,
0.0174524064372797)) ;
#43309=DIRECTION('ref_axis',(4.84783030058612E-14,0.0174524064372797,0.999847695156391)) ;
#43310=DIRECTION('',(-4.84783030058629E-14,-0.0174524064372897,-0.999847695156391)) ;
#43311=DIRECTION('',(4.84783030057975E-14,0.0174524064369153,0.999847695156398)) ;
#43312=DIRECTION('center_axis',(1.76424026290696E-13,0.999847695156391,
0.01745240643728)) ;
#43313=DIRECTION('ref_axis',(-4.23469899241728E-14,0.01745240643728,-0.999847695156391)) ;
#43314=DIRECTION('',(4.2346989924171E-14,-0.01745240643729,0.999847695156391)) ;
#43315=DIRECTION('',(1.,-1.75658099177411E-13,-4.54195640846217E-14)) ;
#43316=DIRECTION('',(-4.23469899241322E-14,0.0174524064375099,-0.999847695156387)) ;
#43317=DIRECTION('center_axis',(-1.74838664905478E-13,-0.999847695156391,
0.0174524064372797)) ;
#43318=DIRECTION('ref_axis',(4.84783030058612E-14,0.0174524064372797,0.999847695156391)) ;
#43319=DIRECTION('',(4.84783030059014E-14,0.0174524064375096,0.999847695156387)) ;
#43320=DIRECTION('',(-1.,1.75658099177411E-13,4.54195640846217E-14)) ;
#43321=DIRECTION('',(-4.84783030058629E-14,-0.0174524064372897,-0.999847695156391)) ;
#43322=DIRECTION('center_axis',(1.76424026290696E-13,0.999847695156391,
0.01745240643728)) ;
#43323=DIRECTION('ref_axis',(-4.23469899241728E-14,0.01745240643728,-0.999847695156391)) ;
#43324=DIRECTION('',(4.2346989924171E-14,-0.01745240643729,0.999847695156391)) ;
#43325=DIRECTION('',(1.,-1.75658099177411E-13,-4.54195640846217E-14)) ;
#43326=DIRECTION('',(-4.23469899241322E-14,0.0174524064375099,-0.999847695156387)) ;
#43327=DIRECTION('center_axis',(-1.74838664905478E-13,-0.999847695156391,
0.0174524064372797)) ;
#43328=DIRECTION('ref_axis',(4.84783030058612E-14,0.0174524064372797,0.999847695156391)) ;
#43329=DIRECTION('',(4.84783030059014E-14,0.0174524064375096,0.999847695156387)) ;
#43330=DIRECTION('',(-1.,1.75658099177411E-13,4.54195640846217E-14)) ;
#43331=DIRECTION('',(-4.84783030058629E-14,-0.0174524064372897,-0.999847695156391)) ;
#43332=DIRECTION('center_axis',(1.76424026290696E-13,0.999847695156391,
0.01745240643728)) ;
#43333=DIRECTION('ref_axis',(-4.23469899241728E-14,0.01745240643728,-0.999847695156391)) ;
#43334=DIRECTION('',(4.2346989924171E-14,-0.01745240643729,0.999847695156391)) ;
#43335=DIRECTION('',(1.,-1.75658099177411E-13,-4.54195640846217E-14)) ;
#43336=DIRECTION('',(-4.23469899241322E-14,0.0174524064375099,-0.999847695156387)) ;
#43337=DIRECTION('center_axis',(-1.74838664905478E-13,-0.999847695156391,
0.0174524064372797)) ;
#43338=DIRECTION('ref_axis',(4.84783030058612E-14,0.0174524064372797,0.999847695156391)) ;
#43339=DIRECTION('',(4.84783030059014E-14,0.0174524064375096,0.999847695156387)) ;
#43340=DIRECTION('',(-1.,1.75658099177411E-13,4.54195640846217E-14)) ;
#43341=DIRECTION('',(-4.84783030058629E-14,-0.0174524064372897,-0.999847695156391)) ;
#43342=DIRECTION('center_axis',(1.76424026290696E-13,0.999847695156391,
0.01745240643728)) ;
#43343=DIRECTION('ref_axis',(-4.23469899241728E-14,0.01745240643728,-0.999847695156391)) ;
#43344=DIRECTION('',(4.2346989924171E-14,-0.01745240643729,0.999847695156391)) ;
#43345=DIRECTION('',(1.,-1.75658099177411E-13,-4.54195640846217E-14)) ;
#43346=DIRECTION('',(-4.23469899241322E-14,0.0174524064375099,-0.999847695156387)) ;
#43347=DIRECTION('center_axis',(1.74838664905478E-13,0.999847695156391,
-0.0174524064372797)) ;
#43348=DIRECTION('ref_axis',(-4.84783030058612E-14,-0.0174524064372797,
-0.999847695156391)) ;
#43349=DIRECTION('',(4.84783030059014E-14,0.0174524064375096,0.999847695156387)) ;
#43350=DIRECTION('',(-1.,1.75658099177411E-13,4.54195640846217E-14)) ;
#43351=DIRECTION('',(-4.84783030058629E-14,-0.0174524064372897,-0.999847695156391)) ;
#43352=DIRECTION('center_axis',(-1.76424026290696E-13,-0.999847695156391,
-0.01745240643728)) ;
#43353=DIRECTION('ref_axis',(4.23469899241728E-14,-0.01745240643728,0.999847695156391)) ;
#43354=DIRECTION('',(4.2346989924171E-14,-0.01745240643729,0.999847695156391)) ;
#43355=DIRECTION('',(1.,-1.75658099177411E-13,-4.54195640846217E-14)) ;
#43356=DIRECTION('',(-4.23469899241322E-14,0.0174524064375099,-0.999847695156387)) ;
#43357=DIRECTION('center_axis',(1.74838664905478E-13,0.999847695156391,
-0.0174524064372797)) ;
#43358=DIRECTION('ref_axis',(-4.84783030058612E-14,-0.0174524064372797,
-0.999847695156391)) ;
#43359=DIRECTION('',(4.84783030059014E-14,0.0174524064375096,0.999847695156387)) ;
#43360=DIRECTION('',(-1.,1.75658099177411E-13,4.54195640846217E-14)) ;
#43361=DIRECTION('',(-4.84783030058629E-14,-0.0174524064372897,-0.999847695156391)) ;
#43362=DIRECTION('center_axis',(-1.76424026290696E-13,-0.999847695156391,
-0.01745240643728)) ;
#43363=DIRECTION('ref_axis',(4.23469899241728E-14,-0.01745240643728,0.999847695156391)) ;
#43364=DIRECTION('',(4.2346989924171E-14,-0.01745240643729,0.999847695156391)) ;
#43365=DIRECTION('',(1.,-1.75658099177411E-13,-4.54195640846217E-14)) ;
#43366=DIRECTION('',(-4.23469899241322E-14,0.0174524064375099,-0.999847695156387)) ;
#43367=DIRECTION('center_axis',(1.74838664905478E-13,0.999847695156391,
-0.0174524064372797)) ;
#43368=DIRECTION('ref_axis',(-4.84783030058612E-14,-0.0174524064372797,
-0.999847695156391)) ;
#43369=DIRECTION('',(4.84783030059031E-14,0.0174524064375196,0.999847695156387)) ;
#43370=DIRECTION('',(-1.,1.75658099177411E-13,4.54195640846217E-14)) ;
#43371=DIRECTION('',(-4.84783030058629E-14,-0.0174524064372897,-0.999847695156391)) ;
#43372=DIRECTION('center_axis',(-1.76424026290696E-13,-0.999847695156391,
-0.01745240643728)) ;
#43373=DIRECTION('ref_axis',(4.23469899241728E-14,-0.01745240643728,0.999847695156391)) ;
#43374=DIRECTION('',(4.2346989924171E-14,-0.01745240643729,0.999847695156391)) ;
#43375=DIRECTION('',(1.,-1.75658099177411E-13,-4.54195640846217E-14)) ;
#43376=DIRECTION('',(-4.23469899241322E-14,0.0174524064375099,-0.999847695156387)) ;
#43377=DIRECTION('center_axis',(1.74838664905478E-13,0.999847695156391,
-0.0174524064372797)) ;
#43378=DIRECTION('ref_axis',(-4.84783030058612E-14,-0.0174524064372797,
-0.999847695156391)) ;
#43379=DIRECTION('',(4.84783030059014E-14,0.0174524064375096,0.999847695156387)) ;
#43380=DIRECTION('',(-1.,1.75658099177411E-13,4.54195640846217E-14)) ;
#43381=DIRECTION('',(-4.84783030058629E-14,-0.0174524064372897,-0.999847695156391)) ;
#43382=DIRECTION('center_axis',(-1.76424026290696E-13,-0.999847695156391,
-0.01745240643728)) ;
#43383=DIRECTION('ref_axis',(4.23469899241728E-14,-0.01745240643728,0.999847695156391)) ;
#43384=DIRECTION('',(4.2346989924171E-14,-0.01745240643729,0.999847695156391)) ;
#43385=DIRECTION('',(1.,-1.75658099177411E-13,-4.54195640846217E-14)) ;
#43386=DIRECTION('',(-4.23469899241322E-14,0.0174524064375099,-0.999847695156387)) ;
#43387=DIRECTION('center_axis',(1.74838664905478E-13,0.999847695156391,
-0.0174524064372797)) ;
#43388=DIRECTION('ref_axis',(-4.84783030058612E-14,-0.0174524064372797,
-0.999847695156391)) ;
#43389=DIRECTION('',(4.84783030059049E-14,0.0174524064375296,0.999847695156387)) ;
#43390=DIRECTION('',(-1.,1.75658099177411E-13,4.54195640846217E-14)) ;
#43391=DIRECTION('',(-4.84783030058647E-14,-0.0174524064372997,-0.999847695156391)) ;
#43392=DIRECTION('center_axis',(-1.,1.75658099177411E-13,4.54195640846217E-14)) ;
#43393=DIRECTION('ref_axis',(-1.75658099177411E-13,-1.,6.26847853931514E-43)) ;
#43394=DIRECTION('center_axis',(-1.,1.73688224296914E-13,4.53957858957841E-14)) ;
#43395=DIRECTION('ref_axis',(4.53957858957841E-14,2.00890147845606E-41,
1.)) ;
#43396=DIRECTION('',(-4.2346989924355E-14,0.0174524064362477,-0.999847695156409)) ;
#43397=DIRECTION('center_axis',(-1.,1.75658099177411E-13,4.54195640846217E-14)) ;
#43398=DIRECTION('ref_axis',(-1.75658099177411E-13,-1.,6.26847853931514E-43)) ;
#43399=DIRECTION('',(1.75658099177411E-13,1.,1.66321791206623E-16)) ;
#43400=DIRECTION('center_axis',(-1.,1.75658099177411E-13,4.54195640846217E-14)) ;
#43401=DIRECTION('ref_axis',(-1.75658099177411E-13,-1.,6.26847853931514E-43)) ;
#43402=DIRECTION('',(1.75658099177411E-13,1.,1.66321791206623E-16)) ;
#43403=DIRECTION('center_axis',(-1.,1.75658099177411E-13,4.54195640846217E-14)) ;
#43404=DIRECTION('ref_axis',(-1.75658099177411E-13,-1.,6.26847853931514E-43)) ;
#43405=DIRECTION('',(1.75658099177411E-13,1.,1.66321791206623E-16)) ;
#43406=DIRECTION('center_axis',(-1.,1.75658099177411E-13,4.54195640846217E-14)) ;
#43407=DIRECTION('ref_axis',(-1.75658099177411E-13,-1.,6.26847853931514E-43)) ;
#43408=DIRECTION('',(1.75658099177411E-13,1.,1.66321791206623E-16)) ;
#43409=DIRECTION('center_axis',(-1.,1.75658099177411E-13,4.54195640846217E-14)) ;
#43410=DIRECTION('ref_axis',(-1.75658099177411E-13,-1.,6.26847853931514E-43)) ;
#43411=DIRECTION('',(1.75658099177411E-13,1.,1.66321791206623E-16)) ;
#43412=DIRECTION('center_axis',(-1.,1.75658099177411E-13,4.54195640846217E-14)) ;
#43413=DIRECTION('ref_axis',(-1.75658099177411E-13,-1.,6.26847853931514E-43)) ;
#43414=DIRECTION('',(1.75658099177411E-13,1.,1.66321791206623E-16)) ;
#43415=DIRECTION('center_axis',(-1.,1.75658099177411E-13,4.54195640846217E-14)) ;
#43416=DIRECTION('ref_axis',(-1.75658099177411E-13,-1.,6.26847853931514E-43)) ;
#43417=DIRECTION('',(1.75658099177411E-13,1.,1.66321791206623E-16)) ;
#43418=DIRECTION('center_axis',(-1.,1.75658099177411E-13,4.54195640846217E-14)) ;
#43419=DIRECTION('ref_axis',(-1.75658099177411E-13,-1.,6.26847853931514E-43)) ;
#43420=DIRECTION('',(1.75658099177411E-13,1.,1.66321791206623E-16)) ;
#43421=DIRECTION('center_axis',(4.54195640846217E-14,-1.66321791214601E-16,
1.)) ;
#43422=DIRECTION('ref_axis',(1.75658099177411E-13,1.,1.66321791206623E-16)) ;
#43423=DIRECTION('center_axis',(-2.16239769233719E-14,8.31608956071042E-17,
-1.)) ;
#43424=DIRECTION('ref_axis',(1.,-9.64599832246215E-47,-2.16239769233719E-14)) ;
#43425=DIRECTION('center_axis',(-2.17161023787787E-15,3.92492613217813E-28,
1.)) ;
#43426=DIRECTION('ref_axis',(1.,-1.46338648716481E-13,2.28654138619502E-15)) ;
#43427=DIRECTION('center_axis',(-2.17161023787787E-15,3.92492613217813E-28,
1.)) ;
#43428=DIRECTION('ref_axis',(-1.,4.92531066966514E-14,-2.17161023787787E-15)) ;
#43429=DIRECTION('center_axis',(-2.17161023787787E-15,3.92492613217813E-28,
1.)) ;
#43430=DIRECTION('ref_axis',(-1.,4.92531066966514E-14,-2.17161023787787E-15)) ;
#43431=DIRECTION('center_axis',(-1.37192483171701E-13,-1.,9.45640122022591E-29)) ;
#43432=DIRECTION('ref_axis',(-1.,1.37192483171701E-13,-2.85817673274378E-15)) ;
#43433=DIRECTION('center_axis',(-2.1716102378779E-15,3.83815143260386E-28,
1.)) ;
#43434=DIRECTION('ref_axis',(-1.,-9.69015809248849E-15,-2.1716102378779E-15)) ;
#43435=DIRECTION('center_axis',(2.1716102378779E-15,-3.83815143260386E-28,
-1.)) ;
#43436=DIRECTION('ref_axis',(-1.,-7.3303373675338E-16,-2.1716102378779E-15)) ;
#43437=DIRECTION('',(-2.1716102378779E-15,3.83815143260386E-28,1.)) ;
#43438=DIRECTION('center_axis',(2.1716102378779E-15,-3.83815143260386E-28,
-1.)) ;
#43439=DIRECTION('ref_axis',(-1.,1.59141680100251E-13,-2.48658875156642E-15)) ;
#43440=DIRECTION('center_axis',(1.49195325093984E-13,1.,-5.98210478427684E-29)) ;
#43441=DIRECTION('ref_axis',(1.,-1.49195325093984E-13,1.554117969729E-15)) ;
#43442=DIRECTION('center_axis',(-1.66533453692587E-16,-1.,3.82991969484897E-28)) ;
#43443=DIRECTION('ref_axis',(2.1716102378779E-15,-3.83353615237885E-28,
-1.)) ;
#43444=DIRECTION('',(-2.17161023787787E-15,3.83420712807771E-28,1.)) ;
#43445=DIRECTION('center_axis',(2.17161023787787E-15,-3.83420712807771E-28,
-1.)) ;
#43446=DIRECTION('ref_axis',(-0.707106781186552,-0.707106781186543,-1.53556032529731E-15)) ;
#43447=DIRECTION('center_axis',(4.54195640846217E-14,-1.66321791214601E-16,
1.)) ;
#43448=DIRECTION('ref_axis',(1.75658099177411E-13,1.,1.66321791206623E-16)) ;
#43449=DIRECTION('center_axis',(-2.16239769233719E-14,8.31608956071042E-17,
-1.)) ;
#43450=DIRECTION('ref_axis',(1.,-9.64599832246215E-47,-2.16239769233719E-14)) ;
#43451=DIRECTION('center_axis',(-2.17161023787787E-15,3.92492613217813E-28,
1.)) ;
#43452=DIRECTION('ref_axis',(1.,-1.46338648716481E-13,2.28654138619502E-15)) ;
#43453=DIRECTION('center_axis',(-2.17161023787787E-15,3.92492613217813E-28,
1.)) ;
#43454=DIRECTION('ref_axis',(-1.,4.92531066966514E-14,-2.17161023787787E-15)) ;
#43455=DIRECTION('center_axis',(-2.17161023787787E-15,3.92492613217813E-28,
1.)) ;
#43456=DIRECTION('ref_axis',(-1.,4.92531066966514E-14,-2.17161023787787E-15)) ;
#43457=DIRECTION('center_axis',(-1.37192483171701E-13,-1.,9.45640122022591E-29)) ;
#43458=DIRECTION('ref_axis',(-1.,1.37192483171701E-13,-2.85817673274378E-15)) ;
#43459=DIRECTION('center_axis',(-2.1716102378779E-15,3.83815143260386E-28,
1.)) ;
#43460=DIRECTION('ref_axis',(-1.,-9.69015809248849E-15,-2.1716102378779E-15)) ;
#43461=DIRECTION('center_axis',(2.1716102378779E-15,-3.83815143260386E-28,
-1.)) ;
#43462=DIRECTION('ref_axis',(-1.,-7.3303373675338E-16,-2.1716102378779E-15)) ;
#43463=DIRECTION('',(-2.1716102378779E-15,3.83815143260386E-28,1.)) ;
#43464=DIRECTION('center_axis',(2.1716102378779E-15,-3.83815143260386E-28,
-1.)) ;
#43465=DIRECTION('ref_axis',(-1.,1.59141680100251E-13,-2.48658875156642E-15)) ;
#43466=DIRECTION('center_axis',(1.49195325093984E-13,1.,-5.98210478427684E-29)) ;
#43467=DIRECTION('ref_axis',(1.,-1.49195325093984E-13,1.554117969729E-15)) ;
#43468=DIRECTION('center_axis',(-1.66533453692587E-16,-1.,3.82991969484897E-28)) ;
#43469=DIRECTION('ref_axis',(2.1716102378779E-15,-3.83353615237885E-28,
-1.)) ;
#43470=DIRECTION('',(-2.17161023787787E-15,3.83420712807771E-28,1.)) ;
#43471=DIRECTION('center_axis',(2.17161023787787E-15,-3.83420712807771E-28,
-1.)) ;
#43472=DIRECTION('ref_axis',(-0.707106781186552,-0.707106781186543,-1.53556032529731E-15)) ;
#43473=DIRECTION('center_axis',(4.54195640846217E-14,-1.66321791214601E-16,
1.)) ;
#43474=DIRECTION('ref_axis',(1.75658099177411E-13,1.,1.66321791206623E-16)) ;
#43475=DIRECTION('center_axis',(-2.16239769233719E-14,8.31608956071042E-17,
-1.)) ;
#43476=DIRECTION('ref_axis',(1.,-9.64599832246215E-47,-2.16239769233719E-14)) ;
#43477=DIRECTION('center_axis',(-2.17161023787787E-15,3.92492613217813E-28,
1.)) ;
#43478=DIRECTION('ref_axis',(1.,-1.46338648716481E-13,2.28654138619502E-15)) ;
#43479=DIRECTION('center_axis',(-2.17161023787787E-15,3.92492613217813E-28,
1.)) ;
#43480=DIRECTION('ref_axis',(-1.,4.92531066966514E-14,-2.17161023787787E-15)) ;
#43481=DIRECTION('center_axis',(-2.17161023787787E-15,3.92492613217813E-28,
1.)) ;
#43482=DIRECTION('ref_axis',(-1.,4.92531066966514E-14,-2.17161023787787E-15)) ;
#43483=DIRECTION('center_axis',(-1.37192483171701E-13,-1.,9.45640122022591E-29)) ;
#43484=DIRECTION('ref_axis',(-1.,1.37192483171701E-13,-2.85817673274378E-15)) ;
#43485=DIRECTION('center_axis',(-2.1716102378779E-15,3.83815143260386E-28,
1.)) ;
#43486=DIRECTION('ref_axis',(-1.,-9.69015809248849E-15,-2.1716102378779E-15)) ;
#43487=DIRECTION('center_axis',(2.1716102378779E-15,-3.83815143260386E-28,
-1.)) ;
#43488=DIRECTION('ref_axis',(-1.,-7.3303373675338E-16,-2.1716102378779E-15)) ;
#43489=DIRECTION('',(-2.1716102378779E-15,3.83815143260386E-28,1.)) ;
#43490=DIRECTION('center_axis',(2.1716102378779E-15,-3.83815143260386E-28,
-1.)) ;
#43491=DIRECTION('ref_axis',(-1.,1.59141680100251E-13,-2.48658875156642E-15)) ;
#43492=DIRECTION('center_axis',(1.49195325093984E-13,1.,-5.98210478427684E-29)) ;
#43493=DIRECTION('ref_axis',(1.,-1.49195325093984E-13,1.554117969729E-15)) ;
#43494=DIRECTION('center_axis',(-1.66533453692587E-16,-1.,3.82991969484897E-28)) ;
#43495=DIRECTION('ref_axis',(2.1716102378779E-15,-3.83353615237885E-28,
-1.)) ;
#43496=DIRECTION('',(-2.17161023787787E-15,3.83420712807771E-28,1.)) ;
#43497=DIRECTION('center_axis',(2.17161023787787E-15,-3.83420712807771E-28,
-1.)) ;
#43498=DIRECTION('ref_axis',(-0.707106781186552,-0.707106781186543,-1.53556032529731E-15)) ;
#43499=DIRECTION('center_axis',(4.54195640846217E-14,-1.66321791214601E-16,
1.)) ;
#43500=DIRECTION('ref_axis',(1.75658099177411E-13,1.,1.66321791206623E-16)) ;
#43501=DIRECTION('center_axis',(-2.16239769233719E-14,8.31608956071042E-17,
-1.)) ;
#43502=DIRECTION('ref_axis',(1.,-9.64599832246215E-47,-2.16239769233719E-14)) ;
#43503=DIRECTION('center_axis',(-2.17161023787787E-15,3.92492613217813E-28,
1.)) ;
#43504=DIRECTION('ref_axis',(1.,-1.46338648716481E-13,2.28654138619502E-15)) ;
#43505=DIRECTION('center_axis',(-2.17161023787787E-15,3.92492613217813E-28,
1.)) ;
#43506=DIRECTION('ref_axis',(-1.,4.92531066966514E-14,-2.17161023787787E-15)) ;
#43507=DIRECTION('center_axis',(-2.17161023787787E-15,3.92492613217813E-28,
1.)) ;
#43508=DIRECTION('ref_axis',(-1.,4.92531066966514E-14,-2.17161023787787E-15)) ;
#43509=DIRECTION('center_axis',(-1.37192483171701E-13,-1.,9.45640122022591E-29)) ;
#43510=DIRECTION('ref_axis',(-1.,1.37192483171701E-13,-2.85817673274378E-15)) ;
#43511=DIRECTION('center_axis',(-2.1716102378779E-15,3.83815143260386E-28,
1.)) ;
#43512=DIRECTION('ref_axis',(-1.,-9.69015809248849E-15,-2.1716102378779E-15)) ;
#43513=DIRECTION('center_axis',(2.1716102378779E-15,-3.83815143260386E-28,
-1.)) ;
#43514=DIRECTION('ref_axis',(-1.,-7.3303373675338E-16,-2.1716102378779E-15)) ;
#43515=DIRECTION('',(-2.1716102378779E-15,3.83815143260386E-28,1.)) ;
#43516=DIRECTION('center_axis',(2.1716102378779E-15,-3.83815143260386E-28,
-1.)) ;
#43517=DIRECTION('ref_axis',(-1.,1.59141680100251E-13,-2.48658875156642E-15)) ;
#43518=DIRECTION('center_axis',(1.49195325093984E-13,1.,-5.98210478427684E-29)) ;
#43519=DIRECTION('ref_axis',(1.,-1.49195325093984E-13,1.554117969729E-15)) ;
#43520=DIRECTION('center_axis',(-1.66533453692587E-16,-1.,3.82991969484897E-28)) ;
#43521=DIRECTION('ref_axis',(2.1716102378779E-15,-3.83353615237885E-28,
-1.)) ;
#43522=DIRECTION('',(-2.17161023787787E-15,3.83420712807771E-28,1.)) ;
#43523=DIRECTION('center_axis',(2.17161023787787E-15,-3.83420712807771E-28,
-1.)) ;
#43524=DIRECTION('ref_axis',(-0.707106781186552,-0.707106781186543,-1.53556032529731E-15)) ;
#43525=DIRECTION('center_axis',(4.54195640846217E-14,-1.66321791214601E-16,
1.)) ;
#43526=DIRECTION('ref_axis',(1.75658099177411E-13,1.,1.66321791206623E-16)) ;
#43527=DIRECTION('center_axis',(-2.16239769233719E-14,8.31608956071042E-17,
-1.)) ;
#43528=DIRECTION('ref_axis',(1.,-9.64599832246215E-47,-2.16239769233719E-14)) ;
#43529=DIRECTION('center_axis',(-2.17161023787787E-15,3.92492613217813E-28,
1.)) ;
#43530=DIRECTION('ref_axis',(1.,-1.46338648716481E-13,2.28654138619502E-15)) ;
#43531=DIRECTION('center_axis',(-2.17161023787787E-15,3.92492613217813E-28,
1.)) ;
#43532=DIRECTION('ref_axis',(-1.,4.92531066966514E-14,-2.17161023787787E-15)) ;
#43533=DIRECTION('center_axis',(-2.17161023787787E-15,3.92492613217813E-28,
1.)) ;
#43534=DIRECTION('ref_axis',(-1.,4.92531066966514E-14,-2.17161023787787E-15)) ;
#43535=DIRECTION('center_axis',(-1.37192483171701E-13,-1.,9.45640122022591E-29)) ;
#43536=DIRECTION('ref_axis',(-1.,1.37192483171701E-13,-2.85817673274378E-15)) ;
#43537=DIRECTION('center_axis',(-2.1716102378779E-15,3.83815143260386E-28,
1.)) ;
#43538=DIRECTION('ref_axis',(-1.,-9.69015809248849E-15,-2.1716102378779E-15)) ;
#43539=DIRECTION('center_axis',(2.1716102378779E-15,-3.83815143260386E-28,
-1.)) ;
#43540=DIRECTION('ref_axis',(-1.,-7.3303373675338E-16,-2.1716102378779E-15)) ;
#43541=DIRECTION('',(-2.1716102378779E-15,3.83815143260386E-28,1.)) ;
#43542=DIRECTION('center_axis',(2.1716102378779E-15,-3.83815143260386E-28,
-1.)) ;
#43543=DIRECTION('ref_axis',(-1.,1.59141680100251E-13,-2.48658875156642E-15)) ;
#43544=DIRECTION('center_axis',(1.49195325093984E-13,1.,-5.98210478427684E-29)) ;
#43545=DIRECTION('ref_axis',(1.,-1.49195325093984E-13,1.554117969729E-15)) ;
#43546=DIRECTION('center_axis',(-1.66533453692587E-16,-1.,3.82991969484897E-28)) ;
#43547=DIRECTION('ref_axis',(2.1716102378779E-15,-3.83353615237885E-28,
-1.)) ;
#43548=DIRECTION('',(-2.17161023787787E-15,3.83420712807771E-28,1.)) ;
#43549=DIRECTION('center_axis',(2.17161023787787E-15,-3.83420712807771E-28,
-1.)) ;
#43550=DIRECTION('ref_axis',(-0.707106781186552,-0.707106781186543,-1.53556032529731E-15)) ;
#43551=DIRECTION('center_axis',(4.54195640846217E-14,-1.66321791214601E-16,
1.)) ;
#43552=DIRECTION('ref_axis',(1.75658099177411E-13,1.,1.66321791206623E-16)) ;
#43553=DIRECTION('center_axis',(-2.16239769233719E-14,8.31608956071042E-17,
-1.)) ;
#43554=DIRECTION('ref_axis',(1.,-9.64599832246215E-47,-2.16239769233719E-14)) ;
#43555=DIRECTION('center_axis',(-2.17161023787787E-15,3.92492613217813E-28,
1.)) ;
#43556=DIRECTION('ref_axis',(1.,-1.46338648716481E-13,2.28654138619502E-15)) ;
#43557=DIRECTION('center_axis',(-2.17161023787787E-15,3.92492613217813E-28,
1.)) ;
#43558=DIRECTION('ref_axis',(-1.,4.92531066966514E-14,-2.17161023787787E-15)) ;
#43559=DIRECTION('center_axis',(-2.17161023787787E-15,3.92492613217813E-28,
1.)) ;
#43560=DIRECTION('ref_axis',(-1.,4.92531066966514E-14,-2.17161023787787E-15)) ;
#43561=DIRECTION('center_axis',(-1.37192483171701E-13,-1.,9.45640122022591E-29)) ;
#43562=DIRECTION('ref_axis',(-1.,1.37192483171701E-13,-2.85817673274378E-15)) ;
#43563=DIRECTION('center_axis',(-2.1716102378779E-15,3.83815143260386E-28,
1.)) ;
#43564=DIRECTION('ref_axis',(-1.,-9.69015809248849E-15,-2.1716102378779E-15)) ;
#43565=DIRECTION('center_axis',(2.1716102378779E-15,-3.83815143260386E-28,
-1.)) ;
#43566=DIRECTION('ref_axis',(-1.,-7.3303373675338E-16,-2.1716102378779E-15)) ;
#43567=DIRECTION('',(-2.1716102378779E-15,3.83815143260386E-28,1.)) ;
#43568=DIRECTION('center_axis',(2.1716102378779E-15,-3.83815143260386E-28,
-1.)) ;
#43569=DIRECTION('ref_axis',(-1.,1.59141680100251E-13,-2.48658875156642E-15)) ;
#43570=DIRECTION('center_axis',(1.49195325093984E-13,1.,-5.98210478427684E-29)) ;
#43571=DIRECTION('ref_axis',(1.,-1.49195325093984E-13,1.554117969729E-15)) ;
#43572=DIRECTION('center_axis',(-1.66533453692587E-16,-1.,3.82991969484897E-28)) ;
#43573=DIRECTION('ref_axis',(2.1716102378779E-15,-3.83353615237885E-28,
-1.)) ;
#43574=DIRECTION('',(-2.17161023787787E-15,3.83420712807771E-28,1.)) ;
#43575=DIRECTION('center_axis',(2.17161023787787E-15,-3.83420712807771E-28,
-1.)) ;
#43576=DIRECTION('ref_axis',(-0.707106781186552,-0.707106781186543,-1.53556032529731E-15)) ;
#43577=DIRECTION('center_axis',(4.54195640846217E-14,-1.66321791214601E-16,
1.)) ;
#43578=DIRECTION('ref_axis',(1.75658099177411E-13,1.,1.66321791206623E-16)) ;
#43579=DIRECTION('center_axis',(-2.16239769233719E-14,8.31608956071042E-17,
-1.)) ;
#43580=DIRECTION('ref_axis',(1.,-9.64599832246215E-47,-2.16239769233719E-14)) ;
#43581=DIRECTION('center_axis',(-2.17161023787787E-15,3.92492613217813E-28,
1.)) ;
#43582=DIRECTION('ref_axis',(1.,-1.46338648716481E-13,2.28654138619502E-15)) ;
#43583=DIRECTION('center_axis',(-2.17161023787787E-15,3.92492613217813E-28,
1.)) ;
#43584=DIRECTION('ref_axis',(-1.,4.92531066966514E-14,-2.17161023787787E-15)) ;
#43585=DIRECTION('center_axis',(-2.17161023787787E-15,3.92492613217813E-28,
1.)) ;
#43586=DIRECTION('ref_axis',(-1.,4.92531066966514E-14,-2.17161023787787E-15)) ;
#43587=DIRECTION('center_axis',(-1.37192483171701E-13,-1.,9.45640122022591E-29)) ;
#43588=DIRECTION('ref_axis',(-1.,1.37192483171701E-13,-2.85817673274378E-15)) ;
#43589=DIRECTION('center_axis',(-2.1716102378779E-15,3.83815143260386E-28,
1.)) ;
#43590=DIRECTION('ref_axis',(-1.,-9.69015809248849E-15,-2.1716102378779E-15)) ;
#43591=DIRECTION('center_axis',(2.1716102378779E-15,-3.83815143260386E-28,
-1.)) ;
#43592=DIRECTION('ref_axis',(-1.,-7.3303373675338E-16,-2.1716102378779E-15)) ;
#43593=DIRECTION('',(-2.1716102378779E-15,3.83815143260386E-28,1.)) ;
#43594=DIRECTION('center_axis',(2.1716102378779E-15,-3.83815143260386E-28,
-1.)) ;
#43595=DIRECTION('ref_axis',(-1.,1.59141680100251E-13,-2.48658875156642E-15)) ;
#43596=DIRECTION('center_axis',(1.49195325093984E-13,1.,-5.98210478427684E-29)) ;
#43597=DIRECTION('ref_axis',(1.,-1.49195325093984E-13,1.554117969729E-15)) ;
#43598=DIRECTION('center_axis',(-1.66533453692587E-16,-1.,3.82991969484897E-28)) ;
#43599=DIRECTION('ref_axis',(2.1716102378779E-15,-3.83353615237885E-28,
-1.)) ;
#43600=DIRECTION('',(-2.17161023787787E-15,3.83420712807771E-28,1.)) ;
#43601=DIRECTION('center_axis',(2.17161023787787E-15,-3.83420712807771E-28,
-1.)) ;
#43602=DIRECTION('ref_axis',(-0.707106781186552,-0.707106781186543,-1.53556032529731E-15)) ;
#43603=DIRECTION('center_axis',(4.54195640846217E-14,-1.66321791214601E-16,
1.)) ;
#43604=DIRECTION('ref_axis',(1.75658099177411E-13,1.,1.66321791206623E-16)) ;
#43605=DIRECTION('center_axis',(-2.16239769233719E-14,8.31608956071042E-17,
-1.)) ;
#43606=DIRECTION('ref_axis',(1.,-9.64599832246215E-47,-2.16239769233719E-14)) ;
#43607=DIRECTION('center_axis',(-2.17161023787787E-15,3.92492613217813E-28,
1.)) ;
#43608=DIRECTION('ref_axis',(1.,-1.46338648716481E-13,2.28654138619502E-15)) ;
#43609=DIRECTION('center_axis',(-2.17161023787787E-15,3.92492613217813E-28,
1.)) ;
#43610=DIRECTION('ref_axis',(-1.,4.92531066966514E-14,-2.17161023787787E-15)) ;
#43611=DIRECTION('center_axis',(-2.17161023787787E-15,3.92492613217813E-28,
1.)) ;
#43612=DIRECTION('ref_axis',(-1.,4.92531066966514E-14,-2.17161023787787E-15)) ;
#43613=DIRECTION('center_axis',(-1.37192483171701E-13,-1.,9.45640122022591E-29)) ;
#43614=DIRECTION('ref_axis',(-1.,1.37192483171701E-13,-2.85817673274378E-15)) ;
#43615=DIRECTION('center_axis',(-2.1716102378779E-15,3.83815143260386E-28,
1.)) ;
#43616=DIRECTION('ref_axis',(-1.,-9.69015809248849E-15,-2.1716102378779E-15)) ;
#43617=DIRECTION('center_axis',(2.1716102378779E-15,-3.83815143260386E-28,
-1.)) ;
#43618=DIRECTION('ref_axis',(-1.,-7.3303373675338E-16,-2.1716102378779E-15)) ;
#43619=DIRECTION('',(-2.1716102378779E-15,3.83815143260386E-28,1.)) ;
#43620=DIRECTION('center_axis',(2.1716102378779E-15,-3.83815143260386E-28,
-1.)) ;
#43621=DIRECTION('ref_axis',(-1.,1.59141680100251E-13,-2.48658875156642E-15)) ;
#43622=DIRECTION('center_axis',(1.49195325093984E-13,1.,-5.98210478427684E-29)) ;
#43623=DIRECTION('ref_axis',(1.,-1.49195325093984E-13,1.554117969729E-15)) ;
#43624=DIRECTION('center_axis',(-1.66533453692587E-16,-1.,3.82991969484897E-28)) ;
#43625=DIRECTION('ref_axis',(2.1716102378779E-15,-3.83353615237885E-28,
-1.)) ;
#43626=DIRECTION('',(-2.17161023787787E-15,3.83420712807771E-28,1.)) ;
#43627=DIRECTION('center_axis',(2.17161023787787E-15,-3.83420712807771E-28,
-1.)) ;
#43628=DIRECTION('ref_axis',(-0.707106781186552,-0.707106781186543,-1.53556032529731E-15)) ;
#43629=DIRECTION('center_axis',(-2.17161023787787E-15,3.92492613217813E-28,
1.)) ;
#43630=DIRECTION('ref_axis',(1.,-1.46338648716481E-13,2.28654138619502E-15)) ;
#43631=DIRECTION('center_axis',(-2.17161023787787E-15,3.92492613217813E-28,
1.)) ;
#43632=DIRECTION('ref_axis',(-1.,4.92531066966514E-14,-2.17161023787787E-15)) ;
#43633=DIRECTION('center_axis',(-2.17161023787787E-15,3.92492613217813E-28,
1.)) ;
#43634=DIRECTION('ref_axis',(-1.,4.92531066966514E-14,-2.17161023787787E-15)) ;
#43635=DIRECTION('center_axis',(-1.37192483171701E-13,-1.,9.45640122022591E-29)) ;
#43636=DIRECTION('ref_axis',(-1.,1.37192483171701E-13,-2.85817673274378E-15)) ;
#43637=DIRECTION('center_axis',(-2.1716102378779E-15,3.83815143260386E-28,
1.)) ;
#43638=DIRECTION('ref_axis',(-1.,-9.69015809248849E-15,-2.1716102378779E-15)) ;
#43639=DIRECTION('center_axis',(2.1716102378779E-15,-3.83815143260386E-28,
-1.)) ;
#43640=DIRECTION('ref_axis',(-1.,-7.3303373675338E-16,-2.1716102378779E-15)) ;
#43641=DIRECTION('',(-2.1716102378779E-15,3.83815143260386E-28,1.)) ;
#43642=DIRECTION('center_axis',(2.1716102378779E-15,-3.83815143260386E-28,
-1.)) ;
#43643=DIRECTION('ref_axis',(-1.,1.59141680100251E-13,-2.48658875156642E-15)) ;
#43644=DIRECTION('center_axis',(1.49195325093984E-13,1.,-5.98210478427684E-29)) ;
#43645=DIRECTION('ref_axis',(1.,-1.49195325093984E-13,1.554117969729E-15)) ;
#43646=DIRECTION('center_axis',(-1.76424026290696E-13,-0.999847695156391,
-0.01745240643728)) ;
#43647=DIRECTION('ref_axis',(4.23469899241728E-14,-0.01745240643728,0.999847695156391)) ;
#43648=DIRECTION('',(4.23469899241728E-14,-0.01745240643728,0.999847695156391)) ;
#43649=DIRECTION('center_axis',(1.,-1.75658099177411E-13,-4.54195640846217E-14)) ;
#43650=DIRECTION('ref_axis',(-4.54195640846217E-14,1.66321791214601E-16,
-1.)) ;
#43651=DIRECTION('center_axis',(-2.1716102378779E-15,3.83815143260386E-28,
1.)) ;
#43652=DIRECTION('ref_axis',(-0.707106781186643,0.707106781186452,-1.53556032529807E-15)) ;
#43653=DIRECTION('',(-2.1716102378779E-15,3.83815143260386E-28,1.)) ;
#43654=DIRECTION('center_axis',(-1.,1.66533453692966E-16,-2.1716102378779E-15)) ;
#43655=DIRECTION('ref_axis',(1.66533453692966E-16,1.,-3.82783884128008E-28)) ;
#43656=DIRECTION('',(2.1716102378779E-15,-3.83420712807775E-28,-1.)) ;
#43657=DIRECTION('center_axis',(2.1716102378779E-15,-3.83420712807775E-28,
-1.)) ;
#43658=DIRECTION('ref_axis',(-0.707106781186452,-0.707106781186643,-1.53556032529712E-15)) ;
#43659=DIRECTION('',(-2.1716102378779E-15,3.83420712807775E-28,1.)) ;
#43660=DIRECTION('center_axis',(-1.66533453692587E-16,-1.,3.82991969484897E-28)) ;
#43661=DIRECTION('ref_axis',(2.1716102378779E-15,-3.83353615237885E-28,
-1.)) ;
#43662=DIRECTION('center_axis',(-2.17161023787787E-15,3.83815143260382E-28,
1.)) ;
#43663=DIRECTION('ref_axis',(-0.707106781186643,0.707106781186452,-1.53556032529805E-15)) ;
#43664=DIRECTION('center_axis',(-2.1716102378779E-15,3.83815143260386E-28,
1.)) ;
#43665=DIRECTION('ref_axis',(-0.707106781186643,0.707106781186452,-1.53556032529807E-15)) ;
#43666=DIRECTION('',(-2.1716102378779E-15,3.83815143260386E-28,1.)) ;
#43667=DIRECTION('center_axis',(-1.,1.66533453692966E-16,-2.1716102378779E-15)) ;
#43668=DIRECTION('ref_axis',(1.66533453692966E-16,1.,-3.82783884128008E-28)) ;
#43669=DIRECTION('',(2.1716102378779E-15,-3.83420712807775E-28,-1.)) ;
#43670=DIRECTION('center_axis',(2.1716102378779E-15,-3.83420712807775E-28,
-1.)) ;
#43671=DIRECTION('ref_axis',(-0.707106781186452,-0.707106781186643,-1.53556032529712E-15)) ;
#43672=DIRECTION('',(-2.1716102378779E-15,3.83420712807775E-28,1.)) ;
#43673=DIRECTION('center_axis',(-1.66533453692587E-16,-1.,3.82991969484897E-28)) ;
#43674=DIRECTION('ref_axis',(2.1716102378779E-15,-3.83353615237885E-28,
-1.)) ;
#43675=DIRECTION('center_axis',(-2.17161023787787E-15,3.83815143260382E-28,
1.)) ;
#43676=DIRECTION('ref_axis',(-0.707106781186643,0.707106781186452,-1.53556032529805E-15)) ;
#43677=DIRECTION('center_axis',(-2.1716102378779E-15,3.83815143260386E-28,
1.)) ;
#43678=DIRECTION('ref_axis',(-0.707106781186643,0.707106781186452,-1.53556032529807E-15)) ;
#43679=DIRECTION('',(-2.1716102378779E-15,3.83815143260386E-28,1.)) ;
#43680=DIRECTION('center_axis',(-1.,1.66533453692966E-16,-2.1716102378779E-15)) ;
#43681=DIRECTION('ref_axis',(1.66533453692966E-16,1.,-3.82783884128008E-28)) ;
#43682=DIRECTION('',(2.1716102378779E-15,-3.83420712807775E-28,-1.)) ;
#43683=DIRECTION('center_axis',(2.1716102378779E-15,-3.83420712807775E-28,
-1.)) ;
#43684=DIRECTION('ref_axis',(-0.707106781186452,-0.707106781186643,-1.53556032529712E-15)) ;
#43685=DIRECTION('',(-2.1716102378779E-15,3.83420712807775E-28,1.)) ;
#43686=DIRECTION('center_axis',(-1.66533453692587E-16,-1.,3.82991969484897E-28)) ;
#43687=DIRECTION('ref_axis',(2.1716102378779E-15,-3.83353615237885E-28,
-1.)) ;
#43688=DIRECTION('center_axis',(-2.17161023787787E-15,3.83815143260382E-28,
1.)) ;
#43689=DIRECTION('ref_axis',(-0.707106781186643,0.707106781186452,-1.53556032529805E-15)) ;
#43690=DIRECTION('center_axis',(-2.1716102378779E-15,3.83815143260386E-28,
1.)) ;
#43691=DIRECTION('ref_axis',(-0.707106781186643,0.707106781186452,-1.53556032529807E-15)) ;
#43692=DIRECTION('',(-2.1716102378779E-15,3.83815143260386E-28,1.)) ;
#43693=DIRECTION('center_axis',(-1.,1.66533453692966E-16,-2.1716102378779E-15)) ;
#43694=DIRECTION('ref_axis',(1.66533453692966E-16,1.,-3.82783884128008E-28)) ;
#43695=DIRECTION('',(2.1716102378779E-15,-3.83420712807775E-28,-1.)) ;
#43696=DIRECTION('center_axis',(2.1716102378779E-15,-3.83420712807775E-28,
-1.)) ;
#43697=DIRECTION('ref_axis',(-0.707106781186452,-0.707106781186643,-1.53556032529712E-15)) ;
#43698=DIRECTION('',(-2.1716102378779E-15,3.83420712807775E-28,1.)) ;
#43699=DIRECTION('center_axis',(-1.66533453692587E-16,-1.,3.82991969484897E-28)) ;
#43700=DIRECTION('ref_axis',(2.1716102378779E-15,-3.83353615237885E-28,
-1.)) ;
#43701=DIRECTION('center_axis',(-2.17161023787787E-15,3.83815143260382E-28,
1.)) ;
#43702=DIRECTION('ref_axis',(-0.707106781186643,0.707106781186452,-1.53556032529805E-15)) ;
#43703=DIRECTION('center_axis',(-2.1716102378779E-15,3.83815143260386E-28,
1.)) ;
#43704=DIRECTION('ref_axis',(-0.707106781186643,0.707106781186452,-1.53556032529807E-15)) ;
#43705=DIRECTION('',(-2.1716102378779E-15,3.83815143260386E-28,1.)) ;
#43706=DIRECTION('center_axis',(-1.,1.66533453692966E-16,-2.1716102378779E-15)) ;
#43707=DIRECTION('ref_axis',(1.66533453692966E-16,1.,-3.82783884128008E-28)) ;
#43708=DIRECTION('',(2.1716102378779E-15,-3.83420712807775E-28,-1.)) ;
#43709=DIRECTION('center_axis',(2.1716102378779E-15,-3.83420712807775E-28,
-1.)) ;
#43710=DIRECTION('ref_axis',(-0.707106781186452,-0.707106781186643,-1.53556032529712E-15)) ;
#43711=DIRECTION('',(-2.1716102378779E-15,3.83420712807775E-28,1.)) ;
#43712=DIRECTION('center_axis',(-1.66533453692587E-16,-1.,3.82991969484897E-28)) ;
#43713=DIRECTION('ref_axis',(2.1716102378779E-15,-3.83353615237885E-28,
-1.)) ;
#43714=DIRECTION('center_axis',(-2.17161023787787E-15,3.83815143260382E-28,
1.)) ;
#43715=DIRECTION('ref_axis',(-0.707106781186643,0.707106781186452,-1.53556032529805E-15)) ;
#43716=DIRECTION('center_axis',(-2.1716102378779E-15,3.83815143260386E-28,
1.)) ;
#43717=DIRECTION('ref_axis',(-0.707106781186643,0.707106781186452,-1.53556032529807E-15)) ;
#43718=DIRECTION('',(-2.1716102378779E-15,3.83815143260386E-28,1.)) ;
#43719=DIRECTION('center_axis',(-1.,1.66533453692966E-16,-2.1716102378779E-15)) ;
#43720=DIRECTION('ref_axis',(1.66533453692966E-16,1.,-3.82783884128008E-28)) ;
#43721=DIRECTION('',(2.1716102378779E-15,-3.83420712807775E-28,-1.)) ;
#43722=DIRECTION('center_axis',(2.1716102378779E-15,-3.83420712807775E-28,
-1.)) ;
#43723=DIRECTION('ref_axis',(-0.707106781186452,-0.707106781186643,-1.53556032529712E-15)) ;
#43724=DIRECTION('',(-2.1716102378779E-15,3.83420712807775E-28,1.)) ;
#43725=DIRECTION('center_axis',(-1.66533453692587E-16,-1.,3.82991969484897E-28)) ;
#43726=DIRECTION('ref_axis',(2.1716102378779E-15,-3.83353615237885E-28,
-1.)) ;
#43727=DIRECTION('center_axis',(-2.17161023787787E-15,3.83815143260382E-28,
1.)) ;
#43728=DIRECTION('ref_axis',(-0.707106781186643,0.707106781186452,-1.53556032529805E-15)) ;
#43729=DIRECTION('center_axis',(-2.1716102378779E-15,3.83815143260386E-28,
1.)) ;
#43730=DIRECTION('ref_axis',(-0.707106781186643,0.707106781186452,-1.53556032529807E-15)) ;
#43731=DIRECTION('',(-2.1716102378779E-15,3.83815143260386E-28,1.)) ;
#43732=DIRECTION('center_axis',(-1.,1.66533453692966E-16,-2.1716102378779E-15)) ;
#43733=DIRECTION('ref_axis',(1.66533453692966E-16,1.,-3.82783884128008E-28)) ;
#43734=DIRECTION('',(2.1716102378779E-15,-3.83420712807775E-28,-1.)) ;
#43735=DIRECTION('center_axis',(2.1716102378779E-15,-3.83420712807775E-28,
-1.)) ;
#43736=DIRECTION('ref_axis',(-0.707106781186452,-0.707106781186643,-1.53556032529712E-15)) ;
#43737=DIRECTION('',(-2.1716102378779E-15,3.83420712807775E-28,1.)) ;
#43738=DIRECTION('center_axis',(-1.66533453692587E-16,-1.,3.82991969484897E-28)) ;
#43739=DIRECTION('ref_axis',(2.1716102378779E-15,-3.83353615237885E-28,
-1.)) ;
#43740=DIRECTION('center_axis',(-2.17161023787787E-15,3.83815143260382E-28,
1.)) ;
#43741=DIRECTION('ref_axis',(-0.707106781186643,0.707106781186452,-1.53556032529805E-15)) ;
#43742=DIRECTION('center_axis',(-2.1716102378779E-15,3.83815143260386E-28,
1.)) ;
#43743=DIRECTION('ref_axis',(-0.707106781186643,0.707106781186452,-1.53556032529807E-15)) ;
#43744=DIRECTION('',(-2.1716102378779E-15,3.83815143260386E-28,1.)) ;
#43745=DIRECTION('center_axis',(-1.,1.66533453692966E-16,-2.1716102378779E-15)) ;
#43746=DIRECTION('ref_axis',(1.66533453692966E-16,1.,-3.82783884128008E-28)) ;
#43747=DIRECTION('',(2.1716102378779E-15,-3.83420712807775E-28,-1.)) ;
#43748=DIRECTION('center_axis',(2.1716102378779E-15,-3.83420712807775E-28,
-1.)) ;
#43749=DIRECTION('ref_axis',(-0.707106781186452,-0.707106781186643,-1.53556032529712E-15)) ;
#43750=DIRECTION('',(-2.1716102378779E-15,3.83420712807775E-28,1.)) ;
#43751=DIRECTION('center_axis',(-1.66533453692587E-16,-1.,3.82991969484897E-28)) ;
#43752=DIRECTION('ref_axis',(2.1716102378779E-15,-3.83353615237885E-28,
-1.)) ;
#43753=DIRECTION('center_axis',(-2.17161023787787E-15,3.83815143260382E-28,
1.)) ;
#43754=DIRECTION('ref_axis',(-0.707106781186643,0.707106781186452,-1.53556032529805E-15)) ;
#69339=CARTESIAN_POINT('',(0.,0.,0.)) ;
#69340=CARTESIAN_POINT('Origin',(194.588527625411,554.617826199637,-31.0221601717604)) ;
#69341=CARTESIAN_POINT('',(194.588527625411,554.617826199637,-31.0221601717604)) ;
#69342=CARTESIAN_POINT('',(194.58852762541,546.397107238503,-31.0221601717604)) ;
#69343=CARTESIAN_POINT('',(194.588527625412,562.045191394428,-31.0221601717604)) ;
#69344=CARTESIAN_POINT('',(197.588527625411,554.617826199637,-31.0221601717605)) ;
#69345=CARTESIAN_POINT('',(194.588527625411,554.617826199637,-31.0221601717604)) ;
#69346=CARTESIAN_POINT('',(197.58852762541,546.397107238503,-31.0221601717605)) ;
#69347=CARTESIAN_POINT('',(197.588527625411,554.617826199637,-31.0221601717605)) ;
#69348=CARTESIAN_POINT('',(194.58852762541,546.397107238503,-31.0221601717604)) ;
#69349=CARTESIAN_POINT('Origin',(194.588527625411,554.617826199637,-41.5221601717604)) ;
#69350=CARTESIAN_POINT('',(194.588527625411,554.617826199637,-41.5221601717604)) ;
#69351=CARTESIAN_POINT('',(194.588527625411,554.617826199637,-37.7721601717604)) ;
#69352=CARTESIAN_POINT('',(197.588527625411,554.617826199637,-41.5221601717605)) ;
#69353=CARTESIAN_POINT('',(203.58852762541,554.617826199636,-41.5221601717608)) ;
#69354=CARTESIAN_POINT('',(197.588527625411,554.617826199637,-41.5221601717605)) ;
#69355=CARTESIAN_POINT('Origin',(194.58852762541,546.397107238503,-31.0221601717604)) ;
#69356=CARTESIAN_POINT('',(194.588527625409,546.397107238503,-41.5221601717604)) ;
#69357=CARTESIAN_POINT('',(194.58852762541,546.397107238503,-32.5221601717604)) ;
#69358=CARTESIAN_POINT('',(197.588527625409,546.397107238503,-41.5221601717605)) ;
#69359=CARTESIAN_POINT('',(197.58852762541,546.397107238503,-31.0221601717605)) ;
#69360=CARTESIAN_POINT('',(203.588527625409,546.397107238502,-41.5221601717608)) ;
#69361=CARTESIAN_POINT('Origin',(197.588527625413,569.472556589218,-34.0221601717605)) ;
#69362=CARTESIAN_POINT('',(197.588527625409,547.972556589215,-41.5221601717605)) ;
#69363=CARTESIAN_POINT('Origin',(194.588527625418,592.617826199638,-31.0221601717604)) ;
#69364=CARTESIAN_POINT('',(194.588527625418,592.617826199638,-31.0221601717604)) ;
#69365=CARTESIAN_POINT('',(194.588527625416,584.397107238503,-31.0221601717604)) ;
#69366=CARTESIAN_POINT('',(194.588527625416,581.045191394428,-31.0221601717604)) ;
#69367=CARTESIAN_POINT('',(197.588527625418,592.617826199637,-31.0221601717605)) ;
#69368=CARTESIAN_POINT('',(194.588527625418,592.617826199638,-31.0221601717604)) ;
#69369=CARTESIAN_POINT('',(197.588527625416,584.397107238503,-31.0221601717605)) ;
#69370=CARTESIAN_POINT('',(197.588527625418,592.617826199637,-31.0221601717605)) ;
#69371=CARTESIAN_POINT('',(194.588527625416,584.397107238503,-31.0221601717604)) ;
#69372=CARTESIAN_POINT('Origin',(194.588527625417,592.617826199638,-41.5221601717604)) ;
#69373=CARTESIAN_POINT('',(194.588527625417,592.617826199638,-41.5221601717604)) ;
#69374=CARTESIAN_POINT('',(194.588527625417,592.617826199638,-37.7721601717604)) ;
#69375=CARTESIAN_POINT('',(197.588527625417,592.617826199637,-41.5221601717605)) ;
#69376=CARTESIAN_POINT('',(203.588527625417,592.617826199636,-41.5221601717608)) ;
#69377=CARTESIAN_POINT('',(197.588527625417,592.617826199637,-41.5221601717605)) ;
#69378=CARTESIAN_POINT('Origin',(194.588527625416,584.397107238503,-31.0221601717604)) ;
#69379=CARTESIAN_POINT('',(194.588527625416,584.397107238503,-41.5221601717604)) ;
#69380=CARTESIAN_POINT('',(194.588527625416,584.397107238503,-32.5221601717604)) ;
#69381=CARTESIAN_POINT('',(197.588527625416,584.397107238503,-41.5221601717605)) ;
#69382=CARTESIAN_POINT('',(197.588527625416,584.397107238503,-31.0221601717605)) ;
#69383=CARTESIAN_POINT('',(203.588527625415,584.397107238502,-41.5221601717608)) ;
#69384=CARTESIAN_POINT('Origin',(197.588527625414,569.472556589218,-34.0221601717605)) ;
#69385=CARTESIAN_POINT('',(197.58852762541,547.972556589215,-41.5221601717605)) ;
#69386=CARTESIAN_POINT('Origin',(194.588527625418,593.897107238503,-31.0221601717604)) ;
#69387=CARTESIAN_POINT('',(194.588527625418,593.897107238503,-31.0221601717604)) ;
#69388=CARTESIAN_POINT('',(194.588527625417,593.897107238503,-41.5221601717604)) ;
#69389=CARTESIAN_POINT('',(194.588527625418,593.897107238503,-32.5221601717604)) ;
#69390=CARTESIAN_POINT('',(197.588527625418,593.897107238503,-31.0221601717605)) ;
#69391=CARTESIAN_POINT('',(194.588527625418,593.897107238503,-31.0221601717604)) ;
#69392=CARTESIAN_POINT('',(197.588527625417,593.897107238503,-41.5221601717605)) ;
#69393=CARTESIAN_POINT('',(197.588527625418,593.897107238503,-31.0221601717605)) ;
#69394=CARTESIAN_POINT('',(203.588527625417,593.897107238502,-41.5221601717608)) ;
#69395=CARTESIAN_POINT('Origin',(194.588527625419,602.117826199638,-31.0221601717604)) ;
#69396=CARTESIAN_POINT('',(194.588527625419,602.117826199638,-31.0221601717604)) ;
#69397=CARTESIAN_POINT('',(194.588527625417,585.795191394428,-31.0221601717604)) ;
#69398=CARTESIAN_POINT('',(197.588527625419,602.117826199637,-31.0221601717605)) ;
#69399=CARTESIAN_POINT('',(194.588527625419,602.117826199638,-31.0221601717604)) ;
#69400=CARTESIAN_POINT('',(197.588527625419,602.117826199637,-31.0221601717605)) ;
#69401=CARTESIAN_POINT('Origin',(194.588527625419,602.117826199638,-41.5221601717604)) ;
#69402=CARTESIAN_POINT('',(194.588527625419,602.117826199638,-41.5221601717604)) ;
#69403=CARTESIAN_POINT('',(194.588527625419,602.117826199638,-37.7721601717604)) ;
#69404=CARTESIAN_POINT('',(197.588527625419,602.117826199637,-41.5221601717605)) ;
#69405=CARTESIAN_POINT('',(203.588527625419,602.117826199636,-41.5221601717608)) ;
#69406=CARTESIAN_POINT('',(197.588527625419,602.117826199637,-41.5221601717605)) ;
#69407=CARTESIAN_POINT('Origin',(197.588527625414,569.472556589218,-34.0221601717605)) ;
#69408=CARTESIAN_POINT('',(197.58852762541,547.972556589215,-41.5221601717605)) ;
#69409=CARTESIAN_POINT('Origin',(194.588527625413,564.117826199637,-31.0221601717604)) ;
#69410=CARTESIAN_POINT('',(194.588527625413,564.117826199637,-31.0221601717604)) ;
#69411=CARTESIAN_POINT('',(194.588527625411,555.897107238503,-31.0221601717604)) ;
#69412=CARTESIAN_POINT('',(194.588527625413,566.795191394428,-31.0221601717604)) ;
#69413=CARTESIAN_POINT('',(197.588527625413,564.117826199637,-31.0221601717605)) ;
#69414=CARTESIAN_POINT('',(194.588527625413,564.117826199637,-31.0221601717604)) ;
#69415=CARTESIAN_POINT('',(197.588527625411,555.897107238503,-31.0221601717605)) ;
#69416=CARTESIAN_POINT('',(197.588527625413,564.117826199637,-31.0221601717605)) ;
#69417=CARTESIAN_POINT('',(194.588527625411,555.897107238503,-31.0221601717604)) ;
#69418=CARTESIAN_POINT('Origin',(194.588527625412,564.117826199637,-41.5221601717604)) ;
#69419=CARTESIAN_POINT('',(194.588527625412,564.117826199637,-41.5221601717604)) ;
#69420=CARTESIAN_POINT('',(194.588527625412,564.117826199637,-37.7721601717604)) ;
#69421=CARTESIAN_POINT('',(197.588527625412,564.117826199637,-41.5221601717605)) ;
#69422=CARTESIAN_POINT('',(203.588527625412,564.117826199636,-41.5221601717608)) ;
#69423=CARTESIAN_POINT('',(197.588527625412,564.117826199637,-41.5221601717605)) ;
#69424=CARTESIAN_POINT('Origin',(194.588527625411,555.897107238503,-31.0221601717604)) ;
#69425=CARTESIAN_POINT('',(194.588527625411,555.897107238503,-41.5221601717604)) ;
#69426=CARTESIAN_POINT('',(194.588527625411,555.897107238503,-32.5221601717604)) ;
#69427=CARTESIAN_POINT('',(197.588527625411,555.897107238503,-41.5221601717605)) ;
#69428=CARTESIAN_POINT('',(197.588527625411,555.897107238503,-31.0221601717605)) ;
#69429=CARTESIAN_POINT('',(203.588527625411,555.897107238502,-41.5221601717608)) ;
#69430=CARTESIAN_POINT('Origin',(197.588527625413,569.472556589218,-34.0221601717605)) ;
#69431=CARTESIAN_POINT('',(197.58852762541,547.972556589215,-41.5221601717605)) ;
#69432=CARTESIAN_POINT('Origin',(194.588527625409,545.117826199637,-31.0221601717604)) ;
#69433=CARTESIAN_POINT('',(194.588527625409,545.117826199637,-31.0221601717604)) ;
#69434=CARTESIAN_POINT('',(194.588527625408,536.897107238503,-31.0221601717604)) ;
#69435=CARTESIAN_POINT('',(194.588527625412,557.295191394428,-31.0221601717604)) ;
#69436=CARTESIAN_POINT('',(197.588527625409,545.117826199637,-31.0221601717605)) ;
#69437=CARTESIAN_POINT('',(194.588527625409,545.117826199637,-31.0221601717604)) ;
#69438=CARTESIAN_POINT('',(197.588527625408,536.897107238502,-31.0221601717605)) ;
#69439=CARTESIAN_POINT('',(197.588527625409,545.117826199637,-31.0221601717605)) ;
#69440=CARTESIAN_POINT('',(194.588527625408,536.897107238503,-31.0221601717604)) ;
#69441=CARTESIAN_POINT('Origin',(194.588527625409,545.117826199637,-41.5221601717604)) ;
#69442=CARTESIAN_POINT('',(194.588527625409,545.117826199637,-41.5221601717604)) ;
#69443=CARTESIAN_POINT('',(194.588527625409,545.117826199637,-37.7721601717604)) ;
#69444=CARTESIAN_POINT('',(197.588527625409,545.117826199637,-41.5221601717605)) ;
#69445=CARTESIAN_POINT('',(203.588527625409,545.117826199636,-41.5221601717608)) ;
#69446=CARTESIAN_POINT('',(197.588527625409,545.117826199637,-41.5221601717605)) ;
#69447=CARTESIAN_POINT('Origin',(194.588527625408,536.897107238503,-31.0221601717604)) ;
#69448=CARTESIAN_POINT('',(194.588527625408,536.897107238503,-41.5221601717604)) ;
#69449=CARTESIAN_POINT('',(194.588527625408,536.897107238503,-32.5221601717604)) ;
#69450=CARTESIAN_POINT('',(197.588527625408,536.897107238502,-41.5221601717605)) ;
#69451=CARTESIAN_POINT('',(197.588527625408,536.897107238502,-31.0221601717605)) ;
#69452=CARTESIAN_POINT('',(203.588527625407,536.897107238502,-41.5221601717608)) ;
#69453=CARTESIAN_POINT('Origin',(197.588527625413,569.472556589218,-34.0221601717605)) ;
#69454=CARTESIAN_POINT('',(197.588527625409,547.972556589215,-41.5221601717605)) ;
#69455=CARTESIAN_POINT('Origin',(194.588527625416,583.117826199638,-31.0221601717604)) ;
#69456=CARTESIAN_POINT('',(194.588527625416,583.117826199638,-31.0221601717604)) ;
#69457=CARTESIAN_POINT('',(194.588527625415,574.897107238503,-31.0221601717604)) ;
#69458=CARTESIAN_POINT('',(194.588527625415,576.295191394428,-31.0221601717604)) ;
#69459=CARTESIAN_POINT('',(197.588527625416,583.117826199637,-31.0221601717605)) ;
#69460=CARTESIAN_POINT('',(194.588527625416,583.117826199638,-31.0221601717604)) ;
#69461=CARTESIAN_POINT('',(197.588527625415,574.897107238503,-31.0221601717605)) ;
#69462=CARTESIAN_POINT('',(197.588527625416,583.117826199637,-31.0221601717605)) ;
#69463=CARTESIAN_POINT('',(194.588527625415,574.897107238503,-31.0221601717604)) ;
#69464=CARTESIAN_POINT('Origin',(194.588527625416,583.117826199638,-41.5221601717604)) ;
#69465=CARTESIAN_POINT('',(194.588527625416,583.117826199638,-41.5221601717604)) ;
#69466=CARTESIAN_POINT('',(194.588527625416,583.117826199638,-37.7721601717604)) ;
#69467=CARTESIAN_POINT('',(197.588527625416,583.117826199637,-41.5221601717605)) ;
#69468=CARTESIAN_POINT('',(203.588527625415,583.117826199636,-41.5221601717608)) ;
#69469=CARTESIAN_POINT('',(197.588527625416,583.117826199637,-41.5221601717605)) ;
#69470=CARTESIAN_POINT('Origin',(194.588527625415,574.897107238503,-31.0221601717604)) ;
#69471=CARTESIAN_POINT('',(194.588527625414,574.897107238503,-41.5221601717604)) ;
#69472=CARTESIAN_POINT('',(194.588527625415,574.897107238503,-32.5221601717604)) ;
#69473=CARTESIAN_POINT('',(197.588527625414,574.897107238503,-41.5221601717605)) ;
#69474=CARTESIAN_POINT('',(197.588527625415,574.897107238503,-31.0221601717605)) ;
#69475=CARTESIAN_POINT('',(203.588527625414,574.897107238502,-41.5221601717608)) ;
#69476=CARTESIAN_POINT('Origin',(197.588527625414,569.472556589218,-34.0221601717605)) ;
#69477=CARTESIAN_POINT('',(197.58852762541,547.972556589215,-41.5221601717605)) ;
#69478=CARTESIAN_POINT('Origin',(194.58852762542,603.397107238503,-31.0221601717604)) ;
#69479=CARTESIAN_POINT('',(194.58852762542,603.397107238503,-31.0221601717604)) ;
#69480=CARTESIAN_POINT('',(194.588527625419,603.397107238503,-41.5221601717604)) ;
#69481=CARTESIAN_POINT('',(194.58852762542,603.397107238503,-32.5221601717604)) ;
#69482=CARTESIAN_POINT('',(197.58852762542,603.397107238503,-31.0221601717605)) ;
#69483=CARTESIAN_POINT('',(194.58852762542,603.397107238503,-31.0221601717604)) ;
#69484=CARTESIAN_POINT('',(197.588527625419,603.397107238503,-41.5221601717605)) ;
#69485=CARTESIAN_POINT('',(197.58852762542,603.397107238503,-31.0221601717605)) ;
#69486=CARTESIAN_POINT('',(203.588527625419,603.397107238502,-41.5221601717608)) ;
#69487=CARTESIAN_POINT('Origin',(194.588527625421,611.617826199638,-31.0221601717604)) ;
#69488=CARTESIAN_POINT('',(194.588527625421,611.617826199638,-31.0221601717604)) ;
#69489=CARTESIAN_POINT('',(194.588527625417,590.545191394428,-31.0221601717604)) ;
#69490=CARTESIAN_POINT('',(197.588527625421,611.617826199637,-31.0221601717605)) ;
#69491=CARTESIAN_POINT('',(194.588527625421,611.617826199638,-31.0221601717604)) ;
#69492=CARTESIAN_POINT('',(197.588527625421,611.617826199637,-31.0221601717605)) ;
#69493=CARTESIAN_POINT('Origin',(194.588527625421,611.617826199638,-41.5221601717604)) ;
#69494=CARTESIAN_POINT('',(194.588527625421,611.617826199638,-41.5221601717604)) ;
#69495=CARTESIAN_POINT('',(194.588527625421,611.617826199638,-37.7721601717604)) ;
#69496=CARTESIAN_POINT('',(197.588527625421,611.617826199637,-41.5221601717605)) ;
#69497=CARTESIAN_POINT('',(203.58852762542,611.617826199636,-41.5221601717608)) ;
#69498=CARTESIAN_POINT('',(197.588527625421,611.617826199637,-41.5221601717605)) ;
#69499=CARTESIAN_POINT('Origin',(197.588527625414,569.472556589218,-34.0221601717605)) ;
#69500=CARTESIAN_POINT('',(197.58852762541,547.972556589215,-41.5221601717605)) ;
#69501=CARTESIAN_POINT('Origin',(194.588527625414,573.617826199637,-31.0221601717604)) ;
#69502=CARTESIAN_POINT('',(194.588527625414,573.617826199637,-31.0221601717604)) ;
#69503=CARTESIAN_POINT('',(194.588527625413,565.397107238503,-31.0221601717604)) ;
#69504=CARTESIAN_POINT('',(194.588527625414,571.545191394428,-31.0221601717604)) ;
#69505=CARTESIAN_POINT('',(197.588527625414,573.617826199637,-31.0221601717605)) ;
#69506=CARTESIAN_POINT('',(194.588527625414,573.617826199637,-31.0221601717604)) ;
#69507=CARTESIAN_POINT('',(197.588527625413,565.397107238503,-31.0221601717605)) ;
#69508=CARTESIAN_POINT('',(197.588527625414,573.617826199637,-31.0221601717605)) ;
#69509=CARTESIAN_POINT('',(194.588527625413,565.397107238503,-31.0221601717604)) ;
#69510=CARTESIAN_POINT('Origin',(194.588527625414,573.617826199637,-41.5221601717604)) ;
#69511=CARTESIAN_POINT('',(194.588527625414,573.617826199637,-41.5221601717604)) ;
#69512=CARTESIAN_POINT('',(194.588527625414,573.617826199637,-37.7721601717604)) ;
#69513=CARTESIAN_POINT('',(197.588527625414,573.617826199637,-41.5221601717605)) ;
#69514=CARTESIAN_POINT('',(203.588527625414,573.617826199636,-41.5221601717608)) ;
#69515=CARTESIAN_POINT('',(197.588527625414,573.617826199637,-41.5221601717605)) ;
#69516=CARTESIAN_POINT('Origin',(194.588527625413,565.397107238503,-31.0221601717604)) ;
#69517=CARTESIAN_POINT('',(194.588527625413,565.397107238503,-41.5221601717604)) ;
#69518=CARTESIAN_POINT('',(194.588527625413,565.397107238503,-32.5221601717604)) ;
#69519=CARTESIAN_POINT('',(197.588527625413,565.397107238503,-41.5221601717605)) ;
#69520=CARTESIAN_POINT('',(197.588527625413,565.397107238503,-31.0221601717605)) ;
#69521=CARTESIAN_POINT('',(203.588527625412,565.397107238502,-41.5221601717608)) ;
#69522=CARTESIAN_POINT('Origin',(197.588527625414,569.472556589218,-34.0221601717605)) ;
#69523=CARTESIAN_POINT('',(197.58852762541,547.972556589215,-41.5221601717605)) ;
#69524=CARTESIAN_POINT('Origin',(194.588527625408,535.617826199637,-31.0221601717604)) ;
#69525=CARTESIAN_POINT('',(194.588527625408,535.617826199637,-31.0221601717604)) ;
#69526=CARTESIAN_POINT('',(194.588527625406,527.397107238503,-31.0221601717604)) ;
#69527=CARTESIAN_POINT('',(194.588527625411,552.545191394428,-31.0221601717604)) ;
#69528=CARTESIAN_POINT('',(197.588527625408,535.617826199637,-31.0221601717605)) ;
#69529=CARTESIAN_POINT('',(194.588527625408,535.617826199637,-31.0221601717604)) ;
#69530=CARTESIAN_POINT('',(197.588527625406,527.397107238502,-31.0221601717605)) ;
#69531=CARTESIAN_POINT('',(197.588527625408,535.617826199637,-31.0221601717605)) ;
#69532=CARTESIAN_POINT('',(194.588527625406,527.397107238503,-31.0221601717604)) ;
#69533=CARTESIAN_POINT('Origin',(194.588527625407,535.617826199637,-41.5221601717604)) ;
#69534=CARTESIAN_POINT('',(194.588527625407,535.617826199637,-41.5221601717604)) ;
#69535=CARTESIAN_POINT('',(194.588527625408,535.617826199637,-37.7721601717604)) ;
#69536=CARTESIAN_POINT('',(197.588527625407,535.617826199637,-41.5221601717605)) ;
#69537=CARTESIAN_POINT('',(203.588527625407,535.617826199636,-41.5221601717608)) ;
#69538=CARTESIAN_POINT('',(197.588527625407,535.617826199637,-41.5221601717605)) ;
#69539=CARTESIAN_POINT('Origin',(194.588527625406,527.397107238503,-31.0221601717604)) ;
#69540=CARTESIAN_POINT('',(194.588527625406,527.397107238503,-41.5221601717604)) ;
#69541=CARTESIAN_POINT('',(194.588527625406,527.397107238503,-32.5221601717604)) ;
#69542=CARTESIAN_POINT('',(197.588527625406,527.397107238502,-41.5221601717605)) ;
#69543=CARTESIAN_POINT('',(197.588527625406,527.397107238502,-31.0221601717605)) ;
#69544=CARTESIAN_POINT('',(203.588527625406,527.397107238502,-41.5221601717608)) ;
#69545=CARTESIAN_POINT('Origin',(197.588527625413,569.472556589218,-34.0221601717605)) ;
#69546=CARTESIAN_POINT('',(197.588527625409,547.972556589215,-41.5221601717605)) ;
#69547=CARTESIAN_POINT('Origin',(212.588527625406,526.47255658921,-41.5221601717612)) ;
#69548=CARTESIAN_POINT('',(194.588527625421,613.010565160533,-41.5221601717604)) ;
#69549=CARTESIAN_POINT('',(194.588527625421,613.010565160533,-41.5221601717604)) ;
#69550=CARTESIAN_POINT('',(194.588527625421,613.010565160533,-41.5221601717604)) ;
#69551=CARTESIAN_POINT('',(194.588527625421,613.010565160533,-41.5221601717604)) ;
#69552=CARTESIAN_POINT('',(194.588527625421,613.010565160533,-41.5221601717604)) ;
#69553=CARTESIAN_POINT('',(194.588527625421,613.010565160533,-41.5221601717604)) ;
#69554=CARTESIAN_POINT('',(194.588527625421,613.010565160533,-41.5221601717604)) ;
#69555=CARTESIAN_POINT('',(194.588527625421,613.010565160533,-41.5221601717604)) ;
#69556=CARTESIAN_POINT('',(212.588527625421,613.01056516053,-41.5221601717612)) ;
#69557=CARTESIAN_POINT('',(212.388527625421,613.01056516053,-41.5221601717612)) ;
#69558=CARTESIAN_POINT('',(212.58852762542,611.54800593993,-41.5221601717612)) ;
#69559=CARTESIAN_POINT('',(212.588527625421,613.01056516053,-41.5221601717612)) ;
#69560=CARTESIAN_POINT('',(199.088527625421,611.548005939932,-41.5221601717606)) ;
#69561=CARTESIAN_POINT('',(212.58852762542,611.548005939915,-41.5221601717612)) ;
#69562=CARTESIAN_POINT('',(199.088527625419,603.397107238502,-41.5221601717606)) ;
#69563=CARTESIAN_POINT('',(199.088527625421,613.010565160532,-41.5221601717606)) ;
#69564=CARTESIAN_POINT('',(212.588527625419,603.3971072385,-41.5221601717612)) ;
#69565=CARTESIAN_POINT('',(205.838527625419,603.397107238493,-41.5221601717609)) ;
#69566=CARTESIAN_POINT('',(212.588527625419,602.04800593993,-41.5221601717612)) ;
#69567=CARTESIAN_POINT('',(212.588527625421,613.01056516053,-41.5221601717612)) ;
#69568=CARTESIAN_POINT('',(199.088527625419,602.048005939932,-41.5221601717606)) ;
#69569=CARTESIAN_POINT('',(212.588527625419,602.048005939935,-41.5221601717612)) ;
#69570=CARTESIAN_POINT('',(199.088527625417,593.897107238502,-41.5221601717606)) ;
#69571=CARTESIAN_POINT('',(199.088527625421,613.010565160532,-41.5221601717606)) ;
#69572=CARTESIAN_POINT('',(212.588527625417,593.8971072385,-41.5221601717612)) ;
#69573=CARTESIAN_POINT('',(205.838527625417,593.897107238493,-41.5221601717609)) ;
#69574=CARTESIAN_POINT('',(212.588527625417,592.54800593993,-41.5221601717612)) ;
#69575=CARTESIAN_POINT('',(212.588527625421,613.01056516053,-41.5221601717612)) ;
#69576=CARTESIAN_POINT('',(199.088527625417,592.548005939932,-41.5221601717606)) ;
#69577=CARTESIAN_POINT('',(212.588527625417,592.548005939935,-41.5221601717612)) ;
#69578=CARTESIAN_POINT('',(199.088527625416,584.397107238502,-41.5221601717606)) ;
#69579=CARTESIAN_POINT('',(199.088527625421,613.010565160532,-41.5221601717606)) ;
#69580=CARTESIAN_POINT('',(212.588527625416,584.3971072385,-41.5221601717612)) ;
#69581=CARTESIAN_POINT('',(205.838527625416,584.397107238493,-41.5221601717609)) ;
#69582=CARTESIAN_POINT('',(212.588527625416,583.04800593993,-41.5221601717612)) ;
#69583=CARTESIAN_POINT('',(212.588527625421,613.01056516053,-41.5221601717612)) ;
#69584=CARTESIAN_POINT('',(199.088527625416,583.048005939932,-41.5221601717606)) ;
#69585=CARTESIAN_POINT('',(212.588527625416,583.048005939935,-41.5221601717612)) ;
#69586=CARTESIAN_POINT('',(199.088527625414,574.897107238502,-41.5221601717606)) ;
#69587=CARTESIAN_POINT('',(199.088527625421,613.010565160532,-41.5221601717606)) ;
#69588=CARTESIAN_POINT('',(212.588527625414,574.8971072385,-41.5221601717612)) ;
#69589=CARTESIAN_POINT('',(205.838527625414,574.897107238493,-41.5221601717609)) ;
#69590=CARTESIAN_POINT('',(212.588527625414,573.54800593993,-41.5221601717612)) ;
#69591=CARTESIAN_POINT('',(212.588527625421,613.01056516053,-41.5221601717612)) ;
#69592=CARTESIAN_POINT('',(199.088527625414,573.548005939932,-41.5221601717606)) ;
#69593=CARTESIAN_POINT('',(212.588527625414,573.548005939935,-41.5221601717612)) ;
#69594=CARTESIAN_POINT('',(199.088527625412,565.397107238502,-41.5221601717606)) ;
#69595=CARTESIAN_POINT('',(199.088527625421,613.010565160532,-41.5221601717606)) ;
#69596=CARTESIAN_POINT('',(212.588527625412,565.3971072385,-41.5221601717612)) ;
#69597=CARTESIAN_POINT('',(205.838527625412,565.397107238497,-41.5221601717609)) ;
#69598=CARTESIAN_POINT('',(212.588527625412,564.04800593993,-41.5221601717612)) ;
#69599=CARTESIAN_POINT('',(212.588527625421,613.01056516053,-41.5221601717612)) ;
#69600=CARTESIAN_POINT('',(199.088527625412,564.048005939932,-41.5221601717606)) ;
#69601=CARTESIAN_POINT('',(212.588527625412,564.048005939928,-41.5221601717612)) ;
#69602=CARTESIAN_POINT('',(199.088527625411,555.897107238502,-41.5221601717606)) ;
#69603=CARTESIAN_POINT('',(199.088527625421,613.010565160532,-41.5221601717606)) ;
#69604=CARTESIAN_POINT('',(212.588527625411,555.8971072385,-41.5221601717612)) ;
#69605=CARTESIAN_POINT('',(205.838527625411,555.897107238496,-41.5221601717609)) ;
#69606=CARTESIAN_POINT('',(212.588527625411,554.54800593993,-41.5221601717612)) ;
#69607=CARTESIAN_POINT('',(212.588527625421,613.01056516053,-41.5221601717612)) ;
#69608=CARTESIAN_POINT('',(199.088527625411,554.548005939932,-41.5221601717606)) ;
#69609=CARTESIAN_POINT('',(212.588527625411,554.548005939928,-41.5221601717612)) ;
#69610=CARTESIAN_POINT('',(199.088527625409,546.397107238502,-41.5221601717606)) ;
#69611=CARTESIAN_POINT('',(199.088527625421,613.010565160532,-41.5221601717606)) ;
#69612=CARTESIAN_POINT('',(212.588527625409,546.3971072385,-41.5221601717612)) ;
#69613=CARTESIAN_POINT('',(205.838527625409,546.397107238497,-41.5221601717609)) ;
#69614=CARTESIAN_POINT('',(212.588527625409,545.04800593993,-41.5221601717612)) ;
#69615=CARTESIAN_POINT('',(212.588527625421,613.01056516053,-41.5221601717612)) ;
#69616=CARTESIAN_POINT('',(199.088527625409,545.048005939932,-41.5221601717606)) ;
#69617=CARTESIAN_POINT('',(212.588527625409,545.048005939928,-41.5221601717612)) ;
#69618=CARTESIAN_POINT('',(199.088527625407,536.897107238502,-41.5221601717606)) ;
#69619=CARTESIAN_POINT('',(199.088527625421,613.010565160532,-41.5221601717606)) ;
#69620=CARTESIAN_POINT('',(212.588527625407,536.8971072385,-41.5221601717612)) ;
#69621=CARTESIAN_POINT('',(205.838527625407,536.897107238496,-41.5221601717609)) ;
#69622=CARTESIAN_POINT('',(212.588527625407,535.54800593993,-41.5221601717612)) ;
#69623=CARTESIAN_POINT('',(212.588527625421,613.01056516053,-41.5221601717612)) ;
#69624=CARTESIAN_POINT('',(199.088527625407,535.548005939932,-41.5221601717606)) ;
#69625=CARTESIAN_POINT('',(212.588527625407,535.548005939928,-41.5221601717612)) ;
#69626=CARTESIAN_POINT('',(199.088527625406,527.397107238502,-41.5221601717606)) ;
#69627=CARTESIAN_POINT('',(199.088527625421,613.010565160532,-41.5221601717606)) ;
#69628=CARTESIAN_POINT('',(212.588527625406,527.3971072385,-41.5221601717612)) ;
#69629=CARTESIAN_POINT('',(205.838527625406,527.397107238497,-41.5221601717609)) ;
#69630=CARTESIAN_POINT('',(212.588527625406,525.9345480179,-41.5221601717612)) ;
#69631=CARTESIAN_POINT('',(212.588527625421,613.01056516053,-41.5221601717612)) ;
#69632=CARTESIAN_POINT('',(194.588527625405,525.934548017903,-41.5221601717604)) ;
#69633=CARTESIAN_POINT('',(199.088527625405,525.934548017902,-41.5221601717606)) ;
#69634=CARTESIAN_POINT('',(194.588527625421,613.010565160533,-41.5221601717604)) ;
#69635=CARTESIAN_POINT('',(194.588527625421,613.010565160533,-41.5221601717604)) ;
#69636=CARTESIAN_POINT('',(194.588527625421,613.010565160533,-41.5221601717604)) ;
#69637=CARTESIAN_POINT('Origin',(206.038527625421,607.472556589211,-40.3971601717609)) ;
#69638=CARTESIAN_POINT('',(207.538527625421,607.472556589211,-40.397160171761)) ;
#69639=CARTESIAN_POINT('Origin',(206.038527625421,607.472556589211,-40.3971601717609)) ;
#69640=CARTESIAN_POINT('',(207.663527625421,607.472556589211,-40.522160171761)) ;
#69641=CARTESIAN_POINT('Origin',(207.663527625421,607.472556589211,-40.397160171761)) ;
#69642=CARTESIAN_POINT('Origin',(206.038527625421,607.472556589211,-40.5221601717609)) ;
#69643=CARTESIAN_POINT('Origin',(206.038527625421,607.472556589211,-29.1521601717606)) ;
#69644=CARTESIAN_POINT('',(207.538527625421,607.472556589211,-37.0052690928546)) ;
#69645=CARTESIAN_POINT('Origin',(206.038527625421,607.472556589211,-37.0052690928546)) ;
#69646=CARTESIAN_POINT('',(207.538527625421,607.472556589211,-29.1521601717607)) ;
#69647=CARTESIAN_POINT('Origin',(205.838527625413,569.472556589214,-40.5221601717609)) ;
#69648=CARTESIAN_POINT('',(212.588527625419,603.3971072385,-40.5221601717612)) ;
#69649=CARTESIAN_POINT('',(212.588527625421,611.54800593993,-40.5221601717612)) ;
#69650=CARTESIAN_POINT('',(212.588527625409,547.972556589211,-40.5221601717612)) ;
#69651=CARTESIAN_POINT('',(199.088527625419,603.397107238502,-40.5221601717606)) ;
#69652=CARTESIAN_POINT('',(209.213527625419,603.397107238493,-40.5221601717611)) ;
#69653=CARTESIAN_POINT('',(199.088527625421,611.548005939932,-40.5221601717606)) ;
#69654=CARTESIAN_POINT('',(199.088527625409,547.972556589214,-40.5221601717606)) ;
#69655=CARTESIAN_POINT('',(202.463527625421,611.548005939916,-40.5221601717608)) ;
#69656=CARTESIAN_POINT('',(202.262277625404,608.357556589212,-40.5221601717608)) ;
#69657=CARTESIAN_POINT('',(201.559777625404,608.357556589212,-40.5221601717607)) ;
#69658=CARTESIAN_POINT('',(212.018652625407,608.357556589212,-40.5221601717612)) ;
#69659=CARTESIAN_POINT('',(201.184777625404,607.982556589212,-40.5221601717607)) ;
#69660=CARTESIAN_POINT('Origin',(201.559777625404,607.982556589212,-40.5221601717607)) ;
#69661=CARTESIAN_POINT('',(201.184777625405,606.962556589212,-40.5221601717607)) ;
#69662=CARTESIAN_POINT('',(201.184777625405,624.170681589212,-40.5221601717607)) ;
#69663=CARTESIAN_POINT('',(201.559777625405,606.587556589212,-40.5221601717607)) ;
#69664=CARTESIAN_POINT('Origin',(201.559777625404,606.962556589212,-40.5221601717607)) ;
#69665=CARTESIAN_POINT('',(202.262277625404,606.587556589212,-40.5221601717608)) ;
#69666=CARTESIAN_POINT('',(212.844152625407,606.587556589212,-40.5221601717612)) ;
#69667=CARTESIAN_POINT('',(202.637277625404,606.962556589212,-40.5221601717608)) ;
#69668=CARTESIAN_POINT('Origin',(202.262277625404,606.962556589212,-40.5221601717608)) ;
#69669=CARTESIAN_POINT('',(202.637277625404,607.982556589212,-40.5221601717608)) ;
#69670=CARTESIAN_POINT('',(202.637277625404,624.170681589213,-40.5221601717608)) ;
#69671=CARTESIAN_POINT('Origin',(202.262277625404,607.982556589212,-40.5221601717608)) ;
#69672=CARTESIAN_POINT('Origin',(206.038527625419,597.972556589211,-40.3971601717609)) ;
#69673=CARTESIAN_POINT('',(207.538527625419,597.972556589211,-40.397160171761)) ;
#69674=CARTESIAN_POINT('Origin',(206.038527625419,597.972556589211,-40.3971601717609)) ;
#69675=CARTESIAN_POINT('',(207.663527625419,597.972556589211,-40.522160171761)) ;
#69676=CARTESIAN_POINT('Origin',(207.663527625419,597.972556589211,-40.397160171761)) ;
#69677=CARTESIAN_POINT('Origin',(206.038527625419,597.972556589211,-40.5221601717609)) ;
#69678=CARTESIAN_POINT('Origin',(206.038527625419,597.972556589211,-29.1521601717606)) ;
#69679=CARTESIAN_POINT('',(207.538527625419,597.972556589211,-37.0052690928546)) ;
#69680=CARTESIAN_POINT('Origin',(206.038527625419,597.972556589211,-37.0052690928546)) ;
#69681=CARTESIAN_POINT('',(207.538527625419,597.972556589211,-29.1521601717607)) ;
#69682=CARTESIAN_POINT('Origin',(205.838527625413,569.472556589214,-40.5221601717609)) ;
#69683=CARTESIAN_POINT('',(212.588527625417,593.8971072385,-40.5221601717612)) ;
#69684=CARTESIAN_POINT('',(212.588527625419,602.04800593993,-40.5221601717612)) ;
#69685=CARTESIAN_POINT('',(212.588527625409,547.972556589211,-40.5221601717612)) ;
#69686=CARTESIAN_POINT('',(199.088527625417,593.897107238502,-40.5221601717606)) ;
#69687=CARTESIAN_POINT('',(209.213527625417,593.897107238493,-40.5221601717611)) ;
#69688=CARTESIAN_POINT('',(199.088527625419,602.048005939932,-40.5221601717606)) ;
#69689=CARTESIAN_POINT('',(199.088527625409,547.972556589214,-40.5221601717606)) ;
#69690=CARTESIAN_POINT('',(202.463527625419,602.048005939937,-40.5221601717608)) ;
#69691=CARTESIAN_POINT('',(202.262277625404,598.857556589212,-40.5221601717608)) ;
#69692=CARTESIAN_POINT('',(201.559777625405,598.857556589212,-40.5221601717607)) ;
#69693=CARTESIAN_POINT('',(212.018652625407,598.857556589212,-40.5221601717612)) ;
#69694=CARTESIAN_POINT('',(201.184777625405,598.482556589212,-40.5221601717607)) ;
#69695=CARTESIAN_POINT('Origin',(201.559777625405,598.482556589212,-40.5221601717607)) ;
#69696=CARTESIAN_POINT('',(201.184777625405,597.462556589212,-40.5221601717607)) ;
#69697=CARTESIAN_POINT('',(201.184777625405,614.670681589212,-40.5221601717607)) ;
#69698=CARTESIAN_POINT('',(201.559777625405,597.087556589212,-40.5221601717607)) ;
#69699=CARTESIAN_POINT('Origin',(201.559777625405,597.462556589212,-40.5221601717607)) ;
#69700=CARTESIAN_POINT('',(202.262277625404,597.087556589212,-40.5221601717608)) ;
#69701=CARTESIAN_POINT('',(212.844152625407,597.087556589212,-40.5221601717612)) ;
#69702=CARTESIAN_POINT('',(202.637277625404,597.462556589212,-40.5221601717608)) ;
#69703=CARTESIAN_POINT('Origin',(202.262277625404,597.462556589212,-40.5221601717608)) ;
#69704=CARTESIAN_POINT('',(202.637277625404,598.482556589212,-40.5221601717608)) ;
#69705=CARTESIAN_POINT('',(202.637277625404,614.670681589213,-40.5221601717608)) ;
#69706=CARTESIAN_POINT('Origin',(202.262277625404,598.482556589212,-40.5221601717608)) ;
#69707=CARTESIAN_POINT('Origin',(206.038527625417,588.472556589211,-40.3971601717609)) ;
#69708=CARTESIAN_POINT('',(207.538527625417,588.472556589211,-40.397160171761)) ;
#69709=CARTESIAN_POINT('Origin',(206.038527625417,588.472556589211,-40.3971601717609)) ;
#69710=CARTESIAN_POINT('',(207.663527625417,588.472556589211,-40.522160171761)) ;
#69711=CARTESIAN_POINT('Origin',(207.663527625417,588.472556589211,-40.397160171761)) ;
#69712=CARTESIAN_POINT('Origin',(206.038527625417,588.472556589211,-40.5221601717609)) ;
#69713=CARTESIAN_POINT('Origin',(206.038527625418,588.472556589211,-29.1521601717607)) ;
#69714=CARTESIAN_POINT('',(207.538527625417,588.472556589211,-37.0052690928546)) ;
#69715=CARTESIAN_POINT('Origin',(206.038527625417,588.472556589211,-37.0052690928546)) ;
#69716=CARTESIAN_POINT('',(207.538527625418,588.472556589211,-29.1521601717608)) ;
#69717=CARTESIAN_POINT('Origin',(205.838527625413,569.472556589214,-40.5221601717609)) ;
#69718=CARTESIAN_POINT('',(212.588527625416,584.3971072385,-40.5221601717612)) ;
#69719=CARTESIAN_POINT('',(212.588527625417,592.54800593993,-40.5221601717612)) ;
#69720=CARTESIAN_POINT('',(212.588527625409,547.972556589211,-40.5221601717612)) ;
#69721=CARTESIAN_POINT('',(199.088527625416,584.397107238502,-40.5221601717606)) ;
#69722=CARTESIAN_POINT('',(209.213527625416,584.397107238493,-40.5221601717611)) ;
#69723=CARTESIAN_POINT('',(199.088527625417,592.548005939932,-40.5221601717606)) ;
#69724=CARTESIAN_POINT('',(199.088527625409,547.972556589214,-40.5221601717606)) ;
#69725=CARTESIAN_POINT('',(202.463527625417,592.548005939937,-40.5221601717608)) ;
#69726=CARTESIAN_POINT('',(202.262277625405,589.357556589212,-40.5221601717608)) ;
#69727=CARTESIAN_POINT('',(201.559777625405,589.357556589212,-40.5221601717607)) ;
#69728=CARTESIAN_POINT('',(212.018652625408,589.357556589212,-40.5221601717612)) ;
#69729=CARTESIAN_POINT('',(201.184777625405,588.982556589212,-40.5221601717607)) ;
#69730=CARTESIAN_POINT('Origin',(201.559777625405,588.982556589212,-40.5221601717607)) ;
#69731=CARTESIAN_POINT('',(201.184777625405,587.962556589212,-40.5221601717607)) ;
#69732=CARTESIAN_POINT('',(201.184777625405,605.170681589212,-40.5221601717607)) ;
#69733=CARTESIAN_POINT('',(201.559777625405,587.587556589212,-40.5221601717607)) ;
#69734=CARTESIAN_POINT('Origin',(201.559777625405,587.962556589212,-40.5221601717607)) ;
#69735=CARTESIAN_POINT('',(202.262277625405,587.587556589212,-40.5221601717608)) ;
#69736=CARTESIAN_POINT('',(212.844152625407,587.587556589212,-40.5221601717612)) ;
#69737=CARTESIAN_POINT('',(202.637277625405,587.962556589212,-40.5221601717608)) ;
#69738=CARTESIAN_POINT('Origin',(202.262277625405,587.962556589212,-40.5221601717608)) ;
#69739=CARTESIAN_POINT('',(202.637277625405,588.982556589212,-40.5221601717608)) ;
#69740=CARTESIAN_POINT('',(202.637277625405,605.170681589213,-40.5221601717608)) ;
#69741=CARTESIAN_POINT('Origin',(202.262277625405,588.982556589212,-40.5221601717608)) ;
#69742=CARTESIAN_POINT('Origin',(206.038527625415,578.972556589211,-40.3971601717609)) ;
#69743=CARTESIAN_POINT('',(207.538527625415,578.972556589211,-40.397160171761)) ;
#69744=CARTESIAN_POINT('Origin',(206.038527625415,578.972556589211,-40.3971601717609)) ;
#69745=CARTESIAN_POINT('',(207.663527625415,578.972556589211,-40.522160171761)) ;
#69746=CARTESIAN_POINT('Origin',(207.663527625415,578.972556589211,-40.397160171761)) ;
#69747=CARTESIAN_POINT('Origin',(206.038527625415,578.972556589211,-40.5221601717609)) ;
#69748=CARTESIAN_POINT('Origin',(206.038527625416,578.972556589211,-29.1521601717607)) ;
#69749=CARTESIAN_POINT('',(207.538527625416,578.972556589211,-37.0052690928546)) ;
#69750=CARTESIAN_POINT('Origin',(206.038527625416,578.972556589211,-37.0052690928546)) ;
#69751=CARTESIAN_POINT('',(207.538527625416,578.972556589211,-29.1521601717608)) ;
#69752=CARTESIAN_POINT('Origin',(205.838527625413,569.472556589214,-40.5221601717609)) ;
#69753=CARTESIAN_POINT('',(212.588527625414,574.8971072385,-40.5221601717612)) ;
#69754=CARTESIAN_POINT('',(212.588527625416,583.04800593993,-40.5221601717612)) ;
#69755=CARTESIAN_POINT('',(212.588527625409,547.972556589211,-40.5221601717612)) ;
#69756=CARTESIAN_POINT('',(199.088527625414,574.897107238502,-40.5221601717606)) ;
#69757=CARTESIAN_POINT('',(209.213527625414,574.897107238493,-40.5221601717611)) ;
#69758=CARTESIAN_POINT('',(199.088527625416,583.048005939932,-40.5221601717606)) ;
#69759=CARTESIAN_POINT('',(199.088527625409,547.972556589214,-40.5221601717606)) ;
#69760=CARTESIAN_POINT('',(202.463527625416,583.048005939937,-40.5221601717608)) ;
#69761=CARTESIAN_POINT('',(202.262277625405,579.857556589212,-40.5221601717608)) ;
#69762=CARTESIAN_POINT('',(201.559777625405,579.857556589212,-40.5221601717607)) ;
#69763=CARTESIAN_POINT('',(212.018652625408,579.857556589212,-40.5221601717612)) ;
#69764=CARTESIAN_POINT('',(201.184777625405,579.482556589212,-40.5221601717607)) ;
#69765=CARTESIAN_POINT('Origin',(201.559777625405,579.482556589212,-40.5221601717607)) ;
#69766=CARTESIAN_POINT('',(201.184777625406,578.462556589212,-40.5221601717607)) ;
#69767=CARTESIAN_POINT('',(201.184777625406,595.670681589212,-40.5221601717607)) ;
#69768=CARTESIAN_POINT('',(201.559777625406,578.087556589212,-40.5221601717607)) ;
#69769=CARTESIAN_POINT('Origin',(201.559777625405,578.462556589212,-40.5221601717607)) ;
#69770=CARTESIAN_POINT('',(202.262277625405,578.087556589212,-40.5221601717608)) ;
#69771=CARTESIAN_POINT('',(212.844152625408,578.087556589212,-40.5221601717612)) ;
#69772=CARTESIAN_POINT('',(202.637277625405,578.462556589212,-40.5221601717608)) ;
#69773=CARTESIAN_POINT('Origin',(202.262277625405,578.462556589212,-40.5221601717608)) ;
#69774=CARTESIAN_POINT('',(202.637277625405,579.482556589212,-40.5221601717608)) ;
#69775=CARTESIAN_POINT('',(202.637277625405,595.670681589213,-40.5221601717608)) ;
#69776=CARTESIAN_POINT('Origin',(202.262277625405,579.482556589212,-40.5221601717608)) ;
#69777=CARTESIAN_POINT('Origin',(206.038527625414,569.472556589211,-40.3971601717609)) ;
#69778=CARTESIAN_POINT('',(207.538527625414,569.472556589211,-40.397160171761)) ;
#69779=CARTESIAN_POINT('Origin',(206.038527625414,569.472556589211,-40.3971601717609)) ;
#69780=CARTESIAN_POINT('',(207.663527625414,569.472556589211,-40.522160171761)) ;
#69781=CARTESIAN_POINT('Origin',(207.663527625414,569.472556589211,-40.397160171761)) ;
#69782=CARTESIAN_POINT('Origin',(206.038527625414,569.472556589211,-40.5221601717609)) ;
#69783=CARTESIAN_POINT('Origin',(206.038527625414,569.472556589211,-29.1521601717607)) ;
#69784=CARTESIAN_POINT('',(207.538527625414,569.472556589211,-37.0052690928546)) ;
#69785=CARTESIAN_POINT('Origin',(206.038527625414,569.472556589211,-37.0052690928546)) ;
#69786=CARTESIAN_POINT('',(207.538527625414,569.472556589211,-29.1521601717608)) ;
#69787=CARTESIAN_POINT('Origin',(205.838527625413,569.472556589214,-40.5221601717609)) ;
#69788=CARTESIAN_POINT('',(199.088527625414,573.548005939932,-40.5221601717606)) ;
#69789=CARTESIAN_POINT('',(199.088527625412,565.397107238502,-40.5221601717606)) ;
#69790=CARTESIAN_POINT('',(199.088527625409,547.972556589214,-40.5221601717606)) ;
#69791=CARTESIAN_POINT('',(212.588527625414,573.54800593993,-40.5221601717612)) ;
#69792=CARTESIAN_POINT('',(202.463527625414,573.548005939937,-40.5221601717608)) ;
#69793=CARTESIAN_POINT('',(212.588527625412,565.3971072385,-40.5221601717612)) ;
#69794=CARTESIAN_POINT('',(212.588527625409,547.972556589211,-40.5221601717612)) ;
#69795=CARTESIAN_POINT('',(209.213527625412,565.397107238496,-40.5221601717611)) ;
#69796=CARTESIAN_POINT('',(202.262277625405,570.357556589212,-40.5221601717608)) ;
#69797=CARTESIAN_POINT('',(201.559777625406,570.357556589212,-40.5221601717607)) ;
#69798=CARTESIAN_POINT('',(212.018652625408,570.357556589212,-40.5221601717612)) ;
#69799=CARTESIAN_POINT('',(201.184777625406,569.982556589212,-40.5221601717607)) ;
#69800=CARTESIAN_POINT('Origin',(201.559777625406,569.982556589212,-40.5221601717607)) ;
#69801=CARTESIAN_POINT('',(201.184777625406,568.962556589212,-40.5221601717607)) ;
#69802=CARTESIAN_POINT('',(201.184777625406,586.170681589212,-40.5221601717607)) ;
#69803=CARTESIAN_POINT('',(201.559777625406,568.587556589212,-40.5221601717607)) ;
#69804=CARTESIAN_POINT('Origin',(201.559777625406,568.962556589212,-40.5221601717607)) ;
#69805=CARTESIAN_POINT('',(202.262277625405,568.587556589212,-40.5221601717608)) ;
#69806=CARTESIAN_POINT('',(212.844152625408,568.587556589212,-40.5221601717612)) ;
#69807=CARTESIAN_POINT('',(202.637277625405,568.962556589212,-40.5221601717608)) ;
#69808=CARTESIAN_POINT('Origin',(202.262277625405,568.962556589212,-40.5221601717608)) ;
#69809=CARTESIAN_POINT('',(202.637277625405,569.982556589212,-40.5221601717608)) ;
#69810=CARTESIAN_POINT('',(202.637277625405,586.170681589213,-40.5221601717608)) ;
#69811=CARTESIAN_POINT('Origin',(202.262277625405,569.982556589212,-40.5221601717608)) ;
#69812=CARTESIAN_POINT('Origin',(206.038527625412,559.972556589211,-40.3971601717609)) ;
#69813=CARTESIAN_POINT('',(207.538527625412,559.972556589211,-40.397160171761)) ;
#69814=CARTESIAN_POINT('Origin',(206.038527625412,559.972556589211,-40.3971601717609)) ;
#69815=CARTESIAN_POINT('',(207.663527625412,559.972556589211,-40.522160171761)) ;
#69816=CARTESIAN_POINT('Origin',(207.663527625412,559.972556589211,-40.397160171761)) ;
#69817=CARTESIAN_POINT('Origin',(206.038527625412,559.972556589211,-40.5221601717609)) ;
#69818=CARTESIAN_POINT('Origin',(206.038527625413,559.972556589211,-29.1521601717607)) ;
#69819=CARTESIAN_POINT('',(207.538527625412,559.972556589211,-37.0052690928546)) ;
#69820=CARTESIAN_POINT('Origin',(206.038527625412,559.972556589211,-37.0052690928546)) ;
#69821=CARTESIAN_POINT('',(207.538527625413,559.972556589211,-29.1521601717608)) ;
#69822=CARTESIAN_POINT('Origin',(205.838527625413,569.472556589214,-40.5221601717609)) ;
#69823=CARTESIAN_POINT('',(199.088527625412,564.048005939932,-40.5221601717606)) ;
#69824=CARTESIAN_POINT('',(199.088527625411,555.897107238502,-40.5221601717606)) ;
#69825=CARTESIAN_POINT('',(199.088527625409,547.972556589214,-40.5221601717606)) ;
#69826=CARTESIAN_POINT('',(212.588527625412,564.04800593993,-40.5221601717612)) ;
#69827=CARTESIAN_POINT('',(202.463527625412,564.04800593993,-40.5221601717608)) ;
#69828=CARTESIAN_POINT('',(212.588527625411,555.8971072385,-40.5221601717612)) ;
#69829=CARTESIAN_POINT('',(212.588527625409,547.972556589211,-40.5221601717612)) ;
#69830=CARTESIAN_POINT('',(209.213527625411,555.897107238496,-40.5221601717611)) ;
#69831=CARTESIAN_POINT('',(202.262277625406,560.857556589212,-40.5221601717608)) ;
#69832=CARTESIAN_POINT('',(201.559777625406,560.857556589212,-40.5221601717607)) ;
#69833=CARTESIAN_POINT('',(212.018652625409,560.857556589212,-40.5221601717612)) ;
#69834=CARTESIAN_POINT('',(201.184777625406,560.482556589212,-40.5221601717607)) ;
#69835=CARTESIAN_POINT('Origin',(201.559777625406,560.482556589212,-40.5221601717607)) ;
#69836=CARTESIAN_POINT('',(201.184777625406,559.462556589212,-40.5221601717607)) ;
#69837=CARTESIAN_POINT('',(201.184777625406,576.670681589212,-40.5221601717607)) ;
#69838=CARTESIAN_POINT('',(201.559777625406,559.087556589212,-40.5221601717607)) ;
#69839=CARTESIAN_POINT('Origin',(201.559777625406,559.462556589212,-40.5221601717607)) ;
#69840=CARTESIAN_POINT('',(202.262277625406,559.087556589212,-40.5221601717608)) ;
#69841=CARTESIAN_POINT('',(212.844152625408,559.087556589212,-40.5221601717612)) ;
#69842=CARTESIAN_POINT('',(202.637277625406,559.462556589212,-40.5221601717608)) ;
#69843=CARTESIAN_POINT('Origin',(202.262277625406,559.462556589212,-40.5221601717608)) ;
#69844=CARTESIAN_POINT('',(202.637277625406,560.482556589212,-40.5221601717608)) ;
#69845=CARTESIAN_POINT('',(202.637277625406,576.670681589213,-40.5221601717608)) ;
#69846=CARTESIAN_POINT('Origin',(202.262277625406,560.482556589212,-40.5221601717608)) ;
#69847=CARTESIAN_POINT('Origin',(206.03852762541,550.472556589211,-40.3971601717609)) ;
#69848=CARTESIAN_POINT('',(207.53852762541,550.47255658921,-40.397160171761)) ;
#69849=CARTESIAN_POINT('Origin',(206.03852762541,550.472556589211,-40.3971601717609)) ;
#69850=CARTESIAN_POINT('',(207.66352762541,550.47255658921,-40.522160171761)) ;
#69851=CARTESIAN_POINT('Origin',(207.66352762541,550.472556589211,-40.397160171761)) ;
#69852=CARTESIAN_POINT('Origin',(206.03852762541,550.472556589211,-40.5221601717609)) ;
#69853=CARTESIAN_POINT('Origin',(206.038527625411,550.472556589211,-29.1521601717607)) ;
#69854=CARTESIAN_POINT('',(207.53852762541,550.47255658921,-37.0052690928546)) ;
#69855=CARTESIAN_POINT('Origin',(206.038527625411,550.472556589211,-37.0052690928546)) ;
#69856=CARTESIAN_POINT('',(207.538527625411,550.472556589211,-29.1521601717608)) ;
#69857=CARTESIAN_POINT('Origin',(205.838527625413,569.472556589214,-40.5221601717609)) ;
#69858=CARTESIAN_POINT('',(199.088527625411,554.548005939932,-40.5221601717606)) ;
#69859=CARTESIAN_POINT('',(199.088527625409,546.397107238502,-40.5221601717606)) ;
#69860=CARTESIAN_POINT('',(199.088527625409,547.972556589214,-40.5221601717606)) ;
#69861=CARTESIAN_POINT('',(212.588527625411,554.54800593993,-40.5221601717612)) ;
#69862=CARTESIAN_POINT('',(202.463527625411,554.54800593993,-40.5221601717608)) ;
#69863=CARTESIAN_POINT('',(212.588527625409,546.3971072385,-40.5221601717612)) ;
#69864=CARTESIAN_POINT('',(212.588527625409,547.972556589211,-40.5221601717612)) ;
#69865=CARTESIAN_POINT('',(209.213527625409,546.397107238496,-40.5221601717611)) ;
#69866=CARTESIAN_POINT('',(202.262277625406,551.357556589212,-40.5221601717608)) ;
#69867=CARTESIAN_POINT('',(201.559777625406,551.357556589212,-40.5221601717607)) ;
#69868=CARTESIAN_POINT('',(212.018652625409,551.357556589212,-40.5221601717612)) ;
#69869=CARTESIAN_POINT('',(201.184777625406,550.982556589212,-40.5221601717607)) ;
#69870=CARTESIAN_POINT('Origin',(201.559777625406,550.982556589212,-40.5221601717607)) ;
#69871=CARTESIAN_POINT('',(201.184777625406,549.962556589212,-40.5221601717607)) ;
#69872=CARTESIAN_POINT('',(201.184777625406,567.170681589212,-40.5221601717607)) ;
#69873=CARTESIAN_POINT('',(201.559777625407,549.587556589212,-40.5221601717607)) ;
#69874=CARTESIAN_POINT('Origin',(201.559777625406,549.962556589212,-40.5221601717607)) ;
#69875=CARTESIAN_POINT('',(202.262277625406,549.587556589212,-40.5221601717608)) ;
#69876=CARTESIAN_POINT('',(212.844152625409,549.587556589212,-40.5221601717612)) ;
#69877=CARTESIAN_POINT('',(202.637277625406,549.962556589212,-40.5221601717608)) ;
#69878=CARTESIAN_POINT('Origin',(202.262277625406,549.962556589212,-40.5221601717608)) ;
#69879=CARTESIAN_POINT('',(202.637277625406,550.982556589212,-40.5221601717608)) ;
#69880=CARTESIAN_POINT('',(202.637277625406,567.170681589213,-40.5221601717608)) ;
#69881=CARTESIAN_POINT('Origin',(202.262277625406,550.982556589212,-40.5221601717608)) ;
#69882=CARTESIAN_POINT('Origin',(206.038527625409,540.972556589211,-40.3971601717609)) ;
#69883=CARTESIAN_POINT('',(207.538527625409,540.97255658921,-40.397160171761)) ;
#69884=CARTESIAN_POINT('Origin',(206.038527625409,540.972556589211,-40.3971601717609)) ;
#69885=CARTESIAN_POINT('',(207.663527625409,540.97255658921,-40.522160171761)) ;
#69886=CARTESIAN_POINT('Origin',(207.663527625409,540.972556589211,-40.397160171761)) ;
#69887=CARTESIAN_POINT('Origin',(206.038527625409,540.972556589211,-40.5221601717609)) ;
#69888=CARTESIAN_POINT('Origin',(206.038527625409,540.972556589211,-29.1521601717607)) ;
#69889=CARTESIAN_POINT('',(207.538527625409,540.97255658921,-37.0052690928546)) ;
#69890=CARTESIAN_POINT('Origin',(206.038527625409,540.972556589211,-37.0052690928546)) ;
#69891=CARTESIAN_POINT('',(207.538527625409,540.972556589211,-29.1521601717608)) ;
#69892=CARTESIAN_POINT('Origin',(205.838527625413,569.472556589214,-40.5221601717609)) ;
#69893=CARTESIAN_POINT('',(199.088527625409,545.048005939932,-40.5221601717606)) ;
#69894=CARTESIAN_POINT('',(199.088527625407,536.897107238502,-40.5221601717606)) ;
#69895=CARTESIAN_POINT('',(199.088527625409,547.972556589214,-40.5221601717606)) ;
#69896=CARTESIAN_POINT('',(212.588527625409,545.04800593993,-40.5221601717612)) ;
#69897=CARTESIAN_POINT('',(202.463527625409,545.04800593993,-40.5221601717608)) ;
#69898=CARTESIAN_POINT('',(212.588527625407,536.8971072385,-40.5221601717612)) ;
#69899=CARTESIAN_POINT('',(212.588527625409,547.972556589211,-40.5221601717612)) ;
#69900=CARTESIAN_POINT('',(209.213527625407,536.897107238496,-40.5221601717611)) ;
#69901=CARTESIAN_POINT('',(202.262277625406,541.857556589212,-40.5221601717608)) ;
#69902=CARTESIAN_POINT('',(201.559777625407,541.857556589212,-40.5221601717607)) ;
#69903=CARTESIAN_POINT('',(212.018652625409,541.857556589212,-40.5221601717612)) ;
#69904=CARTESIAN_POINT('',(201.184777625407,541.482556589212,-40.5221601717607)) ;
#69905=CARTESIAN_POINT('Origin',(201.559777625407,541.482556589212,-40.5221601717607)) ;
#69906=CARTESIAN_POINT('',(201.184777625407,540.462556589212,-40.5221601717607)) ;
#69907=CARTESIAN_POINT('',(201.184777625407,557.670681589212,-40.5221601717607)) ;
#69908=CARTESIAN_POINT('',(201.559777625407,540.087556589212,-40.5221601717607)) ;
#69909=CARTESIAN_POINT('Origin',(201.559777625407,540.462556589212,-40.5221601717607)) ;
#69910=CARTESIAN_POINT('',(202.262277625406,540.087556589212,-40.5221601717608)) ;
#69911=CARTESIAN_POINT('',(212.844152625409,540.087556589212,-40.5221601717612)) ;
#69912=CARTESIAN_POINT('',(202.637277625406,540.462556589212,-40.5221601717608)) ;
#69913=CARTESIAN_POINT('Origin',(202.262277625406,540.462556589212,-40.5221601717608)) ;
#69914=CARTESIAN_POINT('',(202.637277625406,541.482556589212,-40.5221601717608)) ;
#69915=CARTESIAN_POINT('',(202.637277625406,557.670681589212,-40.5221601717608)) ;
#69916=CARTESIAN_POINT('Origin',(202.262277625406,541.482556589212,-40.5221601717608)) ;
#69917=CARTESIAN_POINT('Origin',(206.038527625407,531.472556589211,-40.3971601717609)) ;
#69918=CARTESIAN_POINT('',(207.538527625407,531.47255658921,-40.397160171761)) ;
#69919=CARTESIAN_POINT('Origin',(206.038527625407,531.472556589211,-40.3971601717609)) ;
#69920=CARTESIAN_POINT('',(207.663527625407,531.47255658921,-40.522160171761)) ;
#69921=CARTESIAN_POINT('Origin',(207.663527625407,531.472556589211,-40.397160171761)) ;
#69922=CARTESIAN_POINT('Origin',(206.038527625407,531.472556589211,-40.5221601717609)) ;
#69923=CARTESIAN_POINT('Origin',(205.838527625413,569.472556589214,-40.5221601717609)) ;
#69924=CARTESIAN_POINT('',(199.088527625407,535.548005939932,-40.5221601717606)) ;
#69925=CARTESIAN_POINT('',(199.088527625406,527.397107238502,-40.5221601717606)) ;
#69926=CARTESIAN_POINT('',(199.088527625409,547.972556589214,-40.5221601717606)) ;
#69927=CARTESIAN_POINT('',(212.588527625407,535.54800593993,-40.5221601717612)) ;
#69928=CARTESIAN_POINT('',(202.463527625407,535.54800593993,-40.5221601717608)) ;
#69929=CARTESIAN_POINT('',(212.588527625406,527.3971072385,-40.5221601717612)) ;
#69930=CARTESIAN_POINT('',(212.588527625409,547.972556589211,-40.5221601717612)) ;
#69931=CARTESIAN_POINT('',(209.213527625406,527.397107238496,-40.5221601717611)) ;
#69932=CARTESIAN_POINT('',(201.559777625407,532.357556589212,-40.5221601717607)) ;
#69933=CARTESIAN_POINT('',(202.262277625407,532.357556589212,-40.5221601717608)) ;
#69934=CARTESIAN_POINT('',(212.01865262541,532.357556589212,-40.5221601717612)) ;
#69935=CARTESIAN_POINT('',(201.184777625407,531.982556589212,-40.5221601717607)) ;
#69936=CARTESIAN_POINT('Origin',(201.559777625407,531.982556589212,-40.5221601717607)) ;
#69937=CARTESIAN_POINT('',(201.184777625407,530.962556589212,-40.5221601717607)) ;
#69938=CARTESIAN_POINT('',(201.184777625407,548.170681589212,-40.5221601717607)) ;
#69939=CARTESIAN_POINT('',(201.559777625407,530.587556589212,-40.5221601717607)) ;
#69940=CARTESIAN_POINT('Origin',(201.559777625407,530.962556589212,-40.5221601717607)) ;
#69941=CARTESIAN_POINT('',(202.262277625407,530.587556589212,-40.5221601717608)) ;
#69942=CARTESIAN_POINT('',(212.844152625409,530.587556589212,-40.5221601717613)) ;
#69943=CARTESIAN_POINT('',(202.637277625407,530.962556589212,-40.5221601717608)) ;
#69944=CARTESIAN_POINT('Origin',(202.262277625407,530.962556589212,-40.5221601717608)) ;
#69945=CARTESIAN_POINT('',(202.637277625407,531.982556589212,-40.5221601717608)) ;
#69946=CARTESIAN_POINT('',(202.637277625407,548.170681589212,-40.5221601717608)) ;
#69947=CARTESIAN_POINT('Origin',(202.262277625407,531.982556589212,-40.5221601717608)) ;
#69948=CARTESIAN_POINT('Origin',(206.038527625407,531.472556589211,-29.1521601717607)) ;
#69949=CARTESIAN_POINT('',(207.538527625407,531.47255658921,-37.0052690928546)) ;
#69950=CARTESIAN_POINT('Origin',(206.038527625407,531.472556589211,-37.0052690928546)) ;
#69951=CARTESIAN_POINT('',(207.538527625407,531.472556589211,-29.1521601717608)) ;
#69952=CARTESIAN_POINT('Origin',(202.466652625407,535.044431589211,-37.0052690928544)) ;
#69953=CARTESIAN_POINT('',(208.77102762542,607.472556589211,-37.0052690928544)) ;
#69954=CARTESIAN_POINT('Origin',(206.03852762542,607.472556589211,-37.0052690928544)) ;
#69955=CARTESIAN_POINT('Origin',(202.466652625407,535.044431589211,-37.0052690928544)) ;
#69956=CARTESIAN_POINT('',(208.771027625418,597.972556589211,-37.0052690928544)) ;
#69957=CARTESIAN_POINT('Origin',(206.038527625418,597.972556589211,-37.0052690928544)) ;
#69958=CARTESIAN_POINT('Origin',(202.466652625407,535.044431589211,-37.0052690928544)) ;
#69959=CARTESIAN_POINT('',(208.771027625417,588.472556589211,-37.0052690928544)) ;
#69960=CARTESIAN_POINT('Origin',(206.038527625417,588.472556589211,-37.0052690928544)) ;
#69961=CARTESIAN_POINT('Origin',(202.466652625407,535.044431589211,-37.0052690928544)) ;
#69962=CARTESIAN_POINT('',(208.771027625415,578.972556589211,-37.0052690928544)) ;
#69963=CARTESIAN_POINT('Origin',(206.038527625415,578.972556589211,-37.0052690928544)) ;
#69964=CARTESIAN_POINT('Origin',(202.466652625407,535.044431589211,-37.0052690928544)) ;
#69965=CARTESIAN_POINT('',(208.771027625413,569.472556589211,-37.0052690928544)) ;
#69966=CARTESIAN_POINT('Origin',(206.038527625413,569.472556589211,-37.0052690928544)) ;
#69967=CARTESIAN_POINT('Origin',(202.466652625407,535.044431589211,-37.0052690928544)) ;
#69968=CARTESIAN_POINT('',(208.771027625412,559.972556589211,-37.0052690928544)) ;
#69969=CARTESIAN_POINT('Origin',(206.038527625412,559.972556589211,-37.0052690928544)) ;
#69970=CARTESIAN_POINT('Origin',(202.466652625407,535.044431589211,-37.0052690928544)) ;
#69971=CARTESIAN_POINT('',(208.77102762541,550.472556589211,-37.0052690928544)) ;
#69972=CARTESIAN_POINT('Origin',(206.03852762541,550.472556589211,-37.0052690928544)) ;
#69973=CARTESIAN_POINT('Origin',(202.466652625407,535.044431589211,-37.0052690928544)) ;
#69974=CARTESIAN_POINT('',(208.771027625408,540.972556589211,-37.0052690928544)) ;
#69975=CARTESIAN_POINT('Origin',(206.038527625408,540.972556589211,-37.0052690928544)) ;
#69976=CARTESIAN_POINT('Origin',(212.018652625407,608.357556589212,-40.2721601717612)) ;
#69977=CARTESIAN_POINT('',(202.262277625404,608.107556589212,-40.2721601717608)) ;
#69978=CARTESIAN_POINT('Origin',(202.262277625404,608.357556589212,-40.2721601717608)) ;
#69979=CARTESIAN_POINT('',(201.559777625404,608.107556589212,-40.2721601717607)) ;
#69980=CARTESIAN_POINT('',(212.018652625407,608.107556589212,-40.2721601717612)) ;
#69981=CARTESIAN_POINT('Origin',(201.559777625404,608.357556589212,-40.2721601717607)) ;
#69982=CARTESIAN_POINT('Origin',(201.559777625404,607.982556589212,-40.2721601717609)) ;
#69983=CARTESIAN_POINT('',(201.434777625404,607.982556589212,-40.2721601717609)) ;
#69984=CARTESIAN_POINT('Origin',(201.184777625404,607.982556589212,-40.2721601717609)) ;
#69985=CARTESIAN_POINT('Origin',(201.559777625404,607.982556589212,-40.2721601717609)) ;
#69986=CARTESIAN_POINT('Origin',(201.184777625405,624.170681589212,-40.2721601717607)) ;
#69987=CARTESIAN_POINT('',(201.434777625404,606.962556589212,-40.2721601717607)) ;
#69988=CARTESIAN_POINT('Origin',(201.184777625405,606.962556589212,-40.2721601717607)) ;
#69989=CARTESIAN_POINT('',(201.43477762542,624.170681589212,-40.2721601717607)) ;
#69990=CARTESIAN_POINT('Origin',(201.559777625404,606.962556589212,-40.2721601717609)) ;
#69991=CARTESIAN_POINT('',(201.559777625405,606.837556589212,-40.2721601717609)) ;
#69992=CARTESIAN_POINT('Origin',(201.559777625405,606.587556589212,-40.2721601717609)) ;
#69993=CARTESIAN_POINT('Origin',(201.559777625404,606.962556589212,-40.2721601717609)) ;
#69994=CARTESIAN_POINT('Origin',(212.844152625407,606.587556589212,-40.2721601717612)) ;
#69995=CARTESIAN_POINT('',(202.262277625404,606.837556589212,-40.2721601717608)) ;
#69996=CARTESIAN_POINT('Origin',(202.262277625404,606.587556589212,-40.2721601717608)) ;
#69997=CARTESIAN_POINT('',(212.844152625407,606.837556589212,-40.2721601717612)) ;
#69998=CARTESIAN_POINT('Origin',(202.262277625404,606.962556589212,-40.2721601717609)) ;
#69999=CARTESIAN_POINT('',(202.387277625404,606.962556589212,-40.2721601717609)) ;
#70000=CARTESIAN_POINT('Origin',(202.637277625404,606.962556589212,-40.2721601717609)) ;
#70001=CARTESIAN_POINT('Origin',(202.262277625404,606.962556589212,-40.2721601717609)) ;
#70002=CARTESIAN_POINT('Origin',(202.637277625404,624.170681589213,-40.2721601717608)) ;
#70003=CARTESIAN_POINT('',(202.387277625404,607.982556589212,-40.2721601717608)) ;
#70004=CARTESIAN_POINT('Origin',(202.637277625404,607.982556589212,-40.2721601717608)) ;
#70005=CARTESIAN_POINT('',(202.38727762542,624.170681589213,-40.2721601717608)) ;
#70006=CARTESIAN_POINT('Origin',(202.262277625404,607.982556589212,-40.2721601717609)) ;
#70007=CARTESIAN_POINT('Origin',(202.262277625404,607.982556589212,-40.2721601717609)) ;
#70008=CARTESIAN_POINT('Origin',(201.55977762542,606.962556589212,-42.3117150424525)) ;
#70009=CARTESIAN_POINT('',(201.43477762542,606.962556589212,-39.4182700580611)) ;
#70010=CARTESIAN_POINT('',(201.43477762542,606.962556589212,-42.3117150424525)) ;
#70011=CARTESIAN_POINT('',(201.55977762542,606.837556589212,-39.4182700580611)) ;
#70012=CARTESIAN_POINT('Origin',(201.55977762542,606.962556589212,-39.4182700580611)) ;
#70013=CARTESIAN_POINT('',(201.55977762542,606.837556589212,-42.3117150424525)) ;
#70014=CARTESIAN_POINT('Origin',(201.43477762542,602.868806589211,-43.1012690928543)) ;
#70015=CARTESIAN_POINT('',(201.43477762542,607.982556589212,-39.4182700580611)) ;
#70016=CARTESIAN_POINT('',(201.43477762542,607.982556589212,-44.5342150424525)) ;
#70017=CARTESIAN_POINT('',(201.43477762542,608.171056589212,-39.2297700580612)) ;
#70018=CARTESIAN_POINT('Origin',(201.43477762542,608.171056589212,-39.4182700580612)) ;
#70019=CARTESIAN_POINT('',(201.43477762542,609.347556589211,-39.2297700580612)) ;
#70020=CARTESIAN_POINT('',(201.43477762542,605.488181589211,-39.2297700580612)) ;
#70021=CARTESIAN_POINT('',(201.434777625407,609.347556589211,-35.2721601717607)) ;
#70022=CARTESIAN_POINT('',(201.43477762542,609.347556589211,-38.5610190928544)) ;
#70023=CARTESIAN_POINT('',(201.434777625407,605.597556589211,-35.2721601717609)) ;
#70024=CARTESIAN_POINT('',(201.43477762542,624.170681589221,-35.2721601717607)) ;
#70025=CARTESIAN_POINT('',(201.43477762542,605.597556589211,-39.2297700580612)) ;
#70026=CARTESIAN_POINT('',(201.43477762542,605.597556589211,-40.5297040214914)) ;
#70027=CARTESIAN_POINT('',(201.43477762542,606.774056589212,-39.2297700580612)) ;
#70028=CARTESIAN_POINT('',(201.43477762542,605.488181589211,-39.2297700580612)) ;
#70029=CARTESIAN_POINT('Origin',(201.43477762542,606.774056589212,-39.4182700580611)) ;
#70030=CARTESIAN_POINT('Origin',(201.55977762542,607.982556589212,-44.5342150424525)) ;
#70031=CARTESIAN_POINT('',(201.55977762542,608.107556589212,-39.4182700580612)) ;
#70032=CARTESIAN_POINT('',(201.55977762542,608.107556589212,-44.5342150424525)) ;
#70033=CARTESIAN_POINT('Origin',(201.55977762542,607.982556589212,-39.4182700580611)) ;
#70034=CARTESIAN_POINT('Origin',(218.198777625419,608.107556589212,-45.9671609920506)) ;
#70035=CARTESIAN_POINT('',(202.26227762542,608.107556589212,-39.4182700580612)) ;
#70036=CARTESIAN_POINT('',(202.26227762542,608.107556589212,-39.8669650424525)) ;
#70037=CARTESIAN_POINT('',(218.198777625419,608.107556589212,-39.4182700580611)) ;
#70038=CARTESIAN_POINT('Origin',(212.018652625407,598.857556589212,-40.2721601717612)) ;
#70039=CARTESIAN_POINT('',(202.262277625404,598.607556589212,-40.2721601717608)) ;
#70040=CARTESIAN_POINT('Origin',(202.262277625404,598.857556589212,-40.2721601717608)) ;
#70041=CARTESIAN_POINT('',(201.559777625405,598.607556589212,-40.2721601717607)) ;
#70042=CARTESIAN_POINT('',(212.018652625407,598.607556589212,-40.2721601717612)) ;
#70043=CARTESIAN_POINT('Origin',(201.559777625405,598.857556589212,-40.2721601717607)) ;
#70044=CARTESIAN_POINT('Origin',(201.559777625405,598.482556589212,-40.2721601717609)) ;
#70045=CARTESIAN_POINT('',(201.434777625405,598.482556589212,-40.2721601717609)) ;
#70046=CARTESIAN_POINT('Origin',(201.184777625405,598.482556589212,-40.2721601717609)) ;
#70047=CARTESIAN_POINT('Origin',(201.559777625405,598.482556589212,-40.2721601717609)) ;
#70048=CARTESIAN_POINT('Origin',(201.184777625405,614.670681589212,-40.2721601717607)) ;
#70049=CARTESIAN_POINT('',(201.434777625405,597.462556589212,-40.2721601717607)) ;
#70050=CARTESIAN_POINT('Origin',(201.184777625405,597.462556589212,-40.2721601717607)) ;
#70051=CARTESIAN_POINT('',(201.434777625419,614.670681589212,-40.2721601717607)) ;
#70052=CARTESIAN_POINT('Origin',(201.559777625405,597.462556589212,-40.2721601717609)) ;
#70053=CARTESIAN_POINT('',(201.559777625405,597.337556589212,-40.2721601717609)) ;
#70054=CARTESIAN_POINT('Origin',(201.559777625405,597.087556589212,-40.2721601717609)) ;
#70055=CARTESIAN_POINT('Origin',(201.559777625405,597.462556589212,-40.2721601717609)) ;
#70056=CARTESIAN_POINT('Origin',(212.844152625407,597.087556589212,-40.2721601717612)) ;
#70057=CARTESIAN_POINT('',(202.262277625404,597.337556589212,-40.2721601717608)) ;
#70058=CARTESIAN_POINT('Origin',(202.262277625404,597.087556589212,-40.2721601717608)) ;
#70059=CARTESIAN_POINT('',(212.844152625407,597.337556589212,-40.2721601717612)) ;
#70060=CARTESIAN_POINT('Origin',(202.262277625404,597.462556589212,-40.2721601717609)) ;
#70061=CARTESIAN_POINT('',(202.387277625404,597.462556589212,-40.2721601717609)) ;
#70062=CARTESIAN_POINT('Origin',(202.637277625404,597.462556589212,-40.2721601717609)) ;
#70063=CARTESIAN_POINT('Origin',(202.262277625404,597.462556589212,-40.2721601717609)) ;
#70064=CARTESIAN_POINT('Origin',(202.637277625404,614.670681589213,-40.2721601717608)) ;
#70065=CARTESIAN_POINT('',(202.387277625404,598.482556589212,-40.2721601717608)) ;
#70066=CARTESIAN_POINT('Origin',(202.637277625404,598.482556589212,-40.2721601717608)) ;
#70067=CARTESIAN_POINT('',(202.387277625418,614.670681589213,-40.2721601717608)) ;
#70068=CARTESIAN_POINT('Origin',(202.262277625404,598.482556589212,-40.2721601717609)) ;
#70069=CARTESIAN_POINT('Origin',(202.262277625404,598.482556589212,-40.2721601717609)) ;
#70070=CARTESIAN_POINT('Origin',(201.559777625419,597.462556589212,-42.3117150424525)) ;
#70071=CARTESIAN_POINT('',(201.434777625419,597.462556589212,-39.4182700580611)) ;
#70072=CARTESIAN_POINT('',(201.434777625419,597.462556589212,-42.3117150424525)) ;
#70073=CARTESIAN_POINT('',(201.559777625419,597.337556589212,-39.4182700580611)) ;
#70074=CARTESIAN_POINT('Origin',(201.559777625419,597.462556589212,-39.4182700580611)) ;
#70075=CARTESIAN_POINT('',(201.559777625419,597.337556589212,-42.3117150424525)) ;
#70076=CARTESIAN_POINT('Origin',(201.434777625419,593.368806589211,-43.1012690928543)) ;
#70077=CARTESIAN_POINT('',(201.434777625419,598.482556589212,-39.4182700580611)) ;
#70078=CARTESIAN_POINT('',(201.434777625419,598.482556589212,-44.5342150424525)) ;
#70079=CARTESIAN_POINT('',(201.434777625419,598.671056589212,-39.2297700580612)) ;
#70080=CARTESIAN_POINT('Origin',(201.434777625419,598.671056589212,-39.4182700580612)) ;
#70081=CARTESIAN_POINT('',(201.434777625419,599.847556589211,-39.2297700580612)) ;
#70082=CARTESIAN_POINT('',(201.434777625419,595.988181589211,-39.2297700580612)) ;
#70083=CARTESIAN_POINT('',(201.434777625407,599.847556589211,-35.2721601717607)) ;
#70084=CARTESIAN_POINT('',(201.434777625419,599.847556589211,-38.5610190928544)) ;
#70085=CARTESIAN_POINT('',(201.434777625407,596.097556589211,-35.2721601717609)) ;
#70086=CARTESIAN_POINT('',(201.434777625419,614.670681589221,-35.2721601717607)) ;
#70087=CARTESIAN_POINT('',(201.434777625419,596.097556589211,-39.2297700580612)) ;
#70088=CARTESIAN_POINT('',(201.434777625419,596.097556589211,-40.5297040214914)) ;
#70089=CARTESIAN_POINT('',(201.434777625419,597.274056589212,-39.2297700580612)) ;
#70090=CARTESIAN_POINT('',(201.434777625419,595.988181589211,-39.2297700580612)) ;
#70091=CARTESIAN_POINT('Origin',(201.434777625419,597.274056589212,-39.4182700580611)) ;
#70092=CARTESIAN_POINT('Origin',(201.559777625419,598.482556589212,-44.5342150424525)) ;
#70093=CARTESIAN_POINT('',(201.559777625419,598.607556589212,-39.4182700580612)) ;
#70094=CARTESIAN_POINT('',(201.559777625419,598.607556589212,-44.5342150424525)) ;
#70095=CARTESIAN_POINT('Origin',(201.559777625419,598.482556589212,-39.4182700580611)) ;
#70096=CARTESIAN_POINT('Origin',(218.198777625417,598.607556589212,-45.9671609920506)) ;
#70097=CARTESIAN_POINT('',(202.262277625418,598.607556589212,-39.4182700580612)) ;
#70098=CARTESIAN_POINT('',(202.262277625418,598.607556589212,-39.8669650424525)) ;
#70099=CARTESIAN_POINT('',(218.198777625418,598.607556589212,-39.4182700580611)) ;
#70100=CARTESIAN_POINT('Origin',(212.018652625408,589.357556589212,-40.2721601717612)) ;
#70101=CARTESIAN_POINT('',(202.262277625405,589.107556589212,-40.2721601717608)) ;
#70102=CARTESIAN_POINT('Origin',(202.262277625405,589.357556589212,-40.2721601717608)) ;
#70103=CARTESIAN_POINT('',(201.559777625405,589.107556589212,-40.2721601717607)) ;
#70104=CARTESIAN_POINT('',(212.018652625408,589.107556589212,-40.2721601717612)) ;
#70105=CARTESIAN_POINT('Origin',(201.559777625405,589.357556589212,-40.2721601717607)) ;
#70106=CARTESIAN_POINT('Origin',(201.559777625405,588.982556589212,-40.2721601717609)) ;
#70107=CARTESIAN_POINT('',(201.434777625405,588.982556589212,-40.2721601717609)) ;
#70108=CARTESIAN_POINT('Origin',(201.184777625405,588.982556589212,-40.2721601717609)) ;
#70109=CARTESIAN_POINT('Origin',(201.559777625405,588.982556589212,-40.2721601717609)) ;
#70110=CARTESIAN_POINT('Origin',(201.184777625405,605.170681589212,-40.2721601717607)) ;
#70111=CARTESIAN_POINT('',(201.434777625405,587.962556589212,-40.2721601717607)) ;
#70112=CARTESIAN_POINT('Origin',(201.184777625405,587.962556589212,-40.2721601717607)) ;
#70113=CARTESIAN_POINT('',(201.434777625417,605.170681589212,-40.2721601717607)) ;
#70114=CARTESIAN_POINT('Origin',(201.559777625405,587.962556589212,-40.2721601717609)) ;
#70115=CARTESIAN_POINT('',(201.559777625405,587.837556589212,-40.2721601717609)) ;
#70116=CARTESIAN_POINT('Origin',(201.559777625405,587.587556589212,-40.2721601717609)) ;
#70117=CARTESIAN_POINT('Origin',(201.559777625405,587.962556589212,-40.2721601717609)) ;
#70118=CARTESIAN_POINT('Origin',(212.844152625407,587.587556589212,-40.2721601717612)) ;
#70119=CARTESIAN_POINT('',(202.262277625405,587.837556589212,-40.2721601717608)) ;
#70120=CARTESIAN_POINT('Origin',(202.262277625405,587.587556589212,-40.2721601717608)) ;
#70121=CARTESIAN_POINT('',(212.844152625408,587.837556589212,-40.2721601717612)) ;
#70122=CARTESIAN_POINT('Origin',(202.262277625405,587.962556589212,-40.2721601717609)) ;
#70123=CARTESIAN_POINT('',(202.387277625405,587.962556589212,-40.2721601717609)) ;
#70124=CARTESIAN_POINT('Origin',(202.637277625405,587.962556589212,-40.2721601717609)) ;
#70125=CARTESIAN_POINT('Origin',(202.262277625405,587.962556589212,-40.2721601717609)) ;
#70126=CARTESIAN_POINT('Origin',(202.637277625405,605.170681589213,-40.2721601717608)) ;
#70127=CARTESIAN_POINT('',(202.387277625405,588.982556589212,-40.2721601717608)) ;
#70128=CARTESIAN_POINT('Origin',(202.637277625405,588.982556589212,-40.2721601717608)) ;
#70129=CARTESIAN_POINT('',(202.387277625417,605.170681589213,-40.2721601717608)) ;
#70130=CARTESIAN_POINT('Origin',(202.262277625405,588.982556589212,-40.2721601717609)) ;
#70131=CARTESIAN_POINT('Origin',(202.262277625405,588.982556589212,-40.2721601717609)) ;
#70132=CARTESIAN_POINT('Origin',(201.559777625417,587.962556589212,-42.3117150424525)) ;
#70133=CARTESIAN_POINT('',(201.434777625417,587.962556589212,-39.4182700580611)) ;
#70134=CARTESIAN_POINT('',(201.434777625417,587.962556589212,-42.3117150424525)) ;
#70135=CARTESIAN_POINT('',(201.559777625417,587.837556589212,-39.4182700580611)) ;
#70136=CARTESIAN_POINT('Origin',(201.559777625417,587.962556589212,-39.4182700580611)) ;
#70137=CARTESIAN_POINT('',(201.559777625417,587.837556589212,-42.3117150424525)) ;
#70138=CARTESIAN_POINT('Origin',(201.434777625417,583.868806589211,-43.1012690928543)) ;
#70139=CARTESIAN_POINT('',(201.434777625417,588.982556589212,-39.4182700580611)) ;
#70140=CARTESIAN_POINT('',(201.434777625417,588.982556589212,-44.5342150424525)) ;
#70141=CARTESIAN_POINT('',(201.434777625417,589.171056589212,-39.2297700580612)) ;
#70142=CARTESIAN_POINT('Origin',(201.434777625417,589.171056589212,-39.4182700580612)) ;
#70143=CARTESIAN_POINT('',(201.434777625417,590.347556589211,-39.2297700580612)) ;
#70144=CARTESIAN_POINT('',(201.434777625417,586.488181589211,-39.2297700580612)) ;
#70145=CARTESIAN_POINT('',(201.434777625407,590.347556589211,-35.2721601717607)) ;
#70146=CARTESIAN_POINT('',(201.434777625417,590.347556589211,-38.5610190928544)) ;
#70147=CARTESIAN_POINT('',(201.434777625407,586.597556589211,-35.2721601717609)) ;
#70148=CARTESIAN_POINT('',(201.434777625417,605.170681589221,-35.2721601717607)) ;
#70149=CARTESIAN_POINT('',(201.434777625417,586.597556589211,-39.2297700580612)) ;
#70150=CARTESIAN_POINT('',(201.434777625417,586.597556589211,-40.5297040214914)) ;
#70151=CARTESIAN_POINT('',(201.434777625417,587.774056589212,-39.2297700580612)) ;
#70152=CARTESIAN_POINT('',(201.434777625417,586.488181589211,-39.2297700580612)) ;
#70153=CARTESIAN_POINT('Origin',(201.434777625417,587.774056589212,-39.4182700580611)) ;
#70154=CARTESIAN_POINT('Origin',(201.559777625417,588.982556589212,-44.5342150424525)) ;
#70155=CARTESIAN_POINT('',(201.559777625417,589.107556589212,-39.4182700580612)) ;
#70156=CARTESIAN_POINT('',(201.559777625417,589.107556589212,-44.5342150424525)) ;
#70157=CARTESIAN_POINT('Origin',(201.559777625417,588.982556589212,-39.4182700580611)) ;
#70158=CARTESIAN_POINT('Origin',(218.198777625415,589.107556589212,-45.9671609920506)) ;
#70159=CARTESIAN_POINT('',(202.262277625416,589.107556589212,-39.4182700580612)) ;
#70160=CARTESIAN_POINT('',(202.262277625416,589.107556589212,-39.8669650424525)) ;
#70161=CARTESIAN_POINT('',(218.198777625416,589.107556589212,-39.4182700580611)) ;
#70162=CARTESIAN_POINT('Origin',(212.018652625408,579.857556589212,-40.2721601717612)) ;
#70163=CARTESIAN_POINT('',(202.262277625405,579.607556589212,-40.2721601717608)) ;
#70164=CARTESIAN_POINT('Origin',(202.262277625405,579.857556589212,-40.2721601717608)) ;
#70165=CARTESIAN_POINT('',(201.559777625405,579.607556589212,-40.2721601717607)) ;
#70166=CARTESIAN_POINT('',(212.018652625408,579.607556589212,-40.2721601717612)) ;
#70167=CARTESIAN_POINT('Origin',(201.559777625405,579.857556589212,-40.2721601717607)) ;
#70168=CARTESIAN_POINT('Origin',(201.559777625405,579.482556589212,-40.2721601717609)) ;
#70169=CARTESIAN_POINT('',(201.434777625406,579.482556589212,-40.2721601717609)) ;
#70170=CARTESIAN_POINT('Origin',(201.184777625405,579.482556589212,-40.2721601717609)) ;
#70171=CARTESIAN_POINT('Origin',(201.559777625405,579.482556589212,-40.2721601717609)) ;
#70172=CARTESIAN_POINT('Origin',(201.184777625406,595.670681589212,-40.2721601717607)) ;
#70173=CARTESIAN_POINT('',(201.434777625406,578.462556589212,-40.2721601717607)) ;
#70174=CARTESIAN_POINT('Origin',(201.184777625406,578.462556589212,-40.2721601717607)) ;
#70175=CARTESIAN_POINT('',(201.434777625415,595.670681589212,-40.2721601717607)) ;
#70176=CARTESIAN_POINT('Origin',(201.559777625405,578.462556589212,-40.2721601717609)) ;
#70177=CARTESIAN_POINT('',(201.559777625406,578.337556589212,-40.2721601717609)) ;
#70178=CARTESIAN_POINT('Origin',(201.559777625406,578.087556589212,-40.2721601717609)) ;
#70179=CARTESIAN_POINT('Origin',(201.559777625405,578.462556589212,-40.2721601717609)) ;
#70180=CARTESIAN_POINT('Origin',(212.844152625408,578.087556589212,-40.2721601717612)) ;
#70181=CARTESIAN_POINT('',(202.262277625405,578.337556589212,-40.2721601717608)) ;
#70182=CARTESIAN_POINT('Origin',(202.262277625405,578.087556589212,-40.2721601717608)) ;
#70183=CARTESIAN_POINT('',(212.844152625408,578.337556589212,-40.2721601717612)) ;
#70184=CARTESIAN_POINT('Origin',(202.262277625405,578.462556589212,-40.2721601717609)) ;
#70185=CARTESIAN_POINT('',(202.387277625405,578.462556589212,-40.2721601717609)) ;
#70186=CARTESIAN_POINT('Origin',(202.637277625405,578.462556589212,-40.2721601717609)) ;
#70187=CARTESIAN_POINT('Origin',(202.262277625405,578.462556589212,-40.2721601717609)) ;
#70188=CARTESIAN_POINT('Origin',(202.637277625405,595.670681589213,-40.2721601717608)) ;
#70189=CARTESIAN_POINT('',(202.387277625405,579.482556589212,-40.2721601717608)) ;
#70190=CARTESIAN_POINT('Origin',(202.637277625405,579.482556589212,-40.2721601717608)) ;
#70191=CARTESIAN_POINT('',(202.387277625415,595.670681589213,-40.2721601717608)) ;
#70192=CARTESIAN_POINT('Origin',(202.262277625405,579.482556589212,-40.2721601717609)) ;
#70193=CARTESIAN_POINT('Origin',(202.262277625405,579.482556589212,-40.2721601717609)) ;
#70194=CARTESIAN_POINT('Origin',(201.559777625415,578.462556589212,-42.3117150424525)) ;
#70195=CARTESIAN_POINT('',(201.434777625415,578.462556589212,-39.4182700580611)) ;
#70196=CARTESIAN_POINT('',(201.434777625415,578.462556589212,-42.3117150424525)) ;
#70197=CARTESIAN_POINT('',(201.559777625416,578.337556589212,-39.4182700580611)) ;
#70198=CARTESIAN_POINT('Origin',(201.559777625415,578.462556589212,-39.4182700580611)) ;
#70199=CARTESIAN_POINT('',(201.559777625416,578.337556589212,-42.3117150424525)) ;
#70200=CARTESIAN_POINT('Origin',(201.434777625415,574.368806589211,-43.1012690928543)) ;
#70201=CARTESIAN_POINT('',(201.434777625415,579.482556589212,-39.4182700580611)) ;
#70202=CARTESIAN_POINT('',(201.434777625415,579.482556589212,-44.5342150424525)) ;
#70203=CARTESIAN_POINT('',(201.434777625415,579.671056589212,-39.2297700580612)) ;
#70204=CARTESIAN_POINT('Origin',(201.434777625415,579.671056589212,-39.4182700580612)) ;
#70205=CARTESIAN_POINT('',(201.434777625415,580.847556589211,-39.2297700580612)) ;
#70206=CARTESIAN_POINT('',(201.434777625415,576.988181589211,-39.2297700580612)) ;
#70207=CARTESIAN_POINT('',(201.434777625407,580.847556589211,-35.2721601717607)) ;
#70208=CARTESIAN_POINT('',(201.434777625415,580.847556589211,-38.5610190928544)) ;
#70209=CARTESIAN_POINT('',(201.434777625407,577.097556589211,-35.2721601717609)) ;
#70210=CARTESIAN_POINT('',(201.434777625415,595.670681589221,-35.2721601717607)) ;
#70211=CARTESIAN_POINT('',(201.434777625415,577.097556589211,-39.2297700580612)) ;
#70212=CARTESIAN_POINT('',(201.434777625415,577.097556589211,-40.5297040214914)) ;
#70213=CARTESIAN_POINT('',(201.434777625415,578.274056589212,-39.2297700580612)) ;
#70214=CARTESIAN_POINT('',(201.434777625415,576.988181589211,-39.2297700580612)) ;
#70215=CARTESIAN_POINT('Origin',(201.434777625415,578.274056589212,-39.4182700580611)) ;
#70216=CARTESIAN_POINT('Origin',(201.559777625415,579.482556589212,-44.5342150424525)) ;
#70217=CARTESIAN_POINT('',(201.559777625415,579.607556589212,-39.4182700580612)) ;
#70218=CARTESIAN_POINT('',(201.559777625415,579.607556589212,-44.5342150424525)) ;
#70219=CARTESIAN_POINT('Origin',(201.559777625415,579.482556589212,-39.4182700580611)) ;
#70220=CARTESIAN_POINT('Origin',(218.198777625414,579.607556589212,-45.9671609920506)) ;
#70221=CARTESIAN_POINT('',(202.262277625415,579.607556589212,-39.4182700580612)) ;
#70222=CARTESIAN_POINT('',(202.262277625415,579.607556589212,-39.8669650424525)) ;
#70223=CARTESIAN_POINT('',(218.198777625414,579.607556589212,-39.4182700580611)) ;
#70224=CARTESIAN_POINT('Origin',(212.018652625408,570.357556589212,-40.2721601717612)) ;
#70225=CARTESIAN_POINT('',(202.262277625405,570.107556589212,-40.2721601717608)) ;
#70226=CARTESIAN_POINT('Origin',(202.262277625405,570.357556589212,-40.2721601717608)) ;
#70227=CARTESIAN_POINT('',(201.559777625406,570.107556589212,-40.2721601717607)) ;
#70228=CARTESIAN_POINT('',(212.018652625408,570.107556589212,-40.2721601717612)) ;
#70229=CARTESIAN_POINT('Origin',(201.559777625406,570.357556589212,-40.2721601717607)) ;
#70230=CARTESIAN_POINT('Origin',(201.559777625406,569.982556589212,-40.2721601717609)) ;
#70231=CARTESIAN_POINT('',(201.434777625406,569.982556589212,-40.2721601717609)) ;
#70232=CARTESIAN_POINT('Origin',(201.184777625406,569.982556589212,-40.2721601717609)) ;
#70233=CARTESIAN_POINT('Origin',(201.559777625406,569.982556589212,-40.2721601717609)) ;
#70234=CARTESIAN_POINT('Origin',(201.184777625406,586.170681589212,-40.2721601717607)) ;
#70235=CARTESIAN_POINT('',(201.434777625406,568.962556589212,-40.2721601717607)) ;
#70236=CARTESIAN_POINT('Origin',(201.184777625406,568.962556589212,-40.2721601717607)) ;
#70237=CARTESIAN_POINT('',(201.434777625414,586.170681589212,-40.2721601717607)) ;
#70238=CARTESIAN_POINT('Origin',(201.559777625406,568.962556589212,-40.2721601717609)) ;
#70239=CARTESIAN_POINT('',(201.559777625406,568.837556589212,-40.2721601717609)) ;
#70240=CARTESIAN_POINT('Origin',(201.559777625406,568.587556589212,-40.2721601717609)) ;
#70241=CARTESIAN_POINT('Origin',(201.559777625406,568.962556589212,-40.2721601717609)) ;
#70242=CARTESIAN_POINT('Origin',(212.844152625408,568.587556589212,-40.2721601717612)) ;
#70243=CARTESIAN_POINT('',(202.262277625405,568.837556589212,-40.2721601717608)) ;
#70244=CARTESIAN_POINT('Origin',(202.262277625405,568.587556589212,-40.2721601717608)) ;
#70245=CARTESIAN_POINT('',(212.844152625408,568.837556589212,-40.2721601717612)) ;
#70246=CARTESIAN_POINT('Origin',(202.262277625405,568.962556589212,-40.2721601717609)) ;
#70247=CARTESIAN_POINT('',(202.387277625405,568.962556589212,-40.2721601717609)) ;
#70248=CARTESIAN_POINT('Origin',(202.637277625405,568.962556589212,-40.2721601717609)) ;
#70249=CARTESIAN_POINT('Origin',(202.262277625405,568.962556589212,-40.2721601717609)) ;
#70250=CARTESIAN_POINT('Origin',(202.637277625405,586.170681589213,-40.2721601717608)) ;
#70251=CARTESIAN_POINT('',(202.387277625405,569.982556589212,-40.2721601717608)) ;
#70252=CARTESIAN_POINT('Origin',(202.637277625405,569.982556589212,-40.2721601717608)) ;
#70253=CARTESIAN_POINT('',(202.387277625413,586.170681589213,-40.2721601717608)) ;
#70254=CARTESIAN_POINT('Origin',(202.262277625405,569.982556589212,-40.2721601717609)) ;
#70255=CARTESIAN_POINT('Origin',(202.262277625405,569.982556589212,-40.2721601717609)) ;
#70256=CARTESIAN_POINT('Origin',(201.559777625414,568.962556589212,-42.3117150424525)) ;
#70257=CARTESIAN_POINT('',(201.434777625414,568.962556589212,-39.4182700580611)) ;
#70258=CARTESIAN_POINT('',(201.434777625414,568.962556589212,-42.3117150424525)) ;
#70259=CARTESIAN_POINT('',(201.559777625414,568.837556589212,-39.4182700580611)) ;
#70260=CARTESIAN_POINT('Origin',(201.559777625414,568.962556589212,-39.4182700580611)) ;
#70261=CARTESIAN_POINT('',(201.559777625414,568.837556589212,-42.3117150424525)) ;
#70262=CARTESIAN_POINT('Origin',(201.434777625414,564.868806589211,-43.1012690928543)) ;
#70263=CARTESIAN_POINT('',(201.434777625414,569.982556589212,-39.4182700580611)) ;
#70264=CARTESIAN_POINT('',(201.434777625414,569.982556589212,-44.5342150424525)) ;
#70265=CARTESIAN_POINT('',(201.434777625414,570.171056589212,-39.2297700580612)) ;
#70266=CARTESIAN_POINT('Origin',(201.434777625414,570.171056589212,-39.4182700580612)) ;
#70267=CARTESIAN_POINT('',(201.434777625414,571.347556589211,-39.2297700580612)) ;
#70268=CARTESIAN_POINT('',(201.434777625414,567.488181589211,-39.2297700580612)) ;
#70269=CARTESIAN_POINT('',(201.434777625407,571.347556589211,-35.2721601717607)) ;
#70270=CARTESIAN_POINT('',(201.434777625414,571.347556589211,-38.5610190928544)) ;
#70271=CARTESIAN_POINT('',(201.434777625407,567.597556589211,-35.2721601717609)) ;
#70272=CARTESIAN_POINT('',(201.434777625414,586.170681589221,-35.2721601717607)) ;
#70273=CARTESIAN_POINT('',(201.434777625414,567.59755658921,-39.2297700580612)) ;
#70274=CARTESIAN_POINT('',(201.434777625414,567.59755658921,-40.5297040214914)) ;
#70275=CARTESIAN_POINT('',(201.434777625414,568.774056589212,-39.2297700580612)) ;
#70276=CARTESIAN_POINT('',(201.434777625414,567.488181589211,-39.2297700580612)) ;
#70277=CARTESIAN_POINT('Origin',(201.434777625414,568.774056589212,-39.4182700580611)) ;
#70278=CARTESIAN_POINT('Origin',(201.559777625414,569.982556589212,-44.5342150424525)) ;
#70279=CARTESIAN_POINT('',(201.559777625414,570.107556589212,-39.4182700580612)) ;
#70280=CARTESIAN_POINT('',(201.559777625414,570.107556589212,-44.5342150424525)) ;
#70281=CARTESIAN_POINT('Origin',(201.559777625414,569.982556589212,-39.4182700580611)) ;
#70282=CARTESIAN_POINT('Origin',(218.198777625412,570.107556589212,-45.9671609920506)) ;
#70283=CARTESIAN_POINT('',(202.262277625413,570.107556589212,-39.4182700580612)) ;
#70284=CARTESIAN_POINT('',(202.262277625413,570.107556589212,-39.8669650424525)) ;
#70285=CARTESIAN_POINT('',(218.198777625413,570.107556589212,-39.4182700580611)) ;
#70286=CARTESIAN_POINT('Origin',(212.018652625409,560.857556589212,-40.2721601717612)) ;
#70287=CARTESIAN_POINT('',(202.262277625406,560.607556589212,-40.2721601717608)) ;
#70288=CARTESIAN_POINT('Origin',(202.262277625406,560.857556589212,-40.2721601717608)) ;
#70289=CARTESIAN_POINT('',(201.559777625406,560.607556589212,-40.2721601717607)) ;
#70290=CARTESIAN_POINT('',(212.018652625409,560.607556589212,-40.2721601717612)) ;
#70291=CARTESIAN_POINT('Origin',(201.559777625406,560.857556589212,-40.2721601717607)) ;
#70292=CARTESIAN_POINT('Origin',(201.559777625406,560.482556589212,-40.2721601717609)) ;
#70293=CARTESIAN_POINT('',(201.434777625406,560.482556589212,-40.2721601717609)) ;
#70294=CARTESIAN_POINT('Origin',(201.184777625406,560.482556589212,-40.2721601717609)) ;
#70295=CARTESIAN_POINT('Origin',(201.559777625406,560.482556589212,-40.2721601717609)) ;
#70296=CARTESIAN_POINT('Origin',(201.184777625406,576.670681589212,-40.2721601717607)) ;
#70297=CARTESIAN_POINT('',(201.434777625406,559.462556589212,-40.2721601717607)) ;
#70298=CARTESIAN_POINT('Origin',(201.184777625406,559.462556589212,-40.2721601717607)) ;
#70299=CARTESIAN_POINT('',(201.434777625412,576.670681589212,-40.2721601717607)) ;
#70300=CARTESIAN_POINT('Origin',(201.559777625406,559.462556589212,-40.2721601717609)) ;
#70301=CARTESIAN_POINT('',(201.559777625406,559.337556589212,-40.2721601717609)) ;
#70302=CARTESIAN_POINT('Origin',(201.559777625406,559.087556589212,-40.2721601717609)) ;
#70303=CARTESIAN_POINT('Origin',(201.559777625406,559.462556589212,-40.2721601717609)) ;
#70304=CARTESIAN_POINT('Origin',(212.844152625408,559.087556589212,-40.2721601717612)) ;
#70305=CARTESIAN_POINT('',(202.262277625406,559.337556589212,-40.2721601717608)) ;
#70306=CARTESIAN_POINT('Origin',(202.262277625406,559.087556589212,-40.2721601717608)) ;
#70307=CARTESIAN_POINT('',(212.844152625408,559.337556589212,-40.2721601717612)) ;
#70308=CARTESIAN_POINT('Origin',(202.262277625406,559.462556589212,-40.2721601717609)) ;
#70309=CARTESIAN_POINT('',(202.387277625406,559.462556589212,-40.2721601717609)) ;
#70310=CARTESIAN_POINT('Origin',(202.637277625406,559.462556589212,-40.2721601717609)) ;
#70311=CARTESIAN_POINT('Origin',(202.262277625406,559.462556589212,-40.2721601717609)) ;
#70312=CARTESIAN_POINT('Origin',(202.637277625406,576.670681589213,-40.2721601717608)) ;
#70313=CARTESIAN_POINT('',(202.387277625406,560.482556589212,-40.2721601717608)) ;
#70314=CARTESIAN_POINT('Origin',(202.637277625406,560.482556589212,-40.2721601717608)) ;
#70315=CARTESIAN_POINT('',(202.387277625412,576.670681589213,-40.2721601717608)) ;
#70316=CARTESIAN_POINT('Origin',(202.262277625406,560.482556589212,-40.2721601717609)) ;
#70317=CARTESIAN_POINT('Origin',(202.262277625406,560.482556589212,-40.2721601717609)) ;
#70318=CARTESIAN_POINT('Origin',(201.559777625412,559.462556589212,-42.3117150424525)) ;
#70319=CARTESIAN_POINT('',(201.434777625412,559.462556589212,-39.4182700580611)) ;
#70320=CARTESIAN_POINT('',(201.434777625412,559.462556589212,-42.3117150424525)) ;
#70321=CARTESIAN_POINT('',(201.559777625412,559.337556589212,-39.4182700580611)) ;
#70322=CARTESIAN_POINT('Origin',(201.559777625412,559.462556589212,-39.4182700580611)) ;
#70323=CARTESIAN_POINT('',(201.559777625412,559.337556589212,-42.3117150424525)) ;
#70324=CARTESIAN_POINT('Origin',(201.434777625412,555.368806589211,-43.1012690928543)) ;
#70325=CARTESIAN_POINT('',(201.434777625412,560.482556589212,-39.4182700580611)) ;
#70326=CARTESIAN_POINT('',(201.434777625412,560.482556589212,-44.5342150424525)) ;
#70327=CARTESIAN_POINT('',(201.434777625412,560.671056589212,-39.2297700580612)) ;
#70328=CARTESIAN_POINT('Origin',(201.434777625412,560.671056589212,-39.4182700580612)) ;
#70329=CARTESIAN_POINT('',(201.434777625412,561.847556589211,-39.2297700580612)) ;
#70330=CARTESIAN_POINT('',(201.434777625412,557.988181589211,-39.2297700580612)) ;
#70331=CARTESIAN_POINT('',(201.434777625407,561.847556589211,-35.2721601717607)) ;
#70332=CARTESIAN_POINT('',(201.434777625412,561.847556589211,-38.5610190928544)) ;
#70333=CARTESIAN_POINT('',(201.434777625407,558.097556589211,-35.2721601717609)) ;
#70334=CARTESIAN_POINT('',(201.434777625412,576.670681589221,-35.2721601717607)) ;
#70335=CARTESIAN_POINT('',(201.434777625412,558.097556589211,-39.2297700580612)) ;
#70336=CARTESIAN_POINT('',(201.434777625412,558.097556589211,-40.5297040214914)) ;
#70337=CARTESIAN_POINT('',(201.434777625412,559.274056589212,-39.2297700580612)) ;
#70338=CARTESIAN_POINT('',(201.434777625412,557.988181589211,-39.2297700580612)) ;
#70339=CARTESIAN_POINT('Origin',(201.434777625412,559.274056589212,-39.4182700580611)) ;
#70340=CARTESIAN_POINT('Origin',(201.559777625412,560.482556589212,-44.5342150424525)) ;
#70341=CARTESIAN_POINT('',(201.559777625412,560.607556589212,-39.4182700580612)) ;
#70342=CARTESIAN_POINT('',(201.559777625412,560.607556589212,-44.5342150424525)) ;
#70343=CARTESIAN_POINT('Origin',(201.559777625412,560.482556589212,-39.4182700580611)) ;
#70344=CARTESIAN_POINT('Origin',(218.198777625411,560.607556589212,-45.9671609920506)) ;
#70345=CARTESIAN_POINT('',(202.262277625412,560.607556589212,-39.4182700580612)) ;
#70346=CARTESIAN_POINT('',(202.262277625412,560.607556589212,-39.8669650424525)) ;
#70347=CARTESIAN_POINT('',(218.198777625411,560.607556589212,-39.4182700580611)) ;
#70348=CARTESIAN_POINT('Origin',(212.018652625409,551.357556589212,-40.2721601717612)) ;
#70349=CARTESIAN_POINT('',(202.262277625406,551.107556589212,-40.2721601717608)) ;
#70350=CARTESIAN_POINT('Origin',(202.262277625406,551.357556589212,-40.2721601717608)) ;
#70351=CARTESIAN_POINT('',(201.559777625406,551.107556589212,-40.2721601717607)) ;
#70352=CARTESIAN_POINT('',(212.018652625409,551.107556589212,-40.2721601717612)) ;
#70353=CARTESIAN_POINT('Origin',(201.559777625406,551.357556589212,-40.2721601717607)) ;
#70354=CARTESIAN_POINT('Origin',(201.559777625406,550.982556589212,-40.2721601717609)) ;
#70355=CARTESIAN_POINT('',(201.434777625406,550.982556589212,-40.2721601717609)) ;
#70356=CARTESIAN_POINT('Origin',(201.184777625406,550.982556589212,-40.2721601717609)) ;
#70357=CARTESIAN_POINT('Origin',(201.559777625406,550.982556589212,-40.2721601717609)) ;
#70358=CARTESIAN_POINT('Origin',(201.184777625406,567.170681589212,-40.2721601717607)) ;
#70359=CARTESIAN_POINT('',(201.434777625406,549.962556589212,-40.2721601717607)) ;
#70360=CARTESIAN_POINT('Origin',(201.184777625406,549.962556589212,-40.2721601717607)) ;
#70361=CARTESIAN_POINT('',(201.43477762541,567.170681589212,-40.2721601717607)) ;
#70362=CARTESIAN_POINT('Origin',(201.559777625406,549.962556589212,-40.2721601717609)) ;
#70363=CARTESIAN_POINT('',(201.559777625407,549.837556589212,-40.2721601717609)) ;
#70364=CARTESIAN_POINT('Origin',(201.559777625407,549.587556589212,-40.2721601717609)) ;
#70365=CARTESIAN_POINT('Origin',(201.559777625406,549.962556589212,-40.2721601717609)) ;
#70366=CARTESIAN_POINT('Origin',(212.844152625409,549.587556589212,-40.2721601717612)) ;
#70367=CARTESIAN_POINT('',(202.262277625406,549.837556589212,-40.2721601717608)) ;
#70368=CARTESIAN_POINT('Origin',(202.262277625406,549.587556589212,-40.2721601717608)) ;
#70369=CARTESIAN_POINT('',(212.844152625409,549.837556589212,-40.2721601717612)) ;
#70370=CARTESIAN_POINT('Origin',(202.262277625406,549.962556589212,-40.2721601717609)) ;
#70371=CARTESIAN_POINT('',(202.387277625406,549.962556589212,-40.2721601717609)) ;
#70372=CARTESIAN_POINT('Origin',(202.637277625406,549.962556589212,-40.2721601717609)) ;
#70373=CARTESIAN_POINT('Origin',(202.262277625406,549.962556589212,-40.2721601717609)) ;
#70374=CARTESIAN_POINT('Origin',(202.637277625406,567.170681589213,-40.2721601717608)) ;
#70375=CARTESIAN_POINT('',(202.387277625406,550.982556589212,-40.2721601717608)) ;
#70376=CARTESIAN_POINT('Origin',(202.637277625406,550.982556589212,-40.2721601717608)) ;
#70377=CARTESIAN_POINT('',(202.38727762541,567.170681589213,-40.2721601717608)) ;
#70378=CARTESIAN_POINT('Origin',(202.262277625406,550.982556589212,-40.2721601717609)) ;
#70379=CARTESIAN_POINT('Origin',(202.262277625406,550.982556589212,-40.2721601717609)) ;
#70380=CARTESIAN_POINT('Origin',(201.55977762541,549.962556589212,-42.3117150424525)) ;
#70381=CARTESIAN_POINT('',(201.43477762541,549.962556589212,-39.4182700580611)) ;
#70382=CARTESIAN_POINT('',(201.43477762541,549.962556589212,-42.3117150424525)) ;
#70383=CARTESIAN_POINT('',(201.55977762541,549.837556589212,-39.4182700580611)) ;
#70384=CARTESIAN_POINT('Origin',(201.55977762541,549.962556589212,-39.4182700580611)) ;
#70385=CARTESIAN_POINT('',(201.55977762541,549.837556589212,-42.3117150424525)) ;
#70386=CARTESIAN_POINT('Origin',(201.43477762541,545.868806589211,-43.1012690928543)) ;
#70387=CARTESIAN_POINT('',(201.43477762541,550.982556589212,-39.4182700580611)) ;
#70388=CARTESIAN_POINT('',(201.43477762541,550.982556589212,-44.5342150424525)) ;
#70389=CARTESIAN_POINT('',(201.43477762541,551.171056589212,-39.2297700580612)) ;
#70390=CARTESIAN_POINT('Origin',(201.43477762541,551.171056589212,-39.4182700580612)) ;
#70391=CARTESIAN_POINT('',(201.43477762541,552.347556589211,-39.2297700580612)) ;
#70392=CARTESIAN_POINT('',(201.43477762541,548.488181589211,-39.2297700580612)) ;
#70393=CARTESIAN_POINT('',(201.434777625407,552.347556589211,-35.2721601717607)) ;
#70394=CARTESIAN_POINT('',(201.43477762541,552.347556589211,-38.5610190928544)) ;
#70395=CARTESIAN_POINT('',(201.434777625407,548.59755658921,-35.2721601717609)) ;
#70396=CARTESIAN_POINT('',(201.43477762541,567.170681589221,-35.2721601717607)) ;
#70397=CARTESIAN_POINT('',(201.43477762541,548.59755658921,-39.2297700580612)) ;
#70398=CARTESIAN_POINT('',(201.43477762541,548.59755658921,-40.5297040214914)) ;
#70399=CARTESIAN_POINT('',(201.43477762541,549.774056589212,-39.2297700580612)) ;
#70400=CARTESIAN_POINT('',(201.43477762541,548.488181589211,-39.2297700580612)) ;
#70401=CARTESIAN_POINT('Origin',(201.43477762541,549.774056589212,-39.4182700580611)) ;
#70402=CARTESIAN_POINT('Origin',(201.55977762541,550.982556589212,-44.5342150424525)) ;
#70403=CARTESIAN_POINT('',(201.55977762541,551.107556589212,-39.4182700580612)) ;
#70404=CARTESIAN_POINT('',(201.55977762541,551.107556589212,-44.5342150424525)) ;
#70405=CARTESIAN_POINT('Origin',(201.55977762541,550.982556589212,-39.4182700580611)) ;
#70406=CARTESIAN_POINT('Origin',(218.198777625409,551.107556589212,-45.9671609920506)) ;
#70407=CARTESIAN_POINT('',(202.26227762541,551.107556589212,-39.4182700580612)) ;
#70408=CARTESIAN_POINT('',(202.26227762541,551.107556589212,-39.8669650424525)) ;
#70409=CARTESIAN_POINT('',(218.198777625409,551.107556589212,-39.4182700580611)) ;
#70410=CARTESIAN_POINT('Origin',(212.018652625409,541.857556589212,-40.2721601717612)) ;
#70411=CARTESIAN_POINT('',(202.262277625406,541.607556589212,-40.2721601717608)) ;
#70412=CARTESIAN_POINT('Origin',(202.262277625406,541.857556589212,-40.2721601717608)) ;
#70413=CARTESIAN_POINT('',(201.559777625407,541.607556589212,-40.2721601717607)) ;
#70414=CARTESIAN_POINT('',(212.018652625409,541.607556589212,-40.2721601717612)) ;
#70415=CARTESIAN_POINT('Origin',(201.559777625407,541.857556589212,-40.2721601717607)) ;
#70416=CARTESIAN_POINT('Origin',(201.559777625407,541.482556589212,-40.2721601717609)) ;
#70417=CARTESIAN_POINT('',(201.434777625407,541.482556589212,-40.2721601717609)) ;
#70418=CARTESIAN_POINT('Origin',(201.184777625407,541.482556589212,-40.2721601717609)) ;
#70419=CARTESIAN_POINT('Origin',(201.559777625407,541.482556589212,-40.2721601717609)) ;
#70420=CARTESIAN_POINT('Origin',(201.184777625407,557.670681589212,-40.2721601717607)) ;
#70421=CARTESIAN_POINT('',(201.434777625407,540.462556589212,-40.2721601717607)) ;
#70422=CARTESIAN_POINT('Origin',(201.184777625407,540.462556589212,-40.2721601717607)) ;
#70423=CARTESIAN_POINT('',(201.434777625409,557.670681589212,-40.2721601717607)) ;
#70424=CARTESIAN_POINT('Origin',(201.559777625407,540.462556589212,-40.2721601717609)) ;
#70425=CARTESIAN_POINT('',(201.559777625407,540.337556589212,-40.2721601717609)) ;
#70426=CARTESIAN_POINT('Origin',(201.559777625407,540.087556589212,-40.2721601717609)) ;
#70427=CARTESIAN_POINT('Origin',(201.559777625407,540.462556589212,-40.2721601717609)) ;
#70428=CARTESIAN_POINT('Origin',(212.844152625409,540.087556589212,-40.2721601717612)) ;
#70429=CARTESIAN_POINT('',(202.262277625406,540.337556589212,-40.2721601717608)) ;
#70430=CARTESIAN_POINT('Origin',(202.262277625406,540.087556589212,-40.2721601717608)) ;
#70431=CARTESIAN_POINT('',(212.844152625409,540.337556589212,-40.2721601717612)) ;
#70432=CARTESIAN_POINT('Origin',(202.262277625406,540.462556589212,-40.2721601717609)) ;
#70433=CARTESIAN_POINT('',(202.387277625406,540.462556589212,-40.2721601717609)) ;
#70434=CARTESIAN_POINT('Origin',(202.637277625406,540.462556589212,-40.2721601717609)) ;
#70435=CARTESIAN_POINT('Origin',(202.262277625406,540.462556589212,-40.2721601717609)) ;
#70436=CARTESIAN_POINT('Origin',(202.637277625406,557.670681589212,-40.2721601717608)) ;
#70437=CARTESIAN_POINT('',(202.387277625406,541.482556589212,-40.2721601717608)) ;
#70438=CARTESIAN_POINT('Origin',(202.637277625406,541.482556589212,-40.2721601717608)) ;
#70439=CARTESIAN_POINT('',(202.387277625408,557.670681589212,-40.2721601717608)) ;
#70440=CARTESIAN_POINT('Origin',(202.262277625406,541.482556589212,-40.2721601717609)) ;
#70441=CARTESIAN_POINT('Origin',(202.262277625406,541.482556589212,-40.2721601717609)) ;
#70442=CARTESIAN_POINT('Origin',(201.559777625409,540.462556589212,-42.3117150424525)) ;
#70443=CARTESIAN_POINT('',(201.434777625409,540.462556589212,-39.4182700580611)) ;
#70444=CARTESIAN_POINT('',(201.434777625409,540.462556589212,-42.3117150424525)) ;
#70445=CARTESIAN_POINT('',(201.559777625409,540.337556589212,-39.4182700580611)) ;
#70446=CARTESIAN_POINT('Origin',(201.559777625409,540.462556589212,-39.4182700580611)) ;
#70447=CARTESIAN_POINT('',(201.559777625409,540.337556589212,-42.3117150424525)) ;
#70448=CARTESIAN_POINT('Origin',(201.434777625409,536.368806589211,-43.1012690928543)) ;
#70449=CARTESIAN_POINT('',(201.434777625409,541.482556589212,-39.4182700580611)) ;
#70450=CARTESIAN_POINT('',(201.434777625409,541.482556589212,-44.5342150424525)) ;
#70451=CARTESIAN_POINT('',(201.434777625409,541.671056589212,-39.2297700580612)) ;
#70452=CARTESIAN_POINT('Origin',(201.434777625409,541.671056589212,-39.4182700580612)) ;
#70453=CARTESIAN_POINT('',(201.434777625409,542.847556589211,-39.2297700580612)) ;
#70454=CARTESIAN_POINT('',(201.434777625409,538.988181589211,-39.2297700580612)) ;
#70455=CARTESIAN_POINT('',(201.434777625407,542.847556589211,-35.2721601717607)) ;
#70456=CARTESIAN_POINT('',(201.434777625409,542.847556589211,-38.5610190928544)) ;
#70457=CARTESIAN_POINT('',(201.434777625407,539.09755658921,-35.2721601717609)) ;
#70458=CARTESIAN_POINT('',(201.434777625409,557.670681589221,-35.2721601717607)) ;
#70459=CARTESIAN_POINT('',(201.434777625409,539.09755658921,-39.2297700580612)) ;
#70460=CARTESIAN_POINT('',(201.434777625409,539.09755658921,-40.5297040214914)) ;
#70461=CARTESIAN_POINT('',(201.434777625409,540.274056589212,-39.2297700580612)) ;
#70462=CARTESIAN_POINT('',(201.434777625409,538.988181589211,-39.2297700580612)) ;
#70463=CARTESIAN_POINT('Origin',(201.434777625409,540.274056589212,-39.4182700580611)) ;
#70464=CARTESIAN_POINT('Origin',(201.559777625409,541.482556589212,-44.5342150424525)) ;
#70465=CARTESIAN_POINT('',(201.559777625409,541.607556589212,-39.4182700580612)) ;
#70466=CARTESIAN_POINT('',(201.559777625409,541.607556589212,-44.5342150424525)) ;
#70467=CARTESIAN_POINT('Origin',(201.559777625409,541.482556589212,-39.4182700580611)) ;
#70468=CARTESIAN_POINT('Origin',(218.198777625407,541.607556589212,-45.9671609920506)) ;
#70469=CARTESIAN_POINT('',(202.262277625408,541.607556589212,-39.4182700580612)) ;
#70470=CARTESIAN_POINT('',(202.262277625408,541.607556589212,-39.8669650424525)) ;
#70471=CARTESIAN_POINT('',(218.198777625408,541.607556589212,-39.4182700580611)) ;
#70472=CARTESIAN_POINT('Origin',(212.01865262541,532.357556589212,-40.2721601717612)) ;
#70473=CARTESIAN_POINT('',(202.262277625407,532.107556589212,-40.2721601717608)) ;
#70474=CARTESIAN_POINT('Origin',(202.262277625407,532.357556589212,-40.2721601717608)) ;
#70475=CARTESIAN_POINT('',(201.559777625407,532.107556589212,-40.2721601717607)) ;
#70476=CARTESIAN_POINT('',(212.01865262541,532.107556589212,-40.2721601717612)) ;
#70477=CARTESIAN_POINT('Origin',(201.559777625407,532.357556589212,-40.2721601717607)) ;
#70478=CARTESIAN_POINT('Origin',(201.559777625407,531.982556589212,-40.2721601717609)) ;
#70479=CARTESIAN_POINT('',(201.434777625407,531.982556589212,-40.2721601717609)) ;
#70480=CARTESIAN_POINT('Origin',(201.184777625407,531.982556589212,-40.2721601717609)) ;
#70481=CARTESIAN_POINT('Origin',(201.559777625407,531.982556589212,-40.2721601717609)) ;
#70482=CARTESIAN_POINT('Origin',(201.184777625407,548.170681589212,-40.2721601717607)) ;
#70483=CARTESIAN_POINT('',(201.434777625407,530.962556589212,-40.2721601717607)) ;
#70484=CARTESIAN_POINT('Origin',(201.184777625407,530.962556589212,-40.2721601717607)) ;
#70485=CARTESIAN_POINT('',(201.434777625407,548.170681589212,-40.2721601717607)) ;
#70486=CARTESIAN_POINT('Origin',(201.559777625407,530.962556589212,-40.2721601717609)) ;
#70487=CARTESIAN_POINT('',(201.559777625407,530.837556589212,-40.2721601717609)) ;
#70488=CARTESIAN_POINT('Origin',(201.559777625407,530.587556589212,-40.2721601717609)) ;
#70489=CARTESIAN_POINT('Origin',(201.559777625407,530.962556589212,-40.2721601717609)) ;
#70490=CARTESIAN_POINT('Origin',(212.844152625409,530.587556589212,-40.2721601717612)) ;
#70491=CARTESIAN_POINT('',(202.262277625407,530.837556589212,-40.2721601717608)) ;
#70492=CARTESIAN_POINT('Origin',(202.262277625407,530.587556589212,-40.2721601717608)) ;
#70493=CARTESIAN_POINT('',(212.844152625409,530.837556589212,-40.2721601717612)) ;
#70494=CARTESIAN_POINT('Origin',(202.262277625407,530.962556589212,-40.2721601717609)) ;
#70495=CARTESIAN_POINT('',(202.387277625407,530.962556589212,-40.2721601717609)) ;
#70496=CARTESIAN_POINT('Origin',(202.637277625407,530.962556589212,-40.2721601717609)) ;
#70497=CARTESIAN_POINT('Origin',(202.262277625407,530.962556589212,-40.2721601717609)) ;
#70498=CARTESIAN_POINT('Origin',(202.637277625407,548.170681589212,-40.2721601717608)) ;
#70499=CARTESIAN_POINT('',(202.387277625407,531.982556589212,-40.2721601717608)) ;
#70500=CARTESIAN_POINT('Origin',(202.637277625407,531.982556589212,-40.2721601717608)) ;
#70501=CARTESIAN_POINT('',(202.387277625407,548.170681589212,-40.2721601717608)) ;
#70502=CARTESIAN_POINT('Origin',(202.262277625407,531.982556589212,-40.2721601717609)) ;
#70503=CARTESIAN_POINT('Origin',(202.262277625407,531.982556589212,-40.2721601717609)) ;
#70504=CARTESIAN_POINT('Origin',(201.559777625407,530.962556589212,-42.3117150424525)) ;
#70505=CARTESIAN_POINT('',(201.434777625407,530.962556589212,-39.4182700580611)) ;
#70506=CARTESIAN_POINT('',(201.434777625407,530.962556589212,-42.3117150424525)) ;
#70507=CARTESIAN_POINT('',(201.559777625407,530.837556589212,-39.4182700580611)) ;
#70508=CARTESIAN_POINT('Origin',(201.559777625407,530.962556589212,-39.4182700580611)) ;
#70509=CARTESIAN_POINT('',(201.559777625407,530.837556589212,-42.3117150424525)) ;
#70510=CARTESIAN_POINT('Origin',(201.434777625407,526.868806589211,-43.1012690928543)) ;
#70511=CARTESIAN_POINT('',(201.434777625407,529.59755658921,-35.2721601717609)) ;
#70512=CARTESIAN_POINT('',(201.434777625407,533.347556589211,-35.2721601717607)) ;
#70513=CARTESIAN_POINT('',(201.434777625407,548.170681589221,-35.2721601717607)) ;
#70514=CARTESIAN_POINT('',(201.434777625407,529.59755658921,-39.2297700580612)) ;
#70515=CARTESIAN_POINT('',(201.434777625407,529.59755658921,-40.5297040214914)) ;
#70516=CARTESIAN_POINT('',(201.434777625407,530.774056589212,-39.2297700580612)) ;
#70517=CARTESIAN_POINT('',(201.434777625407,529.488181589211,-39.2297700580612)) ;
#70518=CARTESIAN_POINT('Origin',(201.434777625407,530.774056589212,-39.4182700580611)) ;
#70519=CARTESIAN_POINT('',(201.434777625407,531.982556589212,-39.4182700580611)) ;
#70520=CARTESIAN_POINT('',(201.434777625407,531.982556589212,-44.5342150424525)) ;
#70521=CARTESIAN_POINT('',(201.434777625407,532.171056589212,-39.2297700580612)) ;
#70522=CARTESIAN_POINT('Origin',(201.434777625407,532.171056589212,-39.4182700580612)) ;
#70523=CARTESIAN_POINT('',(201.434777625407,533.347556589211,-39.2297700580612)) ;
#70524=CARTESIAN_POINT('',(201.434777625407,529.488181589211,-39.2297700580612)) ;
#70525=CARTESIAN_POINT('',(201.434777625407,533.347556589211,-38.5610190928544)) ;
#70526=CARTESIAN_POINT('Origin',(201.559777625407,531.982556589212,-44.5342150424525)) ;
#70527=CARTESIAN_POINT('',(201.559777625407,532.107556589212,-39.4182700580612)) ;
#70528=CARTESIAN_POINT('',(201.559777625407,532.107556589212,-44.5342150424525)) ;
#70529=CARTESIAN_POINT('Origin',(201.559777625407,531.982556589212,-39.4182700580611)) ;
#70530=CARTESIAN_POINT('Origin',(218.198777625406,532.107556589212,-45.9671609920506)) ;
#70531=CARTESIAN_POINT('',(202.262277625407,532.107556589212,-39.4182700580612)) ;
#70532=CARTESIAN_POINT('',(202.262277625407,532.107556589212,-39.8669650424525)) ;
#70533=CARTESIAN_POINT('',(218.198777625406,532.107556589212,-39.4182700580611)) ;
#70534=CARTESIAN_POINT('Origin',(201.57290262541,609.722556589211,-35.2721601717607)) ;
#70535=CARTESIAN_POINT('',(209.814777625407,609.722556589211,-35.0221601717611)) ;
#70536=CARTESIAN_POINT('',(209.814777625407,609.472556589211,-35.2721601717611)) ;
#70537=CARTESIAN_POINT('Origin',(209.814777625407,609.722556589211,-35.2721601717611)) ;
#70538=CARTESIAN_POINT('',(210.517277625407,609.472556589211,-35.2721601717611)) ;
#70539=CARTESIAN_POINT('',(201.57290262541,609.472556589211,-35.2721601717607)) ;
#70540=CARTESIAN_POINT('',(210.517277625407,609.722556589211,-35.0221601717611)) ;
#70541=CARTESIAN_POINT('Origin',(210.517277625407,609.722556589211,-35.2721601717611)) ;
#70542=CARTESIAN_POINT('',(201.57290262541,609.722556589211,-35.0221601717607)) ;
#70543=CARTESIAN_POINT('Origin',(210.517277625407,609.347556589211,-35.2721601717609)) ;
#70544=CARTESIAN_POINT('',(210.642277625407,609.347556589211,-35.2721601717609)) ;
#70545=CARTESIAN_POINT('',(210.892277625407,609.347556589211,-35.0221601717612)) ;
#70546=CARTESIAN_POINT('Origin',(210.892277625407,609.347556589211,-35.2721601717609)) ;
#70547=CARTESIAN_POINT('Origin',(210.517277625407,609.347556589211,-35.0221601717611)) ;
#70548=CARTESIAN_POINT('Origin',(210.517277625407,609.347556589211,-35.2721601717609)) ;
#70549=CARTESIAN_POINT('Origin',(210.892277625407,624.170681589221,-35.2721601717611)) ;
#70550=CARTESIAN_POINT('',(210.642277625407,605.597556589211,-35.2721601717612)) ;
#70551=CARTESIAN_POINT('',(210.892277625407,605.597556589211,-35.0221601717612)) ;
#70552=CARTESIAN_POINT('Origin',(210.892277625407,605.597556589211,-35.2721601717612)) ;
#70553=CARTESIAN_POINT('',(210.892277625407,624.170681589221,-35.0221601717611)) ;
#70554=CARTESIAN_POINT('',(210.64227762542,624.170681589221,-35.2721601717611)) ;
#70555=CARTESIAN_POINT('Origin',(210.517277625407,605.597556589211,-35.2721601717609)) ;
#70556=CARTESIAN_POINT('',(210.517277625407,605.472556589211,-35.2721601717609)) ;
#70557=CARTESIAN_POINT('',(210.517277625407,605.222556589211,-35.0221601717611)) ;
#70558=CARTESIAN_POINT('Origin',(210.517277625407,605.222556589211,-35.2721601717609)) ;
#70559=CARTESIAN_POINT('Origin',(210.517277625407,605.597556589211,-35.0221601717611)) ;
#70560=CARTESIAN_POINT('Origin',(210.517277625407,605.597556589211,-35.2721601717609)) ;
#70561=CARTESIAN_POINT('Origin',(205.938476772278,605.222556589211,-35.2721601717609)) ;
#70562=CARTESIAN_POINT('',(209.814777625407,605.472556589211,-35.2721601717611)) ;
#70563=CARTESIAN_POINT('',(209.814777625407,605.222556589211,-35.0221601717611)) ;
#70564=CARTESIAN_POINT('Origin',(209.814777625407,605.222556589211,-35.2721601717611)) ;
#70565=CARTESIAN_POINT('',(205.938476772278,605.222556589211,-35.0221601717609)) ;
#70566=CARTESIAN_POINT('',(205.938476772278,605.472556589211,-35.2721601717609)) ;
#70567=CARTESIAN_POINT('Origin',(209.814777625407,605.597556589211,-35.2721601717609)) ;
#70568=CARTESIAN_POINT('',(209.689777625407,605.597556589211,-35.2721601717609)) ;
#70569=CARTESIAN_POINT('',(209.439777625407,605.597556589211,-35.0221601717611)) ;
#70570=CARTESIAN_POINT('Origin',(209.439777625407,605.597556589211,-35.2721601717609)) ;
#70571=CARTESIAN_POINT('Origin',(209.814777625407,605.597556589211,-35.0221601717611)) ;
#70572=CARTESIAN_POINT('Origin',(209.814777625407,605.597556589211,-35.2721601717609)) ;
#70573=CARTESIAN_POINT('Origin',(209.439777625407,624.170681589221,-35.2721601717611)) ;
#70574=CARTESIAN_POINT('',(209.689777625407,609.347556589211,-35.2721601717611)) ;
#70575=CARTESIAN_POINT('',(209.439777625407,609.347556589211,-35.0221601717611)) ;
#70576=CARTESIAN_POINT('Origin',(209.439777625407,609.347556589211,-35.2721601717611)) ;
#70577=CARTESIAN_POINT('',(209.439777625407,624.170681589221,-35.0221601717611)) ;
#70578=CARTESIAN_POINT('',(209.68977762542,624.170681589221,-35.2721601717611)) ;
#70579=CARTESIAN_POINT('Origin',(209.814777625407,609.347556589211,-35.2721601717609)) ;
#70580=CARTESIAN_POINT('Origin',(209.814777625407,609.347556589211,-35.0221601717611)) ;
#70581=CARTESIAN_POINT('Origin',(209.814777625407,609.347556589211,-35.2721601717609)) ;
#70582=CARTESIAN_POINT('Origin',(210.51727762542,605.597556589211,-35.7037040214914)) ;
#70583=CARTESIAN_POINT('',(210.64227762542,605.597556589211,-39.2297690928544)) ;
#70584=CARTESIAN_POINT('',(210.64227762542,605.597556589211,-35.7037040214914)) ;
#70585=CARTESIAN_POINT('',(210.51727762542,605.472556589211,-39.2297690928544)) ;
#70586=CARTESIAN_POINT('Origin',(210.51727762542,605.597556589211,-39.2297690928544)) ;
#70587=CARTESIAN_POINT('',(210.51727762542,605.472556589211,-35.7037040214914)) ;
#70588=CARTESIAN_POINT('Origin',(210.64227762542,602.868806589211,-33.4492690928543)) ;
#70589=CARTESIAN_POINT('',(210.64227762542,609.347556589211,-39.2297690928544)) ;
#70590=CARTESIAN_POINT('',(210.64227762542,609.347556589211,-33.7350190928543)) ;
#70591=CARTESIAN_POINT('',(210.64227762542,605.488181589211,-39.2297690928544)) ;
#70592=CARTESIAN_POINT('Origin',(210.51727762542,609.347556589211,-33.7350190928543)) ;
#70593=CARTESIAN_POINT('',(210.51727762542,609.472556589211,-39.2297690928544)) ;
#70594=CARTESIAN_POINT('',(210.51727762542,609.472556589211,-33.7350190928543)) ;
#70595=CARTESIAN_POINT('Origin',(210.51727762542,609.347556589211,-39.2297690928544)) ;
#70596=CARTESIAN_POINT('Origin',(197.30727762542,609.472556589211,-34.0207690928544)) ;
#70597=CARTESIAN_POINT('',(209.81477762542,609.472556589211,-39.2297690928544)) ;
#70598=CARTESIAN_POINT('',(209.81477762542,609.472556589211,-38.5610190928544)) ;
#70599=CARTESIAN_POINT('',(207.75302762542,609.472556589211,-39.2297690928544)) ;
#70600=CARTESIAN_POINT('Origin',(201.57290262541,600.222556589211,-35.2721601717607)) ;
#70601=CARTESIAN_POINT('',(209.814777625407,600.222556589211,-35.0221601717611)) ;
#70602=CARTESIAN_POINT('',(209.814777625407,599.972556589211,-35.2721601717611)) ;
#70603=CARTESIAN_POINT('Origin',(209.814777625407,600.222556589211,-35.2721601717611)) ;
#70604=CARTESIAN_POINT('',(210.517277625407,599.972556589211,-35.2721601717611)) ;
#70605=CARTESIAN_POINT('',(201.57290262541,599.972556589211,-35.2721601717607)) ;
#70606=CARTESIAN_POINT('',(210.517277625407,600.222556589211,-35.0221601717611)) ;
#70607=CARTESIAN_POINT('Origin',(210.517277625407,600.222556589211,-35.2721601717611)) ;
#70608=CARTESIAN_POINT('',(201.57290262541,600.222556589211,-35.0221601717607)) ;
#70609=CARTESIAN_POINT('Origin',(210.517277625407,599.847556589211,-35.2721601717609)) ;
#70610=CARTESIAN_POINT('',(210.642277625407,599.847556589211,-35.2721601717609)) ;
#70611=CARTESIAN_POINT('',(210.892277625407,599.847556589211,-35.0221601717612)) ;
#70612=CARTESIAN_POINT('Origin',(210.892277625407,599.847556589211,-35.2721601717609)) ;
#70613=CARTESIAN_POINT('Origin',(210.517277625407,599.847556589211,-35.0221601717611)) ;
#70614=CARTESIAN_POINT('Origin',(210.517277625407,599.847556589211,-35.2721601717609)) ;
#70615=CARTESIAN_POINT('Origin',(210.892277625407,614.670681589221,-35.2721601717611)) ;
#70616=CARTESIAN_POINT('',(210.642277625407,596.097556589211,-35.2721601717612)) ;
#70617=CARTESIAN_POINT('',(210.892277625407,596.097556589211,-35.0221601717612)) ;
#70618=CARTESIAN_POINT('Origin',(210.892277625407,596.097556589211,-35.2721601717612)) ;
#70619=CARTESIAN_POINT('',(210.892277625407,614.670681589221,-35.0221601717611)) ;
#70620=CARTESIAN_POINT('',(210.642277625419,614.670681589221,-35.2721601717611)) ;
#70621=CARTESIAN_POINT('Origin',(210.517277625407,596.097556589211,-35.2721601717609)) ;
#70622=CARTESIAN_POINT('',(210.517277625407,595.972556589211,-35.2721601717609)) ;
#70623=CARTESIAN_POINT('',(210.517277625407,595.722556589211,-35.0221601717611)) ;
#70624=CARTESIAN_POINT('Origin',(210.517277625407,595.722556589211,-35.2721601717609)) ;
#70625=CARTESIAN_POINT('Origin',(210.517277625407,596.097556589211,-35.0221601717611)) ;
#70626=CARTESIAN_POINT('Origin',(210.517277625407,596.097556589211,-35.2721601717609)) ;
#70627=CARTESIAN_POINT('Origin',(205.938476772278,595.722556589211,-35.2721601717609)) ;
#70628=CARTESIAN_POINT('',(209.814777625407,595.972556589211,-35.2721601717611)) ;
#70629=CARTESIAN_POINT('',(209.814777625407,595.722556589211,-35.0221601717611)) ;
#70630=CARTESIAN_POINT('Origin',(209.814777625407,595.722556589211,-35.2721601717611)) ;
#70631=CARTESIAN_POINT('',(205.938476772278,595.722556589211,-35.0221601717609)) ;
#70632=CARTESIAN_POINT('',(205.938476772278,595.972556589211,-35.2721601717609)) ;
#70633=CARTESIAN_POINT('Origin',(209.814777625407,596.097556589211,-35.2721601717609)) ;
#70634=CARTESIAN_POINT('',(209.689777625407,596.097556589211,-35.2721601717609)) ;
#70635=CARTESIAN_POINT('',(209.439777625407,596.097556589211,-35.0221601717611)) ;
#70636=CARTESIAN_POINT('Origin',(209.439777625407,596.097556589211,-35.2721601717609)) ;
#70637=CARTESIAN_POINT('Origin',(209.814777625407,596.097556589211,-35.0221601717611)) ;
#70638=CARTESIAN_POINT('Origin',(209.814777625407,596.097556589211,-35.2721601717609)) ;
#70639=CARTESIAN_POINT('Origin',(209.439777625407,614.670681589221,-35.2721601717611)) ;
#70640=CARTESIAN_POINT('',(209.689777625407,599.847556589211,-35.2721601717611)) ;
#70641=CARTESIAN_POINT('',(209.439777625407,599.847556589211,-35.0221601717611)) ;
#70642=CARTESIAN_POINT('Origin',(209.439777625407,599.847556589211,-35.2721601717611)) ;
#70643=CARTESIAN_POINT('',(209.439777625407,614.670681589221,-35.0221601717611)) ;
#70644=CARTESIAN_POINT('',(209.689777625418,614.670681589221,-35.2721601717611)) ;
#70645=CARTESIAN_POINT('Origin',(209.814777625407,599.847556589211,-35.2721601717609)) ;
#70646=CARTESIAN_POINT('Origin',(209.814777625407,599.847556589211,-35.0221601717611)) ;
#70647=CARTESIAN_POINT('Origin',(209.814777625407,599.847556589211,-35.2721601717609)) ;
#70648=CARTESIAN_POINT('Origin',(210.517277625419,596.097556589211,-35.7037040214914)) ;
#70649=CARTESIAN_POINT('',(210.642277625419,596.097556589211,-39.2297690928544)) ;
#70650=CARTESIAN_POINT('',(210.642277625419,596.097556589211,-35.7037040214914)) ;
#70651=CARTESIAN_POINT('',(210.517277625419,595.972556589211,-39.2297690928544)) ;
#70652=CARTESIAN_POINT('Origin',(210.517277625419,596.097556589211,-39.2297690928544)) ;
#70653=CARTESIAN_POINT('',(210.517277625419,595.972556589211,-35.7037040214914)) ;
#70654=CARTESIAN_POINT('Origin',(210.642277625419,593.368806589211,-33.4492690928543)) ;
#70655=CARTESIAN_POINT('',(210.642277625419,599.847556589211,-39.2297690928544)) ;
#70656=CARTESIAN_POINT('',(210.642277625419,599.847556589211,-33.7350190928543)) ;
#70657=CARTESIAN_POINT('',(210.642277625419,595.988181589211,-39.2297690928544)) ;
#70658=CARTESIAN_POINT('Origin',(210.517277625419,599.847556589211,-33.7350190928543)) ;
#70659=CARTESIAN_POINT('',(210.517277625419,599.972556589211,-39.2297690928544)) ;
#70660=CARTESIAN_POINT('',(210.517277625419,599.972556589211,-33.7350190928543)) ;
#70661=CARTESIAN_POINT('Origin',(210.517277625419,599.847556589211,-39.2297690928544)) ;
#70662=CARTESIAN_POINT('Origin',(197.307277625418,599.972556589211,-34.0207690928544)) ;
#70663=CARTESIAN_POINT('',(209.814777625418,599.972556589211,-39.2297690928544)) ;
#70664=CARTESIAN_POINT('',(209.814777625418,599.972556589211,-38.5610190928544)) ;
#70665=CARTESIAN_POINT('',(207.753027625418,599.972556589211,-39.2297690928544)) ;
#70666=CARTESIAN_POINT('Origin',(201.57290262541,590.722556589211,-35.2721601717607)) ;
#70667=CARTESIAN_POINT('',(209.814777625407,590.722556589211,-35.0221601717611)) ;
#70668=CARTESIAN_POINT('',(209.814777625407,590.472556589211,-35.2721601717611)) ;
#70669=CARTESIAN_POINT('Origin',(209.814777625407,590.722556589211,-35.2721601717611)) ;
#70670=CARTESIAN_POINT('',(210.517277625407,590.472556589211,-35.2721601717611)) ;
#70671=CARTESIAN_POINT('',(201.57290262541,590.472556589211,-35.2721601717607)) ;
#70672=CARTESIAN_POINT('',(210.517277625407,590.722556589211,-35.0221601717611)) ;
#70673=CARTESIAN_POINT('Origin',(210.517277625407,590.722556589211,-35.2721601717611)) ;
#70674=CARTESIAN_POINT('',(201.57290262541,590.722556589211,-35.0221601717607)) ;
#70675=CARTESIAN_POINT('Origin',(210.517277625407,590.347556589211,-35.2721601717609)) ;
#70676=CARTESIAN_POINT('',(210.642277625407,590.347556589211,-35.2721601717609)) ;
#70677=CARTESIAN_POINT('',(210.892277625407,590.347556589211,-35.0221601717612)) ;
#70678=CARTESIAN_POINT('Origin',(210.892277625407,590.347556589211,-35.2721601717609)) ;
#70679=CARTESIAN_POINT('Origin',(210.517277625407,590.347556589211,-35.0221601717611)) ;
#70680=CARTESIAN_POINT('Origin',(210.517277625407,590.347556589211,-35.2721601717609)) ;
#70681=CARTESIAN_POINT('Origin',(210.892277625407,605.170681589221,-35.2721601717611)) ;
#70682=CARTESIAN_POINT('',(210.642277625407,586.597556589211,-35.2721601717612)) ;
#70683=CARTESIAN_POINT('',(210.892277625407,586.597556589211,-35.0221601717612)) ;
#70684=CARTESIAN_POINT('Origin',(210.892277625407,586.597556589211,-35.2721601717612)) ;
#70685=CARTESIAN_POINT('',(210.892277625407,605.170681589221,-35.0221601717611)) ;
#70686=CARTESIAN_POINT('',(210.642277625417,605.170681589221,-35.2721601717611)) ;
#70687=CARTESIAN_POINT('Origin',(210.517277625407,586.597556589211,-35.2721601717609)) ;
#70688=CARTESIAN_POINT('',(210.517277625407,586.472556589211,-35.2721601717609)) ;
#70689=CARTESIAN_POINT('',(210.517277625407,586.222556589211,-35.0221601717611)) ;
#70690=CARTESIAN_POINT('Origin',(210.517277625407,586.222556589211,-35.2721601717609)) ;
#70691=CARTESIAN_POINT('Origin',(210.517277625407,586.597556589211,-35.0221601717611)) ;
#70692=CARTESIAN_POINT('Origin',(210.517277625407,586.597556589211,-35.2721601717609)) ;
#70693=CARTESIAN_POINT('Origin',(205.938476772278,586.222556589211,-35.2721601717609)) ;
#70694=CARTESIAN_POINT('',(209.814777625407,586.472556589211,-35.2721601717611)) ;
#70695=CARTESIAN_POINT('',(209.814777625407,586.222556589211,-35.0221601717611)) ;
#70696=CARTESIAN_POINT('Origin',(209.814777625407,586.222556589211,-35.2721601717611)) ;
#70697=CARTESIAN_POINT('',(205.938476772278,586.222556589211,-35.0221601717609)) ;
#70698=CARTESIAN_POINT('',(205.938476772278,586.472556589211,-35.2721601717609)) ;
#70699=CARTESIAN_POINT('Origin',(209.814777625407,586.597556589211,-35.2721601717609)) ;
#70700=CARTESIAN_POINT('',(209.689777625407,586.597556589211,-35.2721601717609)) ;
#70701=CARTESIAN_POINT('',(209.439777625407,586.597556589211,-35.0221601717611)) ;
#70702=CARTESIAN_POINT('Origin',(209.439777625407,586.597556589211,-35.2721601717609)) ;
#70703=CARTESIAN_POINT('Origin',(209.814777625407,586.597556589211,-35.0221601717611)) ;
#70704=CARTESIAN_POINT('Origin',(209.814777625407,586.597556589211,-35.2721601717609)) ;
#70705=CARTESIAN_POINT('Origin',(209.439777625407,605.170681589221,-35.2721601717611)) ;
#70706=CARTESIAN_POINT('',(209.689777625407,590.347556589211,-35.2721601717611)) ;
#70707=CARTESIAN_POINT('',(209.439777625407,590.347556589211,-35.0221601717611)) ;
#70708=CARTESIAN_POINT('Origin',(209.439777625407,590.347556589211,-35.2721601717611)) ;
#70709=CARTESIAN_POINT('',(209.439777625407,605.170681589221,-35.0221601717611)) ;
#70710=CARTESIAN_POINT('',(209.689777625417,605.170681589221,-35.2721601717611)) ;
#70711=CARTESIAN_POINT('Origin',(209.814777625407,590.347556589211,-35.2721601717609)) ;
#70712=CARTESIAN_POINT('Origin',(209.814777625407,590.347556589211,-35.0221601717611)) ;
#70713=CARTESIAN_POINT('Origin',(209.814777625407,590.347556589211,-35.2721601717609)) ;
#70714=CARTESIAN_POINT('Origin',(210.517277625417,586.597556589211,-35.7037040214914)) ;
#70715=CARTESIAN_POINT('',(210.642277625417,586.597556589211,-39.2297690928544)) ;
#70716=CARTESIAN_POINT('',(210.642277625417,586.597556589211,-35.7037040214914)) ;
#70717=CARTESIAN_POINT('',(210.517277625417,586.472556589211,-39.2297690928544)) ;
#70718=CARTESIAN_POINT('Origin',(210.517277625417,586.597556589211,-39.2297690928544)) ;
#70719=CARTESIAN_POINT('',(210.517277625417,586.472556589211,-35.7037040214914)) ;
#70720=CARTESIAN_POINT('Origin',(210.642277625417,583.868806589211,-33.4492690928543)) ;
#70721=CARTESIAN_POINT('',(210.642277625417,590.347556589211,-39.2297690928544)) ;
#70722=CARTESIAN_POINT('',(210.642277625417,590.347556589211,-33.7350190928543)) ;
#70723=CARTESIAN_POINT('',(210.642277625417,586.488181589211,-39.2297690928544)) ;
#70724=CARTESIAN_POINT('Origin',(210.517277625417,590.347556589211,-33.7350190928543)) ;
#70725=CARTESIAN_POINT('',(210.517277625417,590.472556589211,-39.2297690928544)) ;
#70726=CARTESIAN_POINT('',(210.517277625417,590.472556589211,-33.7350190928543)) ;
#70727=CARTESIAN_POINT('Origin',(210.517277625417,590.347556589211,-39.2297690928544)) ;
#70728=CARTESIAN_POINT('Origin',(197.307277625417,590.472556589211,-34.0207690928544)) ;
#70729=CARTESIAN_POINT('',(209.814777625417,590.472556589211,-39.2297690928544)) ;
#70730=CARTESIAN_POINT('',(209.814777625417,590.472556589211,-38.5610190928544)) ;
#70731=CARTESIAN_POINT('',(207.753027625417,590.472556589211,-39.2297690928544)) ;
#70732=CARTESIAN_POINT('Origin',(201.57290262541,581.222556589211,-35.2721601717607)) ;
#70733=CARTESIAN_POINT('',(209.814777625407,581.222556589211,-35.0221601717611)) ;
#70734=CARTESIAN_POINT('',(209.814777625407,580.972556589211,-35.2721601717611)) ;
#70735=CARTESIAN_POINT('Origin',(209.814777625407,581.222556589211,-35.2721601717611)) ;
#70736=CARTESIAN_POINT('',(210.517277625407,580.972556589211,-35.2721601717611)) ;
#70737=CARTESIAN_POINT('',(201.57290262541,580.972556589211,-35.2721601717607)) ;
#70738=CARTESIAN_POINT('',(210.517277625407,581.222556589211,-35.0221601717611)) ;
#70739=CARTESIAN_POINT('Origin',(210.517277625407,581.222556589211,-35.2721601717611)) ;
#70740=CARTESIAN_POINT('',(201.57290262541,581.222556589211,-35.0221601717607)) ;
#70741=CARTESIAN_POINT('Origin',(210.517277625407,580.847556589211,-35.2721601717609)) ;
#70742=CARTESIAN_POINT('',(210.642277625407,580.847556589211,-35.2721601717609)) ;
#70743=CARTESIAN_POINT('',(210.892277625407,580.847556589211,-35.0221601717612)) ;
#70744=CARTESIAN_POINT('Origin',(210.892277625407,580.847556589211,-35.2721601717609)) ;
#70745=CARTESIAN_POINT('Origin',(210.517277625407,580.847556589211,-35.0221601717611)) ;
#70746=CARTESIAN_POINT('Origin',(210.517277625407,580.847556589211,-35.2721601717609)) ;
#70747=CARTESIAN_POINT('Origin',(210.892277625407,595.670681589221,-35.2721601717611)) ;
#70748=CARTESIAN_POINT('',(210.642277625407,577.097556589211,-35.2721601717612)) ;
#70749=CARTESIAN_POINT('',(210.892277625407,577.097556589211,-35.0221601717612)) ;
#70750=CARTESIAN_POINT('Origin',(210.892277625407,577.097556589211,-35.2721601717612)) ;
#70751=CARTESIAN_POINT('',(210.892277625407,595.670681589221,-35.0221601717611)) ;
#70752=CARTESIAN_POINT('',(210.642277625415,595.670681589221,-35.2721601717611)) ;
#70753=CARTESIAN_POINT('Origin',(210.517277625407,577.097556589211,-35.2721601717609)) ;
#70754=CARTESIAN_POINT('',(210.517277625407,576.972556589211,-35.2721601717609)) ;
#70755=CARTESIAN_POINT('',(210.517277625407,576.722556589211,-35.0221601717611)) ;
#70756=CARTESIAN_POINT('Origin',(210.517277625407,576.722556589211,-35.2721601717609)) ;
#70757=CARTESIAN_POINT('Origin',(210.517277625407,577.097556589211,-35.0221601717611)) ;
#70758=CARTESIAN_POINT('Origin',(210.517277625407,577.097556589211,-35.2721601717609)) ;
#70759=CARTESIAN_POINT('Origin',(205.938476772278,576.722556589211,-35.2721601717609)) ;
#70760=CARTESIAN_POINT('',(209.814777625407,576.972556589211,-35.2721601717611)) ;
#70761=CARTESIAN_POINT('',(209.814777625407,576.722556589211,-35.0221601717611)) ;
#70762=CARTESIAN_POINT('Origin',(209.814777625407,576.722556589211,-35.2721601717611)) ;
#70763=CARTESIAN_POINT('',(205.938476772278,576.722556589211,-35.0221601717609)) ;
#70764=CARTESIAN_POINT('',(205.938476772278,576.972556589211,-35.2721601717609)) ;
#70765=CARTESIAN_POINT('Origin',(209.814777625407,577.097556589211,-35.2721601717609)) ;
#70766=CARTESIAN_POINT('',(209.689777625407,577.097556589211,-35.2721601717609)) ;
#70767=CARTESIAN_POINT('',(209.439777625407,577.097556589211,-35.0221601717611)) ;
#70768=CARTESIAN_POINT('Origin',(209.439777625407,577.097556589211,-35.2721601717609)) ;
#70769=CARTESIAN_POINT('Origin',(209.814777625407,577.097556589211,-35.0221601717611)) ;
#70770=CARTESIAN_POINT('Origin',(209.814777625407,577.097556589211,-35.2721601717609)) ;
#70771=CARTESIAN_POINT('Origin',(209.439777625407,595.670681589221,-35.2721601717611)) ;
#70772=CARTESIAN_POINT('',(209.689777625407,580.847556589211,-35.2721601717611)) ;
#70773=CARTESIAN_POINT('',(209.439777625407,580.847556589211,-35.0221601717611)) ;
#70774=CARTESIAN_POINT('Origin',(209.439777625407,580.847556589211,-35.2721601717611)) ;
#70775=CARTESIAN_POINT('',(209.439777625407,595.670681589221,-35.0221601717611)) ;
#70776=CARTESIAN_POINT('',(209.689777625415,595.670681589221,-35.2721601717611)) ;
#70777=CARTESIAN_POINT('Origin',(209.814777625407,580.847556589211,-35.2721601717609)) ;
#70778=CARTESIAN_POINT('Origin',(209.814777625407,580.847556589211,-35.0221601717611)) ;
#70779=CARTESIAN_POINT('Origin',(209.814777625407,580.847556589211,-35.2721601717609)) ;
#70780=CARTESIAN_POINT('Origin',(210.517277625416,577.097556589211,-35.7037040214914)) ;
#70781=CARTESIAN_POINT('',(210.642277625416,577.097556589211,-39.2297690928544)) ;
#70782=CARTESIAN_POINT('',(210.642277625416,577.097556589211,-35.7037040214914)) ;
#70783=CARTESIAN_POINT('',(210.517277625416,576.972556589211,-39.2297690928544)) ;
#70784=CARTESIAN_POINT('Origin',(210.517277625416,577.097556589211,-39.2297690928544)) ;
#70785=CARTESIAN_POINT('',(210.517277625416,576.972556589211,-35.7037040214914)) ;
#70786=CARTESIAN_POINT('Origin',(210.642277625415,574.368806589211,-33.4492690928543)) ;
#70787=CARTESIAN_POINT('',(210.642277625416,580.847556589211,-39.2297690928544)) ;
#70788=CARTESIAN_POINT('',(210.642277625415,580.847556589211,-33.7350190928543)) ;
#70789=CARTESIAN_POINT('',(210.642277625416,576.988181589211,-39.2297690928544)) ;
#70790=CARTESIAN_POINT('Origin',(210.517277625415,580.847556589211,-33.7350190928543)) ;
#70791=CARTESIAN_POINT('',(210.517277625416,580.972556589211,-39.2297690928544)) ;
#70792=CARTESIAN_POINT('',(210.517277625415,580.972556589211,-33.7350190928543)) ;
#70793=CARTESIAN_POINT('Origin',(210.517277625416,580.847556589211,-39.2297690928544)) ;
#70794=CARTESIAN_POINT('Origin',(197.307277625415,580.972556589211,-34.0207690928544)) ;
#70795=CARTESIAN_POINT('',(209.814777625415,580.972556589211,-39.2297690928544)) ;
#70796=CARTESIAN_POINT('',(209.814777625415,580.972556589211,-38.5610190928544)) ;
#70797=CARTESIAN_POINT('',(207.753027625415,580.972556589211,-39.2297690928544)) ;
#70798=CARTESIAN_POINT('Origin',(201.57290262541,571.722556589211,-35.2721601717607)) ;
#70799=CARTESIAN_POINT('',(209.814777625407,571.722556589211,-35.0221601717611)) ;
#70800=CARTESIAN_POINT('',(209.814777625407,571.472556589211,-35.2721601717611)) ;
#70801=CARTESIAN_POINT('Origin',(209.814777625407,571.722556589211,-35.2721601717611)) ;
#70802=CARTESIAN_POINT('',(210.517277625407,571.472556589211,-35.2721601717611)) ;
#70803=CARTESIAN_POINT('',(201.57290262541,571.472556589211,-35.2721601717607)) ;
#70804=CARTESIAN_POINT('',(210.517277625407,571.722556589211,-35.0221601717611)) ;
#70805=CARTESIAN_POINT('Origin',(210.517277625407,571.722556589211,-35.2721601717611)) ;
#70806=CARTESIAN_POINT('',(201.57290262541,571.722556589211,-35.0221601717607)) ;
#70807=CARTESIAN_POINT('Origin',(210.517277625407,571.347556589211,-35.2721601717609)) ;
#70808=CARTESIAN_POINT('',(210.642277625407,571.347556589211,-35.2721601717609)) ;
#70809=CARTESIAN_POINT('',(210.892277625407,571.347556589211,-35.0221601717612)) ;
#70810=CARTESIAN_POINT('Origin',(210.892277625407,571.347556589211,-35.2721601717609)) ;
#70811=CARTESIAN_POINT('Origin',(210.517277625407,571.347556589211,-35.0221601717611)) ;
#70812=CARTESIAN_POINT('Origin',(210.517277625407,571.347556589211,-35.2721601717609)) ;
#70813=CARTESIAN_POINT('Origin',(210.892277625407,586.170681589221,-35.2721601717611)) ;
#70814=CARTESIAN_POINT('',(210.642277625407,567.59755658921,-35.2721601717612)) ;
#70815=CARTESIAN_POINT('',(210.892277625407,567.59755658921,-35.0221601717612)) ;
#70816=CARTESIAN_POINT('Origin',(210.892277625407,567.59755658921,-35.2721601717612)) ;
#70817=CARTESIAN_POINT('',(210.892277625407,586.170681589221,-35.0221601717611)) ;
#70818=CARTESIAN_POINT('',(210.642277625414,586.170681589221,-35.2721601717611)) ;
#70819=CARTESIAN_POINT('Origin',(210.517277625407,567.59755658921,-35.2721601717609)) ;
#70820=CARTESIAN_POINT('',(210.517277625407,567.472556589211,-35.2721601717609)) ;
#70821=CARTESIAN_POINT('',(210.517277625407,567.222556589211,-35.0221601717611)) ;
#70822=CARTESIAN_POINT('Origin',(210.517277625407,567.222556589211,-35.2721601717609)) ;
#70823=CARTESIAN_POINT('Origin',(210.517277625407,567.59755658921,-35.0221601717611)) ;
#70824=CARTESIAN_POINT('Origin',(210.517277625407,567.59755658921,-35.2721601717609)) ;
#70825=CARTESIAN_POINT('Origin',(205.938476772278,567.222556589211,-35.2721601717609)) ;
#70826=CARTESIAN_POINT('',(209.814777625407,567.472556589211,-35.2721601717611)) ;
#70827=CARTESIAN_POINT('',(209.814777625407,567.222556589211,-35.0221601717611)) ;
#70828=CARTESIAN_POINT('Origin',(209.814777625407,567.222556589211,-35.2721601717611)) ;
#70829=CARTESIAN_POINT('',(205.938476772278,567.222556589211,-35.0221601717609)) ;
#70830=CARTESIAN_POINT('',(205.938476772278,567.47255658921,-35.2721601717609)) ;
#70831=CARTESIAN_POINT('Origin',(209.814777625407,567.597556589211,-35.2721601717609)) ;
#70832=CARTESIAN_POINT('',(209.689777625407,567.597556589211,-35.2721601717609)) ;
#70833=CARTESIAN_POINT('',(209.439777625407,567.597556589211,-35.0221601717611)) ;
#70834=CARTESIAN_POINT('Origin',(209.439777625407,567.597556589211,-35.2721601717609)) ;
#70835=CARTESIAN_POINT('Origin',(209.814777625407,567.597556589211,-35.0221601717611)) ;
#70836=CARTESIAN_POINT('Origin',(209.814777625407,567.597556589211,-35.2721601717609)) ;
#70837=CARTESIAN_POINT('Origin',(209.439777625407,586.170681589221,-35.2721601717611)) ;
#70838=CARTESIAN_POINT('',(209.689777625407,571.347556589211,-35.2721601717611)) ;
#70839=CARTESIAN_POINT('',(209.439777625407,571.347556589211,-35.0221601717611)) ;
#70840=CARTESIAN_POINT('Origin',(209.439777625407,571.347556589211,-35.2721601717611)) ;
#70841=CARTESIAN_POINT('',(209.439777625407,586.170681589221,-35.0221601717611)) ;
#70842=CARTESIAN_POINT('',(209.689777625413,586.170681589221,-35.2721601717611)) ;
#70843=CARTESIAN_POINT('Origin',(209.814777625407,571.347556589211,-35.2721601717609)) ;
#70844=CARTESIAN_POINT('Origin',(209.814777625407,571.347556589211,-35.0221601717611)) ;
#70845=CARTESIAN_POINT('Origin',(209.814777625407,571.347556589211,-35.2721601717609)) ;
#70846=CARTESIAN_POINT('Origin',(210.517277625414,567.59755658921,-35.7037040214914)) ;
#70847=CARTESIAN_POINT('',(210.642277625414,567.59755658921,-39.2297690928544)) ;
#70848=CARTESIAN_POINT('',(210.642277625414,567.59755658921,-35.7037040214914)) ;
#70849=CARTESIAN_POINT('',(210.517277625414,567.47255658921,-39.2297690928544)) ;
#70850=CARTESIAN_POINT('Origin',(210.517277625414,567.59755658921,-39.2297690928544)) ;
#70851=CARTESIAN_POINT('',(210.517277625414,567.47255658921,-35.7037040214914)) ;
#70852=CARTESIAN_POINT('Origin',(210.642277625414,564.868806589211,-33.4492690928543)) ;
#70853=CARTESIAN_POINT('',(210.642277625414,571.347556589211,-39.2297690928544)) ;
#70854=CARTESIAN_POINT('',(210.642277625414,571.347556589211,-33.7350190928543)) ;
#70855=CARTESIAN_POINT('',(210.642277625414,567.488181589211,-39.2297690928544)) ;
#70856=CARTESIAN_POINT('Origin',(210.517277625414,571.347556589211,-33.7350190928543)) ;
#70857=CARTESIAN_POINT('',(210.517277625414,571.472556589211,-39.2297690928544)) ;
#70858=CARTESIAN_POINT('',(210.517277625414,571.472556589211,-33.7350190928543)) ;
#70859=CARTESIAN_POINT('Origin',(210.517277625414,571.347556589211,-39.2297690928544)) ;
#70860=CARTESIAN_POINT('Origin',(197.307277625413,571.472556589211,-34.0207690928544)) ;
#70861=CARTESIAN_POINT('',(209.814777625413,571.472556589211,-39.2297690928544)) ;
#70862=CARTESIAN_POINT('',(209.814777625413,571.472556589211,-38.5610190928544)) ;
#70863=CARTESIAN_POINT('',(207.753027625413,571.472556589211,-39.2297690928544)) ;
#70864=CARTESIAN_POINT('Origin',(201.57290262541,562.222556589211,-35.2721601717607)) ;
#70865=CARTESIAN_POINT('',(209.814777625407,562.222556589211,-35.0221601717611)) ;
#70866=CARTESIAN_POINT('',(209.814777625407,561.972556589211,-35.2721601717611)) ;
#70867=CARTESIAN_POINT('Origin',(209.814777625407,562.222556589211,-35.2721601717611)) ;
#70868=CARTESIAN_POINT('',(210.517277625407,561.972556589211,-35.2721601717611)) ;
#70869=CARTESIAN_POINT('',(201.57290262541,561.972556589211,-35.2721601717607)) ;
#70870=CARTESIAN_POINT('',(210.517277625407,562.222556589211,-35.0221601717611)) ;
#70871=CARTESIAN_POINT('Origin',(210.517277625407,562.222556589211,-35.2721601717611)) ;
#70872=CARTESIAN_POINT('',(201.57290262541,562.222556589211,-35.0221601717607)) ;
#70873=CARTESIAN_POINT('Origin',(210.517277625407,561.847556589211,-35.2721601717609)) ;
#70874=CARTESIAN_POINT('',(210.642277625407,561.847556589211,-35.2721601717609)) ;
#70875=CARTESIAN_POINT('',(210.892277625407,561.847556589211,-35.0221601717612)) ;
#70876=CARTESIAN_POINT('Origin',(210.892277625407,561.847556589211,-35.2721601717609)) ;
#70877=CARTESIAN_POINT('Origin',(210.517277625407,561.847556589211,-35.0221601717611)) ;
#70878=CARTESIAN_POINT('Origin',(210.517277625407,561.847556589211,-35.2721601717609)) ;
#70879=CARTESIAN_POINT('Origin',(210.892277625407,576.670681589221,-35.2721601717611)) ;
#70880=CARTESIAN_POINT('',(210.642277625407,558.09755658921,-35.2721601717612)) ;
#70881=CARTESIAN_POINT('',(210.892277625407,558.09755658921,-35.0221601717612)) ;
#70882=CARTESIAN_POINT('Origin',(210.892277625407,558.09755658921,-35.2721601717612)) ;
#70883=CARTESIAN_POINT('',(210.892277625407,576.670681589221,-35.0221601717611)) ;
#70884=CARTESIAN_POINT('',(210.642277625412,576.670681589221,-35.2721601717611)) ;
#70885=CARTESIAN_POINT('Origin',(210.517277625407,558.09755658921,-35.2721601717609)) ;
#70886=CARTESIAN_POINT('',(210.517277625407,557.97255658921,-35.2721601717609)) ;
#70887=CARTESIAN_POINT('',(210.517277625407,557.722556589211,-35.0221601717611)) ;
#70888=CARTESIAN_POINT('Origin',(210.517277625407,557.722556589211,-35.2721601717609)) ;
#70889=CARTESIAN_POINT('Origin',(210.517277625407,558.09755658921,-35.0221601717611)) ;
#70890=CARTESIAN_POINT('Origin',(210.517277625407,558.09755658921,-35.2721601717609)) ;
#70891=CARTESIAN_POINT('Origin',(205.938476772278,557.722556589211,-35.2721601717609)) ;
#70892=CARTESIAN_POINT('',(209.814777625407,557.97255658921,-35.2721601717611)) ;
#70893=CARTESIAN_POINT('',(209.814777625407,557.722556589211,-35.0221601717611)) ;
#70894=CARTESIAN_POINT('Origin',(209.814777625407,557.722556589211,-35.2721601717611)) ;
#70895=CARTESIAN_POINT('',(205.938476772278,557.722556589211,-35.0221601717609)) ;
#70896=CARTESIAN_POINT('',(205.938476772278,557.97255658921,-35.2721601717609)) ;
#70897=CARTESIAN_POINT('Origin',(209.814777625407,558.097556589211,-35.2721601717609)) ;
#70898=CARTESIAN_POINT('',(209.689777625407,558.097556589211,-35.2721601717609)) ;
#70899=CARTESIAN_POINT('',(209.439777625407,558.097556589211,-35.0221601717611)) ;
#70900=CARTESIAN_POINT('Origin',(209.439777625407,558.097556589211,-35.2721601717609)) ;
#70901=CARTESIAN_POINT('Origin',(209.814777625407,558.097556589211,-35.0221601717611)) ;
#70902=CARTESIAN_POINT('Origin',(209.814777625407,558.097556589211,-35.2721601717609)) ;
#70903=CARTESIAN_POINT('Origin',(209.439777625407,576.670681589221,-35.2721601717611)) ;
#70904=CARTESIAN_POINT('',(209.689777625407,561.847556589211,-35.2721601717611)) ;
#70905=CARTESIAN_POINT('',(209.439777625407,561.847556589211,-35.0221601717611)) ;
#70906=CARTESIAN_POINT('Origin',(209.439777625407,561.847556589211,-35.2721601717611)) ;
#70907=CARTESIAN_POINT('',(209.439777625407,576.670681589221,-35.0221601717611)) ;
#70908=CARTESIAN_POINT('',(209.689777625412,576.670681589221,-35.2721601717611)) ;
#70909=CARTESIAN_POINT('Origin',(209.814777625407,561.847556589211,-35.2721601717609)) ;
#70910=CARTESIAN_POINT('Origin',(209.814777625407,561.847556589211,-35.0221601717611)) ;
#70911=CARTESIAN_POINT('Origin',(209.814777625407,561.847556589211,-35.2721601717609)) ;
#70912=CARTESIAN_POINT('Origin',(210.517277625412,558.09755658921,-35.7037040214914)) ;
#70913=CARTESIAN_POINT('',(210.642277625412,558.097556589211,-39.2297690928544)) ;
#70914=CARTESIAN_POINT('',(210.642277625412,558.09755658921,-35.7037040214914)) ;
#70915=CARTESIAN_POINT('',(210.517277625412,557.97255658921,-39.2297690928544)) ;
#70916=CARTESIAN_POINT('Origin',(210.517277625412,558.097556589211,-39.2297690928544)) ;
#70917=CARTESIAN_POINT('',(210.517277625412,557.97255658921,-35.7037040214914)) ;
#70918=CARTESIAN_POINT('Origin',(210.642277625412,555.368806589211,-33.4492690928543)) ;
#70919=CARTESIAN_POINT('',(210.642277625412,561.847556589211,-39.2297690928544)) ;
#70920=CARTESIAN_POINT('',(210.642277625412,561.847556589211,-33.7350190928543)) ;
#70921=CARTESIAN_POINT('',(210.642277625412,557.988181589211,-39.2297690928544)) ;
#70922=CARTESIAN_POINT('Origin',(210.517277625412,561.847556589211,-33.7350190928543)) ;
#70923=CARTESIAN_POINT('',(210.517277625412,561.972556589211,-39.2297690928544)) ;
#70924=CARTESIAN_POINT('',(210.517277625412,561.972556589211,-33.7350190928543)) ;
#70925=CARTESIAN_POINT('Origin',(210.517277625412,561.847556589211,-39.2297690928544)) ;
#70926=CARTESIAN_POINT('Origin',(197.307277625412,561.972556589211,-34.0207690928544)) ;
#70927=CARTESIAN_POINT('',(209.814777625412,561.972556589211,-39.2297690928544)) ;
#70928=CARTESIAN_POINT('',(209.814777625412,561.972556589211,-38.5610190928544)) ;
#70929=CARTESIAN_POINT('',(207.753027625412,561.972556589211,-39.2297690928544)) ;
#70930=CARTESIAN_POINT('Origin',(201.57290262541,552.722556589211,-35.2721601717607)) ;
#70931=CARTESIAN_POINT('',(209.814777625407,552.722556589211,-35.0221601717611)) ;
#70932=CARTESIAN_POINT('',(209.814777625407,552.472556589211,-35.2721601717611)) ;
#70933=CARTESIAN_POINT('Origin',(209.814777625407,552.722556589211,-35.2721601717611)) ;
#70934=CARTESIAN_POINT('',(210.517277625407,552.472556589211,-35.2721601717611)) ;
#70935=CARTESIAN_POINT('',(201.57290262541,552.472556589211,-35.2721601717607)) ;
#70936=CARTESIAN_POINT('',(210.517277625407,552.722556589211,-35.0221601717611)) ;
#70937=CARTESIAN_POINT('Origin',(210.517277625407,552.722556589211,-35.2721601717611)) ;
#70938=CARTESIAN_POINT('',(201.57290262541,552.722556589211,-35.0221601717607)) ;
#70939=CARTESIAN_POINT('Origin',(210.517277625407,552.347556589211,-35.2721601717609)) ;
#70940=CARTESIAN_POINT('',(210.642277625407,552.347556589211,-35.2721601717609)) ;
#70941=CARTESIAN_POINT('',(210.892277625407,552.347556589211,-35.0221601717612)) ;
#70942=CARTESIAN_POINT('Origin',(210.892277625407,552.347556589211,-35.2721601717609)) ;
#70943=CARTESIAN_POINT('Origin',(210.517277625407,552.347556589211,-35.0221601717611)) ;
#70944=CARTESIAN_POINT('Origin',(210.517277625407,552.347556589211,-35.2721601717609)) ;
#70945=CARTESIAN_POINT('Origin',(210.892277625407,567.170681589221,-35.2721601717611)) ;
#70946=CARTESIAN_POINT('',(210.642277625407,548.59755658921,-35.2721601717612)) ;
#70947=CARTESIAN_POINT('',(210.892277625407,548.59755658921,-35.0221601717612)) ;
#70948=CARTESIAN_POINT('Origin',(210.892277625407,548.59755658921,-35.2721601717612)) ;
#70949=CARTESIAN_POINT('',(210.892277625407,567.170681589221,-35.0221601717611)) ;
#70950=CARTESIAN_POINT('',(210.64227762541,567.170681589221,-35.2721601717611)) ;
#70951=CARTESIAN_POINT('Origin',(210.517277625407,548.59755658921,-35.2721601717609)) ;
#70952=CARTESIAN_POINT('',(210.517277625407,548.47255658921,-35.2721601717609)) ;
#70953=CARTESIAN_POINT('',(210.517277625407,548.22255658921,-35.0221601717611)) ;
#70954=CARTESIAN_POINT('Origin',(210.517277625407,548.22255658921,-35.2721601717609)) ;
#70955=CARTESIAN_POINT('Origin',(210.517277625407,548.59755658921,-35.0221601717611)) ;
#70956=CARTESIAN_POINT('Origin',(210.517277625407,548.59755658921,-35.2721601717609)) ;
#70957=CARTESIAN_POINT('Origin',(205.938476772278,548.22255658921,-35.2721601717609)) ;
#70958=CARTESIAN_POINT('',(209.814777625407,548.47255658921,-35.2721601717611)) ;
#70959=CARTESIAN_POINT('',(209.814777625407,548.22255658921,-35.0221601717611)) ;
#70960=CARTESIAN_POINT('Origin',(209.814777625407,548.22255658921,-35.2721601717611)) ;
#70961=CARTESIAN_POINT('',(205.938476772278,548.22255658921,-35.0221601717609)) ;
#70962=CARTESIAN_POINT('',(205.938476772278,548.47255658921,-35.2721601717609)) ;
#70963=CARTESIAN_POINT('Origin',(209.814777625407,548.59755658921,-35.2721601717609)) ;
#70964=CARTESIAN_POINT('',(209.689777625407,548.59755658921,-35.2721601717609)) ;
#70965=CARTESIAN_POINT('',(209.439777625407,548.59755658921,-35.0221601717611)) ;
#70966=CARTESIAN_POINT('Origin',(209.439777625407,548.59755658921,-35.2721601717609)) ;
#70967=CARTESIAN_POINT('Origin',(209.814777625407,548.59755658921,-35.0221601717611)) ;
#70968=CARTESIAN_POINT('Origin',(209.814777625407,548.59755658921,-35.2721601717609)) ;
#70969=CARTESIAN_POINT('Origin',(209.439777625407,567.170681589221,-35.2721601717611)) ;
#70970=CARTESIAN_POINT('',(209.689777625407,552.347556589211,-35.2721601717611)) ;
#70971=CARTESIAN_POINT('',(209.439777625407,552.347556589211,-35.0221601717611)) ;
#70972=CARTESIAN_POINT('Origin',(209.439777625407,552.347556589211,-35.2721601717611)) ;
#70973=CARTESIAN_POINT('',(209.439777625407,567.170681589221,-35.0221601717611)) ;
#70974=CARTESIAN_POINT('',(209.68977762541,567.170681589221,-35.2721601717611)) ;
#70975=CARTESIAN_POINT('Origin',(209.814777625407,552.347556589211,-35.2721601717609)) ;
#70976=CARTESIAN_POINT('Origin',(209.814777625407,552.347556589211,-35.0221601717611)) ;
#70977=CARTESIAN_POINT('Origin',(209.814777625407,552.347556589211,-35.2721601717609)) ;
#70978=CARTESIAN_POINT('Origin',(210.51727762541,548.59755658921,-35.7037040214914)) ;
#70979=CARTESIAN_POINT('',(210.64227762541,548.59755658921,-39.2297690928544)) ;
#70980=CARTESIAN_POINT('',(210.64227762541,548.59755658921,-35.7037040214914)) ;
#70981=CARTESIAN_POINT('',(210.517277625411,548.47255658921,-39.2297690928544)) ;
#70982=CARTESIAN_POINT('Origin',(210.51727762541,548.59755658921,-39.2297690928544)) ;
#70983=CARTESIAN_POINT('',(210.517277625411,548.47255658921,-35.7037040214914)) ;
#70984=CARTESIAN_POINT('Origin',(210.64227762541,545.86880658921,-33.4492690928543)) ;
#70985=CARTESIAN_POINT('',(210.64227762541,552.347556589211,-39.2297690928544)) ;
#70986=CARTESIAN_POINT('',(210.64227762541,552.347556589211,-33.7350190928543)) ;
#70987=CARTESIAN_POINT('',(210.64227762541,548.488181589211,-39.2297690928544)) ;
#70988=CARTESIAN_POINT('Origin',(210.51727762541,552.347556589211,-33.7350190928543)) ;
#70989=CARTESIAN_POINT('',(210.51727762541,552.472556589211,-39.2297690928544)) ;
#70990=CARTESIAN_POINT('',(210.51727762541,552.472556589211,-33.7350190928543)) ;
#70991=CARTESIAN_POINT('Origin',(210.51727762541,552.347556589211,-39.2297690928544)) ;
#70992=CARTESIAN_POINT('Origin',(197.30727762541,552.472556589211,-34.0207690928544)) ;
#70993=CARTESIAN_POINT('',(209.81477762541,552.472556589211,-39.2297690928544)) ;
#70994=CARTESIAN_POINT('',(209.81477762541,552.472556589211,-38.5610190928544)) ;
#70995=CARTESIAN_POINT('',(207.75302762541,552.472556589211,-39.2297690928544)) ;
#70996=CARTESIAN_POINT('Origin',(201.57290262541,543.222556589211,-35.2721601717607)) ;
#70997=CARTESIAN_POINT('',(209.814777625407,543.222556589211,-35.0221601717611)) ;
#70998=CARTESIAN_POINT('',(209.814777625407,542.972556589211,-35.2721601717611)) ;
#70999=CARTESIAN_POINT('Origin',(209.814777625407,543.222556589211,-35.2721601717611)) ;
#71000=CARTESIAN_POINT('',(210.517277625407,542.972556589211,-35.2721601717611)) ;
#71001=CARTESIAN_POINT('',(201.57290262541,542.972556589211,-35.2721601717607)) ;
#71002=CARTESIAN_POINT('',(210.517277625407,543.222556589211,-35.0221601717611)) ;
#71003=CARTESIAN_POINT('Origin',(210.517277625407,543.222556589211,-35.2721601717611)) ;
#71004=CARTESIAN_POINT('',(201.57290262541,543.222556589211,-35.0221601717607)) ;
#71005=CARTESIAN_POINT('Origin',(210.517277625407,542.847556589211,-35.2721601717609)) ;
#71006=CARTESIAN_POINT('',(210.642277625407,542.847556589211,-35.2721601717609)) ;
#71007=CARTESIAN_POINT('',(210.892277625407,542.847556589211,-35.0221601717612)) ;
#71008=CARTESIAN_POINT('Origin',(210.892277625407,542.847556589211,-35.2721601717609)) ;
#71009=CARTESIAN_POINT('Origin',(210.517277625407,542.847556589211,-35.0221601717611)) ;
#71010=CARTESIAN_POINT('Origin',(210.517277625407,542.847556589211,-35.2721601717609)) ;
#71011=CARTESIAN_POINT('Origin',(210.892277625407,557.670681589221,-35.2721601717611)) ;
#71012=CARTESIAN_POINT('',(210.642277625407,539.09755658921,-35.2721601717612)) ;
#71013=CARTESIAN_POINT('',(210.892277625407,539.09755658921,-35.0221601717612)) ;
#71014=CARTESIAN_POINT('Origin',(210.892277625407,539.09755658921,-35.2721601717612)) ;
#71015=CARTESIAN_POINT('',(210.892277625407,557.670681589221,-35.0221601717611)) ;
#71016=CARTESIAN_POINT('',(210.642277625409,557.670681589221,-35.2721601717611)) ;
#71017=CARTESIAN_POINT('Origin',(210.517277625407,539.09755658921,-35.2721601717609)) ;
#71018=CARTESIAN_POINT('',(210.517277625407,538.97255658921,-35.2721601717609)) ;
#71019=CARTESIAN_POINT('',(210.517277625407,538.72255658921,-35.0221601717611)) ;
#71020=CARTESIAN_POINT('Origin',(210.517277625407,538.72255658921,-35.2721601717609)) ;
#71021=CARTESIAN_POINT('Origin',(210.517277625407,539.09755658921,-35.0221601717611)) ;
#71022=CARTESIAN_POINT('Origin',(210.517277625407,539.09755658921,-35.2721601717609)) ;
#71023=CARTESIAN_POINT('Origin',(205.938476772278,538.72255658921,-35.2721601717609)) ;
#71024=CARTESIAN_POINT('',(209.814777625407,538.97255658921,-35.2721601717611)) ;
#71025=CARTESIAN_POINT('',(209.814777625407,538.72255658921,-35.0221601717611)) ;
#71026=CARTESIAN_POINT('Origin',(209.814777625407,538.72255658921,-35.2721601717611)) ;
#71027=CARTESIAN_POINT('',(205.938476772278,538.72255658921,-35.0221601717609)) ;
#71028=CARTESIAN_POINT('',(205.938476772278,538.97255658921,-35.2721601717609)) ;
#71029=CARTESIAN_POINT('Origin',(209.814777625407,539.09755658921,-35.2721601717609)) ;
#71030=CARTESIAN_POINT('',(209.689777625407,539.09755658921,-35.2721601717609)) ;
#71031=CARTESIAN_POINT('',(209.439777625407,539.09755658921,-35.0221601717611)) ;
#71032=CARTESIAN_POINT('Origin',(209.439777625407,539.09755658921,-35.2721601717609)) ;
#71033=CARTESIAN_POINT('Origin',(209.814777625407,539.09755658921,-35.0221601717611)) ;
#71034=CARTESIAN_POINT('Origin',(209.814777625407,539.09755658921,-35.2721601717609)) ;
#71035=CARTESIAN_POINT('Origin',(209.439777625407,557.670681589221,-35.2721601717611)) ;
#71036=CARTESIAN_POINT('',(209.689777625407,542.847556589211,-35.2721601717611)) ;
#71037=CARTESIAN_POINT('',(209.439777625407,542.847556589211,-35.0221601717611)) ;
#71038=CARTESIAN_POINT('Origin',(209.439777625407,542.847556589211,-35.2721601717611)) ;
#71039=CARTESIAN_POINT('',(209.439777625407,557.670681589221,-35.0221601717611)) ;
#71040=CARTESIAN_POINT('',(209.689777625408,557.670681589221,-35.2721601717611)) ;
#71041=CARTESIAN_POINT('Origin',(209.814777625407,542.847556589211,-35.2721601717609)) ;
#71042=CARTESIAN_POINT('Origin',(209.814777625407,542.847556589211,-35.0221601717611)) ;
#71043=CARTESIAN_POINT('Origin',(209.814777625407,542.847556589211,-35.2721601717609)) ;
#71044=CARTESIAN_POINT('Origin',(210.517277625409,539.09755658921,-35.7037040214914)) ;
#71045=CARTESIAN_POINT('',(210.642277625409,539.09755658921,-39.2297690928544)) ;
#71046=CARTESIAN_POINT('',(210.642277625409,539.09755658921,-35.7037040214914)) ;
#71047=CARTESIAN_POINT('',(210.517277625409,538.97255658921,-39.2297690928544)) ;
#71048=CARTESIAN_POINT('Origin',(210.517277625409,539.09755658921,-39.2297690928544)) ;
#71049=CARTESIAN_POINT('',(210.517277625409,538.97255658921,-35.7037040214914)) ;
#71050=CARTESIAN_POINT('Origin',(210.642277625409,536.36880658921,-33.4492690928543)) ;
#71051=CARTESIAN_POINT('',(210.642277625409,542.847556589211,-39.2297690928544)) ;
#71052=CARTESIAN_POINT('',(210.642277625409,542.847556589211,-33.7350190928543)) ;
#71053=CARTESIAN_POINT('',(210.642277625409,538.988181589211,-39.2297690928544)) ;
#71054=CARTESIAN_POINT('Origin',(210.517277625409,542.847556589211,-33.7350190928543)) ;
#71055=CARTESIAN_POINT('',(210.517277625409,542.972556589211,-39.2297690928544)) ;
#71056=CARTESIAN_POINT('',(210.517277625409,542.972556589211,-33.7350190928543)) ;
#71057=CARTESIAN_POINT('Origin',(210.517277625409,542.847556589211,-39.2297690928544)) ;
#71058=CARTESIAN_POINT('Origin',(197.307277625408,542.972556589211,-34.0207690928544)) ;
#71059=CARTESIAN_POINT('',(209.814777625408,542.972556589211,-39.2297690928544)) ;
#71060=CARTESIAN_POINT('',(209.814777625408,542.972556589211,-38.5610190928544)) ;
#71061=CARTESIAN_POINT('',(207.753027625408,542.972556589211,-39.2297690928544)) ;
#71062=CARTESIAN_POINT('Origin',(201.57290262541,609.722556589211,-35.2721601717607)) ;
#71063=CARTESIAN_POINT('',(201.559777625407,609.722556589211,-35.0221601717607)) ;
#71064=CARTESIAN_POINT('',(201.559777625407,609.472556589211,-35.2721601717607)) ;
#71065=CARTESIAN_POINT('Origin',(201.559777625407,609.722556589211,-35.2721601717607)) ;
#71066=CARTESIAN_POINT('',(202.262277625407,609.472556589211,-35.2721601717608)) ;
#71067=CARTESIAN_POINT('',(201.57290262541,609.472556589211,-35.2721601717607)) ;
#71068=CARTESIAN_POINT('',(202.262277625407,609.722556589211,-35.0221601717608)) ;
#71069=CARTESIAN_POINT('Origin',(202.262277625407,609.722556589211,-35.2721601717608)) ;
#71070=CARTESIAN_POINT('',(201.57290262541,609.722556589211,-35.0221601717607)) ;
#71071=CARTESIAN_POINT('Origin',(202.262277625407,609.347556589211,-35.2721601717609)) ;
#71072=CARTESIAN_POINT('',(202.387277625407,609.347556589211,-35.2721601717609)) ;
#71073=CARTESIAN_POINT('',(202.637277625407,609.347556589211,-35.0221601717608)) ;
#71074=CARTESIAN_POINT('Origin',(202.637277625407,609.347556589211,-35.2721601717609)) ;
#71075=CARTESIAN_POINT('Origin',(202.262277625407,609.347556589211,-35.0221601717607)) ;
#71076=CARTESIAN_POINT('Origin',(202.262277625407,609.347556589211,-35.2721601717609)) ;
#71077=CARTESIAN_POINT('Origin',(202.637277625407,624.170681589221,-35.2721601717608)) ;
#71078=CARTESIAN_POINT('',(202.387277625407,605.597556589211,-35.2721601717608)) ;
#71079=CARTESIAN_POINT('',(202.637277625407,605.597556589211,-35.0221601717608)) ;
#71080=CARTESIAN_POINT('Origin',(202.637277625407,605.597556589211,-35.2721601717608)) ;
#71081=CARTESIAN_POINT('',(202.637277625407,624.170681589221,-35.0221601717608)) ;
#71082=CARTESIAN_POINT('',(202.38727762542,624.170681589221,-35.2721601717608)) ;
#71083=CARTESIAN_POINT('Origin',(202.262277625407,605.597556589211,-35.2721601717609)) ;
#71084=CARTESIAN_POINT('',(202.262277625407,605.472556589211,-35.2721601717609)) ;
#71085=CARTESIAN_POINT('',(202.262277625407,605.222556589211,-35.0221601717608)) ;
#71086=CARTESIAN_POINT('Origin',(202.262277625407,605.222556589211,-35.2721601717609)) ;
#71087=CARTESIAN_POINT('Origin',(202.262277625407,605.597556589211,-35.0221601717607)) ;
#71088=CARTESIAN_POINT('Origin',(202.262277625407,605.597556589211,-35.2721601717609)) ;
#71089=CARTESIAN_POINT('Origin',(205.938476772278,605.222556589211,-35.2721601717609)) ;
#71090=CARTESIAN_POINT('',(201.559777625407,605.472556589211,-35.2721601717607)) ;
#71091=CARTESIAN_POINT('',(201.559777625407,605.222556589211,-35.0221601717607)) ;
#71092=CARTESIAN_POINT('Origin',(201.559777625407,605.222556589211,-35.2721601717607)) ;
#71093=CARTESIAN_POINT('',(205.938476772278,605.222556589211,-35.0221601717609)) ;
#71094=CARTESIAN_POINT('',(205.938476772278,605.472556589211,-35.2721601717609)) ;
#71095=CARTESIAN_POINT('Origin',(201.559777625407,605.597556589211,-35.2721601717609)) ;
#71096=CARTESIAN_POINT('',(201.184777625407,605.597556589211,-35.0221601717607)) ;
#71097=CARTESIAN_POINT('Origin',(201.184777625407,605.597556589211,-35.2721601717609)) ;
#71098=CARTESIAN_POINT('Origin',(201.559777625407,605.597556589211,-35.0221601717607)) ;
#71099=CARTESIAN_POINT('Origin',(201.559777625407,605.597556589211,-35.2721601717609)) ;
#71100=CARTESIAN_POINT('Origin',(201.184777625407,624.170681589221,-35.2721601717607)) ;
#71101=CARTESIAN_POINT('',(201.184777625407,609.347556589211,-35.0221601717607)) ;
#71102=CARTESIAN_POINT('Origin',(201.184777625407,609.347556589211,-35.2721601717607)) ;
#71103=CARTESIAN_POINT('',(201.184777625407,624.170681589221,-35.0221601717607)) ;
#71104=CARTESIAN_POINT('Origin',(201.559777625407,609.347556589211,-35.2721601717609)) ;
#71105=CARTESIAN_POINT('Origin',(201.559777625407,609.347556589211,-35.0221601717607)) ;
#71106=CARTESIAN_POINT('Origin',(201.559777625407,609.347556589211,-35.2721601717609)) ;
#71107=CARTESIAN_POINT('Origin',(202.26227762542,605.597556589211,-35.8624540214915)) ;
#71108=CARTESIAN_POINT('',(202.38727762542,605.597556589211,-39.2297700580612)) ;
#71109=CARTESIAN_POINT('',(202.38727762542,605.597556589211,-35.8624540214915)) ;
#71110=CARTESIAN_POINT('',(202.26227762542,605.472556589211,-39.2297700580612)) ;
#71111=CARTESIAN_POINT('Origin',(202.26227762542,605.597556589211,-39.2297700580612)) ;
#71112=CARTESIAN_POINT('',(202.26227762542,605.472556589211,-35.8624540214915)) ;
#71113=CARTESIAN_POINT('Origin',(202.38727762542,602.868806589211,-33.7667690928544)) ;
#71114=CARTESIAN_POINT('',(202.38727762542,606.962556589212,-39.4182700580611)) ;
#71115=CARTESIAN_POINT('',(202.38727762542,606.962556589212,-37.6444650424525)) ;
#71116=CARTESIAN_POINT('',(202.38727762542,606.774056589212,-39.2297700580612)) ;
#71117=CARTESIAN_POINT('Origin',(202.38727762542,606.774056589212,-39.4182700580611)) ;
#71118=CARTESIAN_POINT('',(202.38727762542,605.488181589211,-39.2297700580612)) ;
#71119=CARTESIAN_POINT('',(202.38727762542,609.347556589211,-39.2297700580612)) ;
#71120=CARTESIAN_POINT('',(202.38727762542,609.347556589211,-33.8937690928544)) ;
#71121=CARTESIAN_POINT('',(202.38727762542,608.171056589212,-39.2297700580612)) ;
#71122=CARTESIAN_POINT('',(202.38727762542,605.488181589211,-39.2297700580612)) ;
#71123=CARTESIAN_POINT('',(202.38727762542,607.982556589212,-39.4182700580611)) ;
#71124=CARTESIAN_POINT('Origin',(202.38727762542,608.171056589212,-39.4182700580612)) ;
#71125=CARTESIAN_POINT('',(202.38727762542,607.982556589212,-39.8669650424525)) ;
#71126=CARTESIAN_POINT('Origin',(202.26227762542,609.347556589211,-33.8937690928544)) ;
#71127=CARTESIAN_POINT('',(202.26227762542,609.472556589211,-39.2297700580612)) ;
#71128=CARTESIAN_POINT('',(202.26227762542,609.472556589211,-33.8937690928544)) ;
#71129=CARTESIAN_POINT('Origin',(202.26227762542,609.347556589211,-39.2297700580612)) ;
#71130=CARTESIAN_POINT('Origin',(197.30727762542,609.472556589211,-34.0207690928544)) ;
#71131=CARTESIAN_POINT('',(201.55977762542,609.472556589211,-39.2297700580612)) ;
#71132=CARTESIAN_POINT('',(201.55977762542,609.472556589211,-38.5610190928544)) ;
#71133=CARTESIAN_POINT('',(207.75302762542,609.472556589211,-39.2297700580612)) ;
#71134=CARTESIAN_POINT('Origin',(201.57290262541,600.222556589211,-35.2721601717607)) ;
#71135=CARTESIAN_POINT('',(201.559777625407,600.222556589211,-35.0221601717607)) ;
#71136=CARTESIAN_POINT('',(201.559777625407,599.972556589211,-35.2721601717607)) ;
#71137=CARTESIAN_POINT('Origin',(201.559777625407,600.222556589211,-35.2721601717607)) ;
#71138=CARTESIAN_POINT('',(202.262277625407,599.972556589211,-35.2721601717608)) ;
#71139=CARTESIAN_POINT('',(201.57290262541,599.972556589211,-35.2721601717607)) ;
#71140=CARTESIAN_POINT('',(202.262277625407,600.222556589211,-35.0221601717608)) ;
#71141=CARTESIAN_POINT('Origin',(202.262277625407,600.222556589211,-35.2721601717608)) ;
#71142=CARTESIAN_POINT('',(201.57290262541,600.222556589211,-35.0221601717607)) ;
#71143=CARTESIAN_POINT('Origin',(202.262277625407,599.847556589211,-35.2721601717609)) ;
#71144=CARTESIAN_POINT('',(202.387277625407,599.847556589211,-35.2721601717609)) ;
#71145=CARTESIAN_POINT('',(202.637277625407,599.847556589211,-35.0221601717608)) ;
#71146=CARTESIAN_POINT('Origin',(202.637277625407,599.847556589211,-35.2721601717609)) ;
#71147=CARTESIAN_POINT('Origin',(202.262277625407,599.847556589211,-35.0221601717607)) ;
#71148=CARTESIAN_POINT('Origin',(202.262277625407,599.847556589211,-35.2721601717609)) ;
#71149=CARTESIAN_POINT('Origin',(202.637277625407,614.670681589221,-35.2721601717608)) ;
#71150=CARTESIAN_POINT('',(202.387277625407,596.097556589211,-35.2721601717608)) ;
#71151=CARTESIAN_POINT('',(202.637277625407,596.097556589211,-35.0221601717608)) ;
#71152=CARTESIAN_POINT('Origin',(202.637277625407,596.097556589211,-35.2721601717608)) ;
#71153=CARTESIAN_POINT('',(202.637277625407,614.670681589221,-35.0221601717608)) ;
#71154=CARTESIAN_POINT('',(202.387277625418,614.670681589221,-35.2721601717608)) ;
#71155=CARTESIAN_POINT('Origin',(202.262277625407,596.097556589211,-35.2721601717609)) ;
#71156=CARTESIAN_POINT('',(202.262277625407,595.972556589211,-35.2721601717609)) ;
#71157=CARTESIAN_POINT('',(202.262277625407,595.722556589211,-35.0221601717608)) ;
#71158=CARTESIAN_POINT('Origin',(202.262277625407,595.722556589211,-35.2721601717609)) ;
#71159=CARTESIAN_POINT('Origin',(202.262277625407,596.097556589211,-35.0221601717607)) ;
#71160=CARTESIAN_POINT('Origin',(202.262277625407,596.097556589211,-35.2721601717609)) ;
#71161=CARTESIAN_POINT('Origin',(205.938476772278,595.722556589211,-35.2721601717609)) ;
#71162=CARTESIAN_POINT('',(201.559777625407,595.972556589211,-35.2721601717607)) ;
#71163=CARTESIAN_POINT('',(201.559777625407,595.722556589211,-35.0221601717607)) ;
#71164=CARTESIAN_POINT('Origin',(201.559777625407,595.722556589211,-35.2721601717607)) ;
#71165=CARTESIAN_POINT('',(205.938476772278,595.722556589211,-35.0221601717609)) ;
#71166=CARTESIAN_POINT('',(205.938476772278,595.972556589211,-35.2721601717609)) ;
#71167=CARTESIAN_POINT('Origin',(201.559777625407,596.097556589211,-35.2721601717609)) ;
#71168=CARTESIAN_POINT('',(201.184777625407,596.097556589211,-35.0221601717607)) ;
#71169=CARTESIAN_POINT('Origin',(201.184777625407,596.097556589211,-35.2721601717609)) ;
#71170=CARTESIAN_POINT('Origin',(201.559777625407,596.097556589211,-35.0221601717607)) ;
#71171=CARTESIAN_POINT('Origin',(201.559777625407,596.097556589211,-35.2721601717609)) ;
#71172=CARTESIAN_POINT('Origin',(201.184777625407,614.670681589221,-35.2721601717607)) ;
#71173=CARTESIAN_POINT('',(201.184777625407,599.847556589211,-35.0221601717607)) ;
#71174=CARTESIAN_POINT('Origin',(201.184777625407,599.847556589211,-35.2721601717607)) ;
#71175=CARTESIAN_POINT('',(201.184777625407,614.670681589221,-35.0221601717607)) ;
#71176=CARTESIAN_POINT('Origin',(201.559777625407,599.847556589211,-35.2721601717609)) ;
#71177=CARTESIAN_POINT('Origin',(201.559777625407,599.847556589211,-35.0221601717607)) ;
#71178=CARTESIAN_POINT('Origin',(201.559777625407,599.847556589211,-35.2721601717609)) ;
#71179=CARTESIAN_POINT('Origin',(202.262277625418,596.097556589211,-35.8624540214915)) ;
#71180=CARTESIAN_POINT('',(202.387277625418,596.097556589211,-39.2297700580612)) ;
#71181=CARTESIAN_POINT('',(202.387277625418,596.097556589211,-35.8624540214915)) ;
#71182=CARTESIAN_POINT('',(202.262277625418,595.972556589211,-39.2297700580612)) ;
#71183=CARTESIAN_POINT('Origin',(202.262277625418,596.097556589211,-39.2297700580612)) ;
#71184=CARTESIAN_POINT('',(202.262277625418,595.972556589211,-35.8624540214915)) ;
#71185=CARTESIAN_POINT('Origin',(202.387277625418,593.368806589211,-33.7667690928544)) ;
#71186=CARTESIAN_POINT('',(202.387277625418,597.462556589212,-39.4182700580611)) ;
#71187=CARTESIAN_POINT('',(202.387277625418,597.462556589212,-37.6444650424525)) ;
#71188=CARTESIAN_POINT('',(202.387277625418,597.274056589212,-39.2297700580612)) ;
#71189=CARTESIAN_POINT('Origin',(202.387277625418,597.274056589212,-39.4182700580611)) ;
#71190=CARTESIAN_POINT('',(202.387277625418,595.988181589211,-39.2297700580612)) ;
#71191=CARTESIAN_POINT('',(202.387277625418,599.847556589211,-39.2297700580612)) ;
#71192=CARTESIAN_POINT('',(202.387277625418,599.847556589211,-33.8937690928544)) ;
#71193=CARTESIAN_POINT('',(202.387277625418,598.671056589212,-39.2297700580612)) ;
#71194=CARTESIAN_POINT('',(202.387277625418,595.988181589211,-39.2297700580612)) ;
#71195=CARTESIAN_POINT('',(202.387277625418,598.482556589212,-39.4182700580611)) ;
#71196=CARTESIAN_POINT('Origin',(202.387277625418,598.671056589212,-39.4182700580612)) ;
#71197=CARTESIAN_POINT('',(202.387277625418,598.482556589212,-39.8669650424525)) ;
#71198=CARTESIAN_POINT('Origin',(202.262277625418,599.847556589211,-33.8937690928544)) ;
#71199=CARTESIAN_POINT('',(202.262277625418,599.972556589211,-39.2297700580612)) ;
#71200=CARTESIAN_POINT('',(202.262277625418,599.972556589211,-33.8937690928544)) ;
#71201=CARTESIAN_POINT('Origin',(202.262277625418,599.847556589211,-39.2297700580612)) ;
#71202=CARTESIAN_POINT('Origin',(197.307277625418,599.972556589211,-34.0207690928544)) ;
#71203=CARTESIAN_POINT('',(201.559777625419,599.972556589211,-39.2297700580612)) ;
#71204=CARTESIAN_POINT('',(201.559777625419,599.972556589211,-38.5610190928544)) ;
#71205=CARTESIAN_POINT('',(207.753027625418,599.972556589211,-39.2297700580612)) ;
#71206=CARTESIAN_POINT('Origin',(201.57290262541,590.722556589211,-35.2721601717607)) ;
#71207=CARTESIAN_POINT('',(201.559777625407,590.722556589211,-35.0221601717607)) ;
#71208=CARTESIAN_POINT('',(201.559777625407,590.472556589211,-35.2721601717607)) ;
#71209=CARTESIAN_POINT('Origin',(201.559777625407,590.722556589211,-35.2721601717607)) ;
#71210=CARTESIAN_POINT('',(202.262277625407,590.472556589211,-35.2721601717608)) ;
#71211=CARTESIAN_POINT('',(201.57290262541,590.472556589211,-35.2721601717607)) ;
#71212=CARTESIAN_POINT('',(202.262277625407,590.722556589211,-35.0221601717608)) ;
#71213=CARTESIAN_POINT('Origin',(202.262277625407,590.722556589211,-35.2721601717608)) ;
#71214=CARTESIAN_POINT('',(201.57290262541,590.722556589211,-35.0221601717607)) ;
#71215=CARTESIAN_POINT('Origin',(202.262277625407,590.347556589211,-35.2721601717609)) ;
#71216=CARTESIAN_POINT('',(202.387277625407,590.347556589211,-35.2721601717609)) ;
#71217=CARTESIAN_POINT('',(202.637277625407,590.347556589211,-35.0221601717608)) ;
#71218=CARTESIAN_POINT('Origin',(202.637277625407,590.347556589211,-35.2721601717609)) ;
#71219=CARTESIAN_POINT('Origin',(202.262277625407,590.347556589211,-35.0221601717608)) ;
#71220=CARTESIAN_POINT('Origin',(202.262277625407,590.347556589211,-35.2721601717609)) ;
#71221=CARTESIAN_POINT('Origin',(202.637277625407,605.170681589221,-35.2721601717608)) ;
#71222=CARTESIAN_POINT('',(202.387277625407,586.597556589211,-35.2721601717608)) ;
#71223=CARTESIAN_POINT('',(202.637277625407,586.597556589211,-35.0221601717608)) ;
#71224=CARTESIAN_POINT('Origin',(202.637277625407,586.597556589211,-35.2721601717608)) ;
#71225=CARTESIAN_POINT('',(202.637277625407,605.170681589221,-35.0221601717608)) ;
#71226=CARTESIAN_POINT('',(202.387277625417,605.170681589221,-35.2721601717608)) ;
#71227=CARTESIAN_POINT('Origin',(202.262277625407,586.597556589211,-35.2721601717609)) ;
#71228=CARTESIAN_POINT('',(202.262277625407,586.472556589211,-35.2721601717609)) ;
#71229=CARTESIAN_POINT('',(202.262277625407,586.222556589211,-35.0221601717608)) ;
#71230=CARTESIAN_POINT('Origin',(202.262277625407,586.222556589211,-35.2721601717609)) ;
#71231=CARTESIAN_POINT('Origin',(202.262277625407,586.597556589211,-35.0221601717608)) ;
#71232=CARTESIAN_POINT('Origin',(202.262277625407,586.597556589211,-35.2721601717609)) ;
#71233=CARTESIAN_POINT('Origin',(205.938476772278,586.222556589211,-35.2721601717609)) ;
#71234=CARTESIAN_POINT('',(201.559777625407,586.472556589211,-35.2721601717607)) ;
#71235=CARTESIAN_POINT('',(201.559777625407,586.222556589211,-35.0221601717607)) ;
#71236=CARTESIAN_POINT('Origin',(201.559777625407,586.222556589211,-35.2721601717607)) ;
#71237=CARTESIAN_POINT('',(205.938476772278,586.222556589211,-35.0221601717609)) ;
#71238=CARTESIAN_POINT('',(205.938476772278,586.472556589211,-35.2721601717609)) ;
#71239=CARTESIAN_POINT('Origin',(201.559777625407,586.597556589211,-35.2721601717609)) ;
#71240=CARTESIAN_POINT('',(201.184777625407,586.597556589211,-35.0221601717607)) ;
#71241=CARTESIAN_POINT('Origin',(201.184777625407,586.597556589211,-35.2721601717609)) ;
#71242=CARTESIAN_POINT('Origin',(201.559777625407,586.597556589211,-35.0221601717607)) ;
#71243=CARTESIAN_POINT('Origin',(201.559777625407,586.597556589211,-35.2721601717609)) ;
#71244=CARTESIAN_POINT('Origin',(201.184777625407,605.170681589221,-35.2721601717607)) ;
#71245=CARTESIAN_POINT('',(201.184777625407,590.347556589211,-35.0221601717607)) ;
#71246=CARTESIAN_POINT('Origin',(201.184777625407,590.347556589211,-35.2721601717607)) ;
#71247=CARTESIAN_POINT('',(201.184777625407,605.170681589221,-35.0221601717607)) ;
#71248=CARTESIAN_POINT('Origin',(201.559777625407,590.347556589211,-35.2721601717609)) ;
#71249=CARTESIAN_POINT('Origin',(201.559777625407,590.347556589211,-35.0221601717607)) ;
#71250=CARTESIAN_POINT('Origin',(201.559777625407,590.347556589211,-35.2721601717609)) ;
#71251=CARTESIAN_POINT('Origin',(202.262277625417,586.597556589211,-35.8624540214915)) ;
#71252=CARTESIAN_POINT('',(202.387277625417,586.597556589211,-39.2297700580612)) ;
#71253=CARTESIAN_POINT('',(202.387277625417,586.597556589211,-35.8624540214915)) ;
#71254=CARTESIAN_POINT('',(202.262277625417,586.472556589211,-39.2297700580612)) ;
#71255=CARTESIAN_POINT('Origin',(202.262277625417,586.597556589211,-39.2297700580612)) ;
#71256=CARTESIAN_POINT('',(202.262277625417,586.472556589211,-35.8624540214915)) ;
#71257=CARTESIAN_POINT('Origin',(202.387277625417,583.868806589211,-33.7667690928544)) ;
#71258=CARTESIAN_POINT('',(202.387277625417,587.962556589212,-39.4182700580611)) ;
#71259=CARTESIAN_POINT('',(202.387277625417,587.962556589212,-37.6444650424525)) ;
#71260=CARTESIAN_POINT('',(202.387277625417,587.774056589212,-39.2297700580612)) ;
#71261=CARTESIAN_POINT('Origin',(202.387277625417,587.774056589212,-39.4182700580611)) ;
#71262=CARTESIAN_POINT('',(202.387277625417,586.488181589211,-39.2297700580612)) ;
#71263=CARTESIAN_POINT('',(202.387277625417,590.347556589211,-39.2297700580612)) ;
#71264=CARTESIAN_POINT('',(202.387277625417,590.347556589211,-33.8937690928544)) ;
#71265=CARTESIAN_POINT('',(202.387277625417,589.171056589212,-39.2297700580612)) ;
#71266=CARTESIAN_POINT('',(202.387277625417,586.488181589211,-39.2297700580612)) ;
#71267=CARTESIAN_POINT('',(202.387277625417,588.982556589212,-39.4182700580611)) ;
#71268=CARTESIAN_POINT('Origin',(202.387277625417,589.171056589212,-39.4182700580612)) ;
#71269=CARTESIAN_POINT('',(202.387277625417,588.982556589212,-39.8669650424525)) ;
#71270=CARTESIAN_POINT('Origin',(202.262277625417,590.347556589211,-33.8937690928544)) ;
#71271=CARTESIAN_POINT('',(202.262277625417,590.472556589211,-39.2297700580612)) ;
#71272=CARTESIAN_POINT('',(202.262277625417,590.472556589211,-33.8937690928544)) ;
#71273=CARTESIAN_POINT('Origin',(202.262277625417,590.347556589211,-39.2297700580612)) ;
#71274=CARTESIAN_POINT('Origin',(197.307277625417,590.472556589211,-34.0207690928544)) ;
#71275=CARTESIAN_POINT('',(201.559777625417,590.472556589211,-39.2297700580612)) ;
#71276=CARTESIAN_POINT('',(201.559777625417,590.472556589211,-38.5610190928544)) ;
#71277=CARTESIAN_POINT('',(207.753027625417,590.472556589211,-39.2297700580612)) ;
#71278=CARTESIAN_POINT('Origin',(201.57290262541,581.222556589211,-35.2721601717607)) ;
#71279=CARTESIAN_POINT('',(201.559777625407,581.222556589211,-35.0221601717607)) ;
#71280=CARTESIAN_POINT('',(201.559777625407,580.972556589211,-35.2721601717607)) ;
#71281=CARTESIAN_POINT('Origin',(201.559777625407,581.222556589211,-35.2721601717607)) ;
#71282=CARTESIAN_POINT('',(202.262277625407,580.972556589211,-35.2721601717608)) ;
#71283=CARTESIAN_POINT('',(201.57290262541,580.972556589211,-35.2721601717607)) ;
#71284=CARTESIAN_POINT('',(202.262277625407,581.222556589211,-35.0221601717608)) ;
#71285=CARTESIAN_POINT('Origin',(202.262277625407,581.222556589211,-35.2721601717608)) ;
#71286=CARTESIAN_POINT('',(201.57290262541,581.222556589211,-35.0221601717607)) ;
#71287=CARTESIAN_POINT('Origin',(202.262277625407,580.847556589211,-35.2721601717609)) ;
#71288=CARTESIAN_POINT('',(202.387277625407,580.847556589211,-35.2721601717609)) ;
#71289=CARTESIAN_POINT('',(202.637277625407,580.847556589211,-35.0221601717608)) ;
#71290=CARTESIAN_POINT('Origin',(202.637277625407,580.847556589211,-35.2721601717609)) ;
#71291=CARTESIAN_POINT('Origin',(202.262277625407,580.847556589211,-35.0221601717608)) ;
#71292=CARTESIAN_POINT('Origin',(202.262277625407,580.847556589211,-35.2721601717609)) ;
#71293=CARTESIAN_POINT('Origin',(202.637277625407,595.670681589221,-35.2721601717608)) ;
#71294=CARTESIAN_POINT('',(202.387277625407,577.097556589211,-35.2721601717608)) ;
#71295=CARTESIAN_POINT('',(202.637277625407,577.097556589211,-35.0221601717608)) ;
#71296=CARTESIAN_POINT('Origin',(202.637277625407,577.097556589211,-35.2721601717608)) ;
#71297=CARTESIAN_POINT('',(202.637277625407,595.670681589221,-35.0221601717608)) ;
#71298=CARTESIAN_POINT('',(202.387277625415,595.670681589221,-35.2721601717608)) ;
#71299=CARTESIAN_POINT('Origin',(202.262277625407,577.097556589211,-35.2721601717609)) ;
#71300=CARTESIAN_POINT('',(202.262277625407,576.972556589211,-35.2721601717609)) ;
#71301=CARTESIAN_POINT('',(202.262277625407,576.722556589211,-35.0221601717608)) ;
#71302=CARTESIAN_POINT('Origin',(202.262277625407,576.722556589211,-35.2721601717609)) ;
#71303=CARTESIAN_POINT('Origin',(202.262277625407,577.097556589211,-35.0221601717608)) ;
#71304=CARTESIAN_POINT('Origin',(202.262277625407,577.097556589211,-35.2721601717609)) ;
#71305=CARTESIAN_POINT('Origin',(205.938476772278,576.722556589211,-35.2721601717609)) ;
#71306=CARTESIAN_POINT('',(201.559777625407,576.972556589211,-35.2721601717607)) ;
#71307=CARTESIAN_POINT('',(201.559777625407,576.722556589211,-35.0221601717607)) ;
#71308=CARTESIAN_POINT('Origin',(201.559777625407,576.722556589211,-35.2721601717607)) ;
#71309=CARTESIAN_POINT('',(205.938476772278,576.722556589211,-35.0221601717609)) ;
#71310=CARTESIAN_POINT('',(205.938476772278,576.972556589211,-35.2721601717609)) ;
#71311=CARTESIAN_POINT('Origin',(201.559777625407,577.097556589211,-35.2721601717609)) ;
#71312=CARTESIAN_POINT('',(201.184777625407,577.097556589211,-35.0221601717607)) ;
#71313=CARTESIAN_POINT('Origin',(201.184777625407,577.097556589211,-35.2721601717609)) ;
#71314=CARTESIAN_POINT('Origin',(201.559777625407,577.097556589211,-35.0221601717607)) ;
#71315=CARTESIAN_POINT('Origin',(201.559777625407,577.097556589211,-35.2721601717609)) ;
#71316=CARTESIAN_POINT('Origin',(201.184777625407,595.670681589221,-35.2721601717607)) ;
#71317=CARTESIAN_POINT('',(201.184777625407,580.847556589211,-35.0221601717607)) ;
#71318=CARTESIAN_POINT('Origin',(201.184777625407,580.847556589211,-35.2721601717607)) ;
#71319=CARTESIAN_POINT('',(201.184777625407,595.670681589221,-35.0221601717607)) ;
#71320=CARTESIAN_POINT('Origin',(201.559777625407,580.847556589211,-35.2721601717609)) ;
#71321=CARTESIAN_POINT('Origin',(201.559777625407,580.847556589211,-35.0221601717607)) ;
#71322=CARTESIAN_POINT('Origin',(201.559777625407,580.847556589211,-35.2721601717609)) ;
#71323=CARTESIAN_POINT('Origin',(202.262277625415,577.097556589211,-35.8624540214915)) ;
#71324=CARTESIAN_POINT('',(202.387277625415,577.097556589211,-39.2297700580612)) ;
#71325=CARTESIAN_POINT('',(202.387277625415,577.097556589211,-35.8624540214915)) ;
#71326=CARTESIAN_POINT('',(202.262277625415,576.972556589211,-39.2297700580612)) ;
#71327=CARTESIAN_POINT('Origin',(202.262277625415,577.097556589211,-39.2297700580612)) ;
#71328=CARTESIAN_POINT('',(202.262277625415,576.972556589211,-35.8624540214915)) ;
#71329=CARTESIAN_POINT('Origin',(202.387277625415,574.368806589211,-33.7667690928544)) ;
#71330=CARTESIAN_POINT('',(202.387277625415,578.462556589212,-39.4182700580611)) ;
#71331=CARTESIAN_POINT('',(202.387277625415,578.462556589212,-37.6444650424525)) ;
#71332=CARTESIAN_POINT('',(202.387277625415,578.274056589212,-39.2297700580612)) ;
#71333=CARTESIAN_POINT('Origin',(202.387277625415,578.274056589212,-39.4182700580611)) ;
#71334=CARTESIAN_POINT('',(202.387277625415,576.988181589211,-39.2297700580612)) ;
#71335=CARTESIAN_POINT('',(202.387277625415,580.847556589211,-39.2297700580612)) ;
#71336=CARTESIAN_POINT('',(202.387277625415,580.847556589211,-33.8937690928544)) ;
#71337=CARTESIAN_POINT('',(202.387277625415,579.671056589212,-39.2297700580612)) ;
#71338=CARTESIAN_POINT('',(202.387277625415,576.988181589211,-39.2297700580612)) ;
#71339=CARTESIAN_POINT('',(202.387277625415,579.482556589212,-39.4182700580611)) ;
#71340=CARTESIAN_POINT('Origin',(202.387277625415,579.671056589212,-39.4182700580612)) ;
#71341=CARTESIAN_POINT('',(202.387277625415,579.482556589212,-39.8669650424525)) ;
#71342=CARTESIAN_POINT('Origin',(202.262277625415,580.847556589211,-33.8937690928544)) ;
#71343=CARTESIAN_POINT('',(202.262277625415,580.972556589211,-39.2297700580612)) ;
#71344=CARTESIAN_POINT('',(202.262277625415,580.972556589211,-33.8937690928544)) ;
#71345=CARTESIAN_POINT('Origin',(202.262277625415,580.847556589211,-39.2297700580612)) ;
#71346=CARTESIAN_POINT('Origin',(197.307277625415,580.972556589211,-34.0207690928544)) ;
#71347=CARTESIAN_POINT('',(201.559777625415,580.972556589211,-39.2297700580612)) ;
#71348=CARTESIAN_POINT('',(201.559777625415,580.972556589211,-38.5610190928544)) ;
#71349=CARTESIAN_POINT('',(207.753027625415,580.972556589211,-39.2297700580612)) ;
#71350=CARTESIAN_POINT('Origin',(201.57290262541,571.722556589211,-35.2721601717607)) ;
#71351=CARTESIAN_POINT('',(201.559777625407,571.722556589211,-35.0221601717607)) ;
#71352=CARTESIAN_POINT('',(201.559777625407,571.472556589211,-35.2721601717607)) ;
#71353=CARTESIAN_POINT('Origin',(201.559777625407,571.722556589211,-35.2721601717607)) ;
#71354=CARTESIAN_POINT('',(202.262277625407,571.472556589211,-35.2721601717608)) ;
#71355=CARTESIAN_POINT('',(201.57290262541,571.472556589211,-35.2721601717607)) ;
#71356=CARTESIAN_POINT('',(202.262277625407,571.722556589211,-35.0221601717608)) ;
#71357=CARTESIAN_POINT('Origin',(202.262277625407,571.722556589211,-35.2721601717608)) ;
#71358=CARTESIAN_POINT('',(201.57290262541,571.722556589211,-35.0221601717607)) ;
#71359=CARTESIAN_POINT('Origin',(202.262277625407,571.347556589211,-35.2721601717609)) ;
#71360=CARTESIAN_POINT('',(202.387277625407,571.347556589211,-35.2721601717609)) ;
#71361=CARTESIAN_POINT('',(202.637277625407,571.347556589211,-35.0221601717608)) ;
#71362=CARTESIAN_POINT('Origin',(202.637277625407,571.347556589211,-35.2721601717609)) ;
#71363=CARTESIAN_POINT('Origin',(202.262277625407,571.347556589211,-35.0221601717608)) ;
#71364=CARTESIAN_POINT('Origin',(202.262277625407,571.347556589211,-35.2721601717609)) ;
#71365=CARTESIAN_POINT('Origin',(202.637277625407,586.170681589221,-35.2721601717608)) ;
#71366=CARTESIAN_POINT('',(202.387277625407,567.59755658921,-35.2721601717608)) ;
#71367=CARTESIAN_POINT('',(202.637277625407,567.59755658921,-35.0221601717608)) ;
#71368=CARTESIAN_POINT('Origin',(202.637277625407,567.59755658921,-35.2721601717608)) ;
#71369=CARTESIAN_POINT('',(202.637277625407,586.170681589221,-35.0221601717608)) ;
#71370=CARTESIAN_POINT('',(202.387277625413,586.170681589221,-35.2721601717608)) ;
#71371=CARTESIAN_POINT('Origin',(202.262277625407,567.59755658921,-35.2721601717609)) ;
#71372=CARTESIAN_POINT('',(202.262277625407,567.472556589211,-35.2721601717609)) ;
#71373=CARTESIAN_POINT('',(202.262277625407,567.222556589211,-35.0221601717608)) ;
#71374=CARTESIAN_POINT('Origin',(202.262277625407,567.222556589211,-35.2721601717609)) ;
#71375=CARTESIAN_POINT('Origin',(202.262277625407,567.59755658921,-35.0221601717608)) ;
#71376=CARTESIAN_POINT('Origin',(202.262277625407,567.59755658921,-35.2721601717609)) ;
#71377=CARTESIAN_POINT('Origin',(205.938476772278,567.222556589211,-35.2721601717609)) ;
#71378=CARTESIAN_POINT('',(201.559777625407,567.472556589211,-35.2721601717607)) ;
#71379=CARTESIAN_POINT('',(201.559777625407,567.222556589211,-35.0221601717607)) ;
#71380=CARTESIAN_POINT('Origin',(201.559777625407,567.222556589211,-35.2721601717607)) ;
#71381=CARTESIAN_POINT('',(205.938476772278,567.222556589211,-35.0221601717609)) ;
#71382=CARTESIAN_POINT('',(205.938476772278,567.47255658921,-35.2721601717609)) ;
#71383=CARTESIAN_POINT('Origin',(201.559777625407,567.597556589211,-35.2721601717609)) ;
#71384=CARTESIAN_POINT('',(201.184777625407,567.597556589211,-35.0221601717607)) ;
#71385=CARTESIAN_POINT('Origin',(201.184777625407,567.597556589211,-35.2721601717609)) ;
#71386=CARTESIAN_POINT('Origin',(201.559777625407,567.597556589211,-35.0221601717607)) ;
#71387=CARTESIAN_POINT('Origin',(201.559777625407,567.597556589211,-35.2721601717609)) ;
#71388=CARTESIAN_POINT('Origin',(201.184777625407,586.170681589221,-35.2721601717607)) ;
#71389=CARTESIAN_POINT('',(201.184777625407,571.347556589211,-35.0221601717607)) ;
#71390=CARTESIAN_POINT('Origin',(201.184777625407,571.347556589211,-35.2721601717607)) ;
#71391=CARTESIAN_POINT('',(201.184777625407,586.170681589221,-35.0221601717607)) ;
#71392=CARTESIAN_POINT('Origin',(201.559777625407,571.347556589211,-35.2721601717609)) ;
#71393=CARTESIAN_POINT('Origin',(201.559777625407,571.347556589211,-35.0221601717607)) ;
#71394=CARTESIAN_POINT('Origin',(201.559777625407,571.347556589211,-35.2721601717609)) ;
#71395=CARTESIAN_POINT('Origin',(202.262277625413,567.59755658921,-35.8624540214915)) ;
#71396=CARTESIAN_POINT('',(202.387277625413,567.59755658921,-39.2297700580612)) ;
#71397=CARTESIAN_POINT('',(202.387277625413,567.59755658921,-35.8624540214915)) ;
#71398=CARTESIAN_POINT('',(202.262277625413,567.47255658921,-39.2297700580612)) ;
#71399=CARTESIAN_POINT('Origin',(202.262277625413,567.59755658921,-39.2297700580612)) ;
#71400=CARTESIAN_POINT('',(202.262277625413,567.47255658921,-35.8624540214915)) ;
#71401=CARTESIAN_POINT('Origin',(202.387277625413,564.868806589211,-33.7667690928544)) ;
#71402=CARTESIAN_POINT('',(202.387277625413,568.962556589212,-39.4182700580611)) ;
#71403=CARTESIAN_POINT('',(202.387277625413,568.962556589212,-37.6444650424525)) ;
#71404=CARTESIAN_POINT('',(202.387277625413,568.774056589212,-39.2297700580612)) ;
#71405=CARTESIAN_POINT('Origin',(202.387277625413,568.774056589212,-39.4182700580611)) ;
#71406=CARTESIAN_POINT('',(202.387277625413,567.488181589211,-39.2297700580612)) ;
#71407=CARTESIAN_POINT('',(202.387277625413,571.347556589211,-39.2297700580612)) ;
#71408=CARTESIAN_POINT('',(202.387277625413,571.347556589211,-33.8937690928544)) ;
#71409=CARTESIAN_POINT('',(202.387277625413,570.171056589212,-39.2297700580612)) ;
#71410=CARTESIAN_POINT('',(202.387277625413,567.488181589211,-39.2297700580612)) ;
#71411=CARTESIAN_POINT('',(202.387277625413,569.982556589212,-39.4182700580611)) ;
#71412=CARTESIAN_POINT('Origin',(202.387277625413,570.171056589212,-39.4182700580612)) ;
#71413=CARTESIAN_POINT('',(202.387277625413,569.982556589212,-39.8669650424525)) ;
#71414=CARTESIAN_POINT('Origin',(202.262277625413,571.347556589211,-33.8937690928544)) ;
#71415=CARTESIAN_POINT('',(202.262277625413,571.472556589211,-39.2297700580612)) ;
#71416=CARTESIAN_POINT('',(202.262277625413,571.472556589211,-33.8937690928544)) ;
#71417=CARTESIAN_POINT('Origin',(202.262277625413,571.347556589211,-39.2297700580612)) ;
#71418=CARTESIAN_POINT('Origin',(197.307277625413,571.472556589211,-34.0207690928544)) ;
#71419=CARTESIAN_POINT('',(201.559777625414,571.472556589211,-39.2297700580612)) ;
#71420=CARTESIAN_POINT('',(201.559777625414,571.472556589211,-38.5610190928544)) ;
#71421=CARTESIAN_POINT('',(207.753027625413,571.472556589211,-39.2297700580612)) ;
#71422=CARTESIAN_POINT('Origin',(201.57290262541,562.222556589211,-35.2721601717607)) ;
#71423=CARTESIAN_POINT('',(201.559777625407,562.222556589211,-35.0221601717607)) ;
#71424=CARTESIAN_POINT('',(201.559777625407,561.972556589211,-35.2721601717607)) ;
#71425=CARTESIAN_POINT('Origin',(201.559777625407,562.222556589211,-35.2721601717607)) ;
#71426=CARTESIAN_POINT('',(202.262277625407,561.972556589211,-35.2721601717608)) ;
#71427=CARTESIAN_POINT('',(201.57290262541,561.972556589211,-35.2721601717607)) ;
#71428=CARTESIAN_POINT('',(202.262277625407,562.222556589211,-35.0221601717608)) ;
#71429=CARTESIAN_POINT('Origin',(202.262277625407,562.222556589211,-35.2721601717608)) ;
#71430=CARTESIAN_POINT('',(201.57290262541,562.222556589211,-35.0221601717607)) ;
#71431=CARTESIAN_POINT('Origin',(202.262277625407,561.847556589211,-35.2721601717609)) ;
#71432=CARTESIAN_POINT('',(202.387277625407,561.847556589211,-35.2721601717609)) ;
#71433=CARTESIAN_POINT('',(202.637277625407,561.847556589211,-35.0221601717608)) ;
#71434=CARTESIAN_POINT('Origin',(202.637277625407,561.847556589211,-35.2721601717609)) ;
#71435=CARTESIAN_POINT('Origin',(202.262277625407,561.847556589211,-35.0221601717608)) ;
#71436=CARTESIAN_POINT('Origin',(202.262277625407,561.847556589211,-35.2721601717609)) ;
#71437=CARTESIAN_POINT('Origin',(202.637277625407,576.670681589221,-35.2721601717608)) ;
#71438=CARTESIAN_POINT('',(202.387277625407,558.09755658921,-35.2721601717608)) ;
#71439=CARTESIAN_POINT('',(202.637277625407,558.09755658921,-35.0221601717608)) ;
#71440=CARTESIAN_POINT('Origin',(202.637277625407,558.09755658921,-35.2721601717608)) ;
#71441=CARTESIAN_POINT('',(202.637277625407,576.670681589221,-35.0221601717608)) ;
#71442=CARTESIAN_POINT('',(202.387277625412,576.670681589221,-35.2721601717608)) ;
#71443=CARTESIAN_POINT('Origin',(202.262277625407,558.09755658921,-35.2721601717609)) ;
#71444=CARTESIAN_POINT('',(202.262277625407,557.97255658921,-35.2721601717609)) ;
#71445=CARTESIAN_POINT('',(202.262277625407,557.722556589211,-35.0221601717608)) ;
#71446=CARTESIAN_POINT('Origin',(202.262277625407,557.722556589211,-35.2721601717609)) ;
#71447=CARTESIAN_POINT('Origin',(202.262277625407,558.09755658921,-35.0221601717608)) ;
#71448=CARTESIAN_POINT('Origin',(202.262277625407,558.09755658921,-35.2721601717609)) ;
#71449=CARTESIAN_POINT('Origin',(205.938476772278,557.722556589211,-35.2721601717609)) ;
#71450=CARTESIAN_POINT('',(201.559777625407,557.97255658921,-35.2721601717607)) ;
#71451=CARTESIAN_POINT('',(201.559777625407,557.722556589211,-35.0221601717607)) ;
#71452=CARTESIAN_POINT('Origin',(201.559777625407,557.722556589211,-35.2721601717607)) ;
#71453=CARTESIAN_POINT('',(205.938476772278,557.722556589211,-35.0221601717609)) ;
#71454=CARTESIAN_POINT('',(205.938476772278,557.97255658921,-35.2721601717609)) ;
#71455=CARTESIAN_POINT('Origin',(201.559777625407,558.097556589211,-35.2721601717609)) ;
#71456=CARTESIAN_POINT('',(201.184777625407,558.097556589211,-35.0221601717607)) ;
#71457=CARTESIAN_POINT('Origin',(201.184777625407,558.097556589211,-35.2721601717609)) ;
#71458=CARTESIAN_POINT('Origin',(201.559777625407,558.097556589211,-35.0221601717607)) ;
#71459=CARTESIAN_POINT('Origin',(201.559777625407,558.097556589211,-35.2721601717609)) ;
#71460=CARTESIAN_POINT('Origin',(201.184777625407,576.670681589221,-35.2721601717607)) ;
#71461=CARTESIAN_POINT('',(201.184777625407,561.847556589211,-35.0221601717607)) ;
#71462=CARTESIAN_POINT('Origin',(201.184777625407,561.847556589211,-35.2721601717607)) ;
#71463=CARTESIAN_POINT('',(201.184777625407,576.670681589221,-35.0221601717607)) ;
#71464=CARTESIAN_POINT('Origin',(201.559777625407,561.847556589211,-35.2721601717609)) ;
#71465=CARTESIAN_POINT('Origin',(201.559777625407,561.847556589211,-35.0221601717607)) ;
#71466=CARTESIAN_POINT('Origin',(201.559777625407,561.847556589211,-35.2721601717609)) ;
#71467=CARTESIAN_POINT('Origin',(202.262277625412,558.09755658921,-35.8624540214915)) ;
#71468=CARTESIAN_POINT('',(202.387277625412,558.09755658921,-39.2297700580612)) ;
#71469=CARTESIAN_POINT('',(202.387277625412,558.09755658921,-35.8624540214915)) ;
#71470=CARTESIAN_POINT('',(202.262277625412,557.97255658921,-39.2297700580612)) ;
#71471=CARTESIAN_POINT('Origin',(202.262277625412,558.09755658921,-39.2297700580612)) ;
#71472=CARTESIAN_POINT('',(202.262277625412,557.97255658921,-35.8624540214915)) ;
#71473=CARTESIAN_POINT('Origin',(202.387277625412,555.368806589211,-33.7667690928544)) ;
#71474=CARTESIAN_POINT('',(202.387277625412,559.462556589212,-39.4182700580611)) ;
#71475=CARTESIAN_POINT('',(202.387277625412,559.462556589212,-37.6444650424525)) ;
#71476=CARTESIAN_POINT('',(202.387277625412,559.274056589212,-39.2297700580612)) ;
#71477=CARTESIAN_POINT('Origin',(202.387277625412,559.274056589212,-39.4182700580611)) ;
#71478=CARTESIAN_POINT('',(202.387277625412,557.988181589211,-39.2297700580612)) ;
#71479=CARTESIAN_POINT('',(202.387277625412,561.847556589211,-39.2297700580612)) ;
#71480=CARTESIAN_POINT('',(202.387277625412,561.847556589211,-33.8937690928544)) ;
#71481=CARTESIAN_POINT('',(202.387277625412,560.671056589212,-39.2297700580612)) ;
#71482=CARTESIAN_POINT('',(202.387277625412,557.988181589211,-39.2297700580612)) ;
#71483=CARTESIAN_POINT('',(202.387277625412,560.482556589212,-39.4182700580611)) ;
#71484=CARTESIAN_POINT('Origin',(202.387277625412,560.671056589212,-39.4182700580612)) ;
#71485=CARTESIAN_POINT('',(202.387277625412,560.482556589212,-39.8669650424525)) ;
#71486=CARTESIAN_POINT('Origin',(202.262277625412,561.847556589211,-33.8937690928544)) ;
#71487=CARTESIAN_POINT('',(202.262277625412,561.972556589211,-39.2297700580612)) ;
#71488=CARTESIAN_POINT('',(202.262277625412,561.972556589211,-33.8937690928544)) ;
#71489=CARTESIAN_POINT('Origin',(202.262277625412,561.847556589211,-39.2297700580612)) ;
#71490=CARTESIAN_POINT('Origin',(197.307277625412,561.972556589211,-34.0207690928544)) ;
#71491=CARTESIAN_POINT('',(201.559777625412,561.972556589211,-39.2297700580612)) ;
#71492=CARTESIAN_POINT('',(201.559777625412,561.972556589211,-38.5610190928544)) ;
#71493=CARTESIAN_POINT('',(207.753027625412,561.972556589211,-39.2297700580612)) ;
#71494=CARTESIAN_POINT('Origin',(201.57290262541,552.722556589211,-35.2721601717607)) ;
#71495=CARTESIAN_POINT('',(201.559777625407,552.722556589211,-35.0221601717607)) ;
#71496=CARTESIAN_POINT('',(201.559777625407,552.472556589211,-35.2721601717607)) ;
#71497=CARTESIAN_POINT('Origin',(201.559777625407,552.722556589211,-35.2721601717607)) ;
#71498=CARTESIAN_POINT('',(202.262277625407,552.472556589211,-35.2721601717608)) ;
#71499=CARTESIAN_POINT('',(201.57290262541,552.472556589211,-35.2721601717607)) ;
#71500=CARTESIAN_POINT('',(202.262277625407,552.722556589211,-35.0221601717608)) ;
#71501=CARTESIAN_POINT('Origin',(202.262277625407,552.722556589211,-35.2721601717608)) ;
#71502=CARTESIAN_POINT('',(201.57290262541,552.722556589211,-35.0221601717607)) ;
#71503=CARTESIAN_POINT('Origin',(202.262277625407,552.347556589211,-35.2721601717609)) ;
#71504=CARTESIAN_POINT('',(202.387277625407,552.347556589211,-35.2721601717609)) ;
#71505=CARTESIAN_POINT('',(202.637277625407,552.347556589211,-35.0221601717608)) ;
#71506=CARTESIAN_POINT('Origin',(202.637277625407,552.347556589211,-35.2721601717609)) ;
#71507=CARTESIAN_POINT('Origin',(202.262277625407,552.347556589211,-35.0221601717608)) ;
#71508=CARTESIAN_POINT('Origin',(202.262277625407,552.347556589211,-35.2721601717609)) ;
#71509=CARTESIAN_POINT('Origin',(202.637277625407,567.170681589221,-35.2721601717608)) ;
#71510=CARTESIAN_POINT('',(202.387277625407,548.59755658921,-35.2721601717608)) ;
#71511=CARTESIAN_POINT('',(202.637277625407,548.59755658921,-35.0221601717608)) ;
#71512=CARTESIAN_POINT('Origin',(202.637277625407,548.59755658921,-35.2721601717608)) ;
#71513=CARTESIAN_POINT('',(202.637277625407,567.170681589221,-35.0221601717608)) ;
#71514=CARTESIAN_POINT('',(202.38727762541,567.170681589221,-35.2721601717608)) ;
#71515=CARTESIAN_POINT('Origin',(202.262277625407,548.59755658921,-35.2721601717609)) ;
#71516=CARTESIAN_POINT('',(202.262277625407,548.47255658921,-35.2721601717609)) ;
#71517=CARTESIAN_POINT('',(202.262277625407,548.22255658921,-35.0221601717608)) ;
#71518=CARTESIAN_POINT('Origin',(202.262277625407,548.22255658921,-35.2721601717609)) ;
#71519=CARTESIAN_POINT('Origin',(202.262277625407,548.59755658921,-35.0221601717608)) ;
#71520=CARTESIAN_POINT('Origin',(202.262277625407,548.59755658921,-35.2721601717609)) ;
#71521=CARTESIAN_POINT('Origin',(205.938476772278,548.22255658921,-35.2721601717609)) ;
#71522=CARTESIAN_POINT('',(201.559777625407,548.47255658921,-35.2721601717607)) ;
#71523=CARTESIAN_POINT('',(201.559777625407,548.22255658921,-35.0221601717607)) ;
#71524=CARTESIAN_POINT('Origin',(201.559777625407,548.22255658921,-35.2721601717607)) ;
#71525=CARTESIAN_POINT('',(205.938476772278,548.22255658921,-35.0221601717609)) ;
#71526=CARTESIAN_POINT('',(205.938476772278,548.47255658921,-35.2721601717609)) ;
#71527=CARTESIAN_POINT('Origin',(201.559777625407,548.59755658921,-35.2721601717609)) ;
#71528=CARTESIAN_POINT('',(201.184777625407,548.59755658921,-35.0221601717607)) ;
#71529=CARTESIAN_POINT('Origin',(201.184777625407,548.59755658921,-35.2721601717609)) ;
#71530=CARTESIAN_POINT('Origin',(201.559777625407,548.59755658921,-35.0221601717607)) ;
#71531=CARTESIAN_POINT('Origin',(201.559777625407,548.59755658921,-35.2721601717609)) ;
#71532=CARTESIAN_POINT('Origin',(201.184777625407,567.170681589221,-35.2721601717607)) ;
#71533=CARTESIAN_POINT('',(201.184777625407,552.347556589211,-35.0221601717607)) ;
#71534=CARTESIAN_POINT('Origin',(201.184777625407,552.347556589211,-35.2721601717607)) ;
#71535=CARTESIAN_POINT('',(201.184777625407,567.170681589221,-35.0221601717607)) ;
#71536=CARTESIAN_POINT('Origin',(201.559777625407,552.347556589211,-35.2721601717609)) ;
#71537=CARTESIAN_POINT('Origin',(201.559777625407,552.347556589211,-35.0221601717607)) ;
#71538=CARTESIAN_POINT('Origin',(201.559777625407,552.347556589211,-35.2721601717609)) ;
#71539=CARTESIAN_POINT('Origin',(202.26227762541,548.59755658921,-35.8624540214915)) ;
#71540=CARTESIAN_POINT('',(202.38727762541,548.59755658921,-39.2297700580612)) ;
#71541=CARTESIAN_POINT('',(202.38727762541,548.59755658921,-35.8624540214915)) ;
#71542=CARTESIAN_POINT('',(202.26227762541,548.47255658921,-39.2297700580612)) ;
#71543=CARTESIAN_POINT('Origin',(202.26227762541,548.59755658921,-39.2297700580612)) ;
#71544=CARTESIAN_POINT('',(202.26227762541,548.47255658921,-35.8624540214915)) ;
#71545=CARTESIAN_POINT('Origin',(202.38727762541,545.868806589211,-33.7667690928544)) ;
#71546=CARTESIAN_POINT('',(202.38727762541,549.962556589212,-39.4182700580611)) ;
#71547=CARTESIAN_POINT('',(202.38727762541,549.962556589212,-37.6444650424525)) ;
#71548=CARTESIAN_POINT('',(202.38727762541,549.774056589212,-39.2297700580612)) ;
#71549=CARTESIAN_POINT('Origin',(202.38727762541,549.774056589212,-39.4182700580611)) ;
#71550=CARTESIAN_POINT('',(202.38727762541,548.488181589211,-39.2297700580612)) ;
#71551=CARTESIAN_POINT('',(202.38727762541,552.347556589211,-39.2297700580612)) ;
#71552=CARTESIAN_POINT('',(202.38727762541,552.347556589211,-33.8937690928544)) ;
#71553=CARTESIAN_POINT('',(202.38727762541,551.171056589212,-39.2297700580612)) ;
#71554=CARTESIAN_POINT('',(202.38727762541,548.488181589211,-39.2297700580612)) ;
#71555=CARTESIAN_POINT('',(202.38727762541,550.982556589212,-39.4182700580611)) ;
#71556=CARTESIAN_POINT('Origin',(202.38727762541,551.171056589212,-39.4182700580612)) ;
#71557=CARTESIAN_POINT('',(202.38727762541,550.982556589212,-39.8669650424525)) ;
#71558=CARTESIAN_POINT('Origin',(202.26227762541,552.347556589211,-33.8937690928544)) ;
#71559=CARTESIAN_POINT('',(202.26227762541,552.472556589211,-39.2297700580612)) ;
#71560=CARTESIAN_POINT('',(202.26227762541,552.472556589211,-33.8937690928544)) ;
#71561=CARTESIAN_POINT('Origin',(202.26227762541,552.347556589211,-39.2297700580612)) ;
#71562=CARTESIAN_POINT('Origin',(197.30727762541,552.472556589211,-34.0207690928544)) ;
#71563=CARTESIAN_POINT('',(201.55977762541,552.472556589211,-39.2297700580612)) ;
#71564=CARTESIAN_POINT('',(201.55977762541,552.472556589211,-38.5610190928544)) ;
#71565=CARTESIAN_POINT('',(207.75302762541,552.472556589211,-39.2297700580612)) ;
#71566=CARTESIAN_POINT('Origin',(201.57290262541,543.222556589211,-35.2721601717607)) ;
#71567=CARTESIAN_POINT('',(201.559777625407,543.222556589211,-35.0221601717607)) ;
#71568=CARTESIAN_POINT('',(201.559777625407,542.972556589211,-35.2721601717607)) ;
#71569=CARTESIAN_POINT('Origin',(201.559777625407,543.222556589211,-35.2721601717607)) ;
#71570=CARTESIAN_POINT('',(202.262277625407,542.972556589211,-35.2721601717608)) ;
#71571=CARTESIAN_POINT('',(201.57290262541,542.972556589211,-35.2721601717607)) ;
#71572=CARTESIAN_POINT('',(202.262277625407,543.222556589211,-35.0221601717608)) ;
#71573=CARTESIAN_POINT('Origin',(202.262277625407,543.222556589211,-35.2721601717608)) ;
#71574=CARTESIAN_POINT('',(201.57290262541,543.222556589211,-35.0221601717607)) ;
#71575=CARTESIAN_POINT('Origin',(202.262277625407,542.847556589211,-35.2721601717609)) ;
#71576=CARTESIAN_POINT('',(202.387277625407,542.847556589211,-35.2721601717609)) ;
#71577=CARTESIAN_POINT('',(202.637277625407,542.847556589211,-35.0221601717608)) ;
#71578=CARTESIAN_POINT('Origin',(202.637277625407,542.847556589211,-35.2721601717609)) ;
#71579=CARTESIAN_POINT('Origin',(202.262277625407,542.847556589211,-35.0221601717608)) ;
#71580=CARTESIAN_POINT('Origin',(202.262277625407,542.847556589211,-35.2721601717609)) ;
#71581=CARTESIAN_POINT('Origin',(202.637277625407,557.670681589221,-35.2721601717608)) ;
#71582=CARTESIAN_POINT('',(202.387277625407,539.09755658921,-35.2721601717608)) ;
#71583=CARTESIAN_POINT('',(202.637277625407,539.09755658921,-35.0221601717608)) ;
#71584=CARTESIAN_POINT('Origin',(202.637277625407,539.09755658921,-35.2721601717608)) ;
#71585=CARTESIAN_POINT('',(202.637277625407,557.670681589221,-35.0221601717608)) ;
#71586=CARTESIAN_POINT('',(202.387277625408,557.670681589221,-35.2721601717608)) ;
#71587=CARTESIAN_POINT('Origin',(202.262277625407,539.09755658921,-35.2721601717609)) ;
#71588=CARTESIAN_POINT('',(202.262277625407,538.97255658921,-35.2721601717609)) ;
#71589=CARTESIAN_POINT('',(202.262277625407,538.72255658921,-35.0221601717608)) ;
#71590=CARTESIAN_POINT('Origin',(202.262277625407,538.72255658921,-35.2721601717609)) ;
#71591=CARTESIAN_POINT('Origin',(202.262277625407,539.09755658921,-35.0221601717608)) ;
#71592=CARTESIAN_POINT('Origin',(202.262277625407,539.09755658921,-35.2721601717609)) ;
#71593=CARTESIAN_POINT('Origin',(205.938476772278,538.72255658921,-35.2721601717609)) ;
#71594=CARTESIAN_POINT('',(201.559777625407,538.97255658921,-35.2721601717607)) ;
#71595=CARTESIAN_POINT('',(201.559777625407,538.72255658921,-35.0221601717607)) ;
#71596=CARTESIAN_POINT('Origin',(201.559777625407,538.72255658921,-35.2721601717607)) ;
#71597=CARTESIAN_POINT('',(205.938476772278,538.72255658921,-35.0221601717609)) ;
#71598=CARTESIAN_POINT('',(205.938476772278,538.97255658921,-35.2721601717609)) ;
#71599=CARTESIAN_POINT('Origin',(201.559777625407,539.09755658921,-35.2721601717609)) ;
#71600=CARTESIAN_POINT('',(201.184777625407,539.09755658921,-35.0221601717607)) ;
#71601=CARTESIAN_POINT('Origin',(201.184777625407,539.09755658921,-35.2721601717609)) ;
#71602=CARTESIAN_POINT('Origin',(201.559777625407,539.09755658921,-35.0221601717607)) ;
#71603=CARTESIAN_POINT('Origin',(201.559777625407,539.09755658921,-35.2721601717609)) ;
#71604=CARTESIAN_POINT('Origin',(201.184777625407,557.670681589221,-35.2721601717607)) ;
#71605=CARTESIAN_POINT('',(201.184777625407,542.847556589211,-35.0221601717607)) ;
#71606=CARTESIAN_POINT('Origin',(201.184777625407,542.847556589211,-35.2721601717607)) ;
#71607=CARTESIAN_POINT('',(201.184777625407,557.670681589221,-35.0221601717607)) ;
#71608=CARTESIAN_POINT('Origin',(201.559777625407,542.847556589211,-35.2721601717609)) ;
#71609=CARTESIAN_POINT('Origin',(201.559777625407,542.847556589211,-35.0221601717607)) ;
#71610=CARTESIAN_POINT('Origin',(201.559777625407,542.847556589211,-35.2721601717609)) ;
#71611=CARTESIAN_POINT('Origin',(202.262277625408,539.09755658921,-35.8624540214915)) ;
#71612=CARTESIAN_POINT('',(202.387277625408,539.09755658921,-39.2297700580612)) ;
#71613=CARTESIAN_POINT('',(202.387277625408,539.09755658921,-35.8624540214915)) ;
#71614=CARTESIAN_POINT('',(202.262277625408,538.97255658921,-39.2297700580612)) ;
#71615=CARTESIAN_POINT('Origin',(202.262277625408,539.09755658921,-39.2297700580612)) ;
#71616=CARTESIAN_POINT('',(202.262277625408,538.97255658921,-35.8624540214915)) ;
#71617=CARTESIAN_POINT('Origin',(202.387277625408,536.368806589211,-33.7667690928544)) ;
#71618=CARTESIAN_POINT('',(202.387277625408,540.462556589212,-39.4182700580611)) ;
#71619=CARTESIAN_POINT('',(202.387277625408,540.462556589212,-37.6444650424525)) ;
#71620=CARTESIAN_POINT('',(202.387277625408,540.274056589212,-39.2297700580612)) ;
#71621=CARTESIAN_POINT('Origin',(202.387277625408,540.274056589212,-39.4182700580611)) ;
#71622=CARTESIAN_POINT('',(202.387277625408,538.988181589211,-39.2297700580612)) ;
#71623=CARTESIAN_POINT('',(202.387277625408,542.847556589211,-39.2297700580612)) ;
#71624=CARTESIAN_POINT('',(202.387277625408,542.847556589211,-33.8937690928544)) ;
#71625=CARTESIAN_POINT('',(202.387277625408,541.671056589212,-39.2297700580612)) ;
#71626=CARTESIAN_POINT('',(202.387277625408,538.988181589211,-39.2297700580612)) ;
#71627=CARTESIAN_POINT('',(202.387277625408,541.482556589212,-39.4182700580611)) ;
#71628=CARTESIAN_POINT('Origin',(202.387277625408,541.671056589212,-39.4182700580612)) ;
#71629=CARTESIAN_POINT('',(202.387277625408,541.482556589212,-39.8669650424525)) ;
#71630=CARTESIAN_POINT('Origin',(202.262277625408,542.847556589211,-33.8937690928544)) ;
#71631=CARTESIAN_POINT('',(202.262277625408,542.972556589211,-39.2297700580612)) ;
#71632=CARTESIAN_POINT('',(202.262277625408,542.972556589211,-33.8937690928544)) ;
#71633=CARTESIAN_POINT('Origin',(202.262277625408,542.847556589211,-39.2297700580612)) ;
#71634=CARTESIAN_POINT('Origin',(197.307277625408,542.972556589211,-34.0207690928544)) ;
#71635=CARTESIAN_POINT('',(201.559777625409,542.972556589211,-39.2297700580612)) ;
#71636=CARTESIAN_POINT('',(201.559777625409,542.972556589211,-38.5610190928544)) ;
#71637=CARTESIAN_POINT('',(207.753027625408,542.972556589211,-39.2297700580612)) ;
#71638=CARTESIAN_POINT('Origin',(201.57290262541,533.722556589211,-35.2721601717607)) ;
#71639=CARTESIAN_POINT('',(209.814777625407,533.722556589211,-35.0221601717611)) ;
#71640=CARTESIAN_POINT('',(209.814777625407,533.472556589211,-35.2721601717611)) ;
#71641=CARTESIAN_POINT('Origin',(209.814777625407,533.722556589211,-35.2721601717611)) ;
#71642=CARTESIAN_POINT('',(210.517277625407,533.472556589211,-35.2721601717611)) ;
#71643=CARTESIAN_POINT('',(201.57290262541,533.472556589211,-35.2721601717607)) ;
#71644=CARTESIAN_POINT('',(210.517277625407,533.722556589211,-35.0221601717611)) ;
#71645=CARTESIAN_POINT('Origin',(210.517277625407,533.722556589211,-35.2721601717611)) ;
#71646=CARTESIAN_POINT('',(201.57290262541,533.722556589211,-35.0221601717607)) ;
#71647=CARTESIAN_POINT('Origin',(210.517277625407,533.347556589211,-35.2721601717609)) ;
#71648=CARTESIAN_POINT('',(210.642277625407,533.347556589211,-35.2721601717609)) ;
#71649=CARTESIAN_POINT('',(210.892277625407,533.347556589211,-35.0221601717612)) ;
#71650=CARTESIAN_POINT('Origin',(210.892277625407,533.347556589211,-35.2721601717609)) ;
#71651=CARTESIAN_POINT('Origin',(210.517277625407,533.347556589211,-35.0221601717611)) ;
#71652=CARTESIAN_POINT('Origin',(210.517277625407,533.347556589211,-35.2721601717609)) ;
#71653=CARTESIAN_POINT('Origin',(210.892277625407,548.170681589221,-35.2721601717611)) ;
#71654=CARTESIAN_POINT('',(210.642277625407,529.59755658921,-35.2721601717612)) ;
#71655=CARTESIAN_POINT('',(210.892277625407,529.59755658921,-35.0221601717612)) ;
#71656=CARTESIAN_POINT('Origin',(210.892277625407,529.59755658921,-35.2721601717612)) ;
#71657=CARTESIAN_POINT('',(210.892277625407,548.170681589221,-35.0221601717611)) ;
#71658=CARTESIAN_POINT('',(210.642277625407,548.170681589221,-35.2721601717611)) ;
#71659=CARTESIAN_POINT('Origin',(210.517277625407,529.59755658921,-35.2721601717609)) ;
#71660=CARTESIAN_POINT('',(210.517277625407,529.47255658921,-35.2721601717609)) ;
#71661=CARTESIAN_POINT('',(210.517277625407,529.22255658921,-35.0221601717611)) ;
#71662=CARTESIAN_POINT('Origin',(210.517277625407,529.22255658921,-35.2721601717609)) ;
#71663=CARTESIAN_POINT('Origin',(210.517277625407,529.59755658921,-35.0221601717611)) ;
#71664=CARTESIAN_POINT('Origin',(210.517277625407,529.59755658921,-35.2721601717609)) ;
#71665=CARTESIAN_POINT('Origin',(205.938476772278,529.22255658921,-35.2721601717609)) ;
#71666=CARTESIAN_POINT('',(209.814777625407,529.47255658921,-35.2721601717611)) ;
#71667=CARTESIAN_POINT('',(209.814777625407,529.22255658921,-35.0221601717611)) ;
#71668=CARTESIAN_POINT('Origin',(209.814777625407,529.22255658921,-35.2721601717611)) ;
#71669=CARTESIAN_POINT('',(205.938476772278,529.22255658921,-35.0221601717609)) ;
#71670=CARTESIAN_POINT('',(205.938476772278,529.47255658921,-35.2721601717609)) ;
#71671=CARTESIAN_POINT('Origin',(209.814777625407,529.59755658921,-35.2721601717609)) ;
#71672=CARTESIAN_POINT('',(209.689777625407,529.59755658921,-35.2721601717609)) ;
#71673=CARTESIAN_POINT('',(209.439777625407,529.59755658921,-35.0221601717611)) ;
#71674=CARTESIAN_POINT('Origin',(209.439777625407,529.59755658921,-35.2721601717609)) ;
#71675=CARTESIAN_POINT('Origin',(209.814777625407,529.59755658921,-35.0221601717611)) ;
#71676=CARTESIAN_POINT('Origin',(209.814777625407,529.59755658921,-35.2721601717609)) ;
#71677=CARTESIAN_POINT('Origin',(209.439777625407,548.170681589221,-35.2721601717611)) ;
#71678=CARTESIAN_POINT('',(209.689777625407,533.347556589211,-35.2721601717611)) ;
#71679=CARTESIAN_POINT('',(209.439777625407,533.347556589211,-35.0221601717611)) ;
#71680=CARTESIAN_POINT('Origin',(209.439777625407,533.347556589211,-35.2721601717611)) ;
#71681=CARTESIAN_POINT('',(209.439777625407,548.170681589221,-35.0221601717611)) ;
#71682=CARTESIAN_POINT('',(209.689777625407,548.170681589221,-35.2721601717611)) ;
#71683=CARTESIAN_POINT('Origin',(209.814777625407,533.347556589211,-35.2721601717609)) ;
#71684=CARTESIAN_POINT('Origin',(209.814777625407,533.347556589211,-35.0221601717611)) ;
#71685=CARTESIAN_POINT('Origin',(209.814777625407,533.347556589211,-35.2721601717609)) ;
#71686=CARTESIAN_POINT('Origin',(210.517277625407,529.59755658921,-35.7037040214914)) ;
#71687=CARTESIAN_POINT('',(210.642277625407,529.59755658921,-39.2297690928544)) ;
#71688=CARTESIAN_POINT('',(210.642277625407,529.59755658921,-35.7037040214914)) ;
#71689=CARTESIAN_POINT('',(210.517277625407,529.47255658921,-39.2297690928544)) ;
#71690=CARTESIAN_POINT('Origin',(210.517277625407,529.59755658921,-39.2297690928544)) ;
#71691=CARTESIAN_POINT('',(210.517277625407,529.47255658921,-35.7037040214914)) ;
#71692=CARTESIAN_POINT('Origin',(210.642277625407,526.86880658921,-33.4492690928543)) ;
#71693=CARTESIAN_POINT('',(210.642277625407,533.347556589211,-39.2297690928544)) ;
#71694=CARTESIAN_POINT('',(210.642277625407,533.347556589211,-33.7350190928543)) ;
#71695=CARTESIAN_POINT('',(210.642277625407,529.488181589211,-39.2297690928544)) ;
#71696=CARTESIAN_POINT('Origin',(210.517277625407,533.347556589211,-33.7350190928543)) ;
#71697=CARTESIAN_POINT('',(210.517277625407,533.472556589211,-39.2297690928544)) ;
#71698=CARTESIAN_POINT('',(210.517277625407,533.472556589211,-33.7350190928543)) ;
#71699=CARTESIAN_POINT('Origin',(210.517277625407,533.347556589211,-39.2297690928544)) ;
#71700=CARTESIAN_POINT('Origin',(197.307277625407,533.472556589211,-34.0207690928544)) ;
#71701=CARTESIAN_POINT('',(209.814777625407,533.472556589211,-39.2297690928544)) ;
#71702=CARTESIAN_POINT('',(209.814777625407,533.472556589211,-38.5610190928544)) ;
#71703=CARTESIAN_POINT('',(207.753027625407,533.472556589211,-39.2297690928544)) ;
#71704=CARTESIAN_POINT('Origin',(205.838527625413,569.472556589231,-35.0221601717609)) ;
#71705=CARTESIAN_POINT('',(212.088527625407,535.548005939928,-35.0221601717612)) ;
#71706=CARTESIAN_POINT('',(199.088527625407,535.548005939932,-35.0221601717606)) ;
#71707=CARTESIAN_POINT('',(201.838527625407,535.54800593993,-35.0221601717607)) ;
#71708=CARTESIAN_POINT('',(199.088527625406,527.3971072385,-35.0221601717606)) ;
#71709=CARTESIAN_POINT('',(199.08852762541,547.972556589222,-35.0221601717606)) ;
#71710=CARTESIAN_POINT('',(212.088527625406,527.397107238496,-35.0221601717612)) ;
#71711=CARTESIAN_POINT('',(201.838527625406,527.397107238497,-35.0221601717607)) ;
#71712=CARTESIAN_POINT('',(212.08852762541,547.97255658922,-35.0221601717612)) ;
#71713=CARTESIAN_POINT('',(202.262277625407,533.722556589211,-35.0221601717608)) ;
#71714=CARTESIAN_POINT('',(201.559777625407,533.722556589211,-35.0221601717607)) ;
#71715=CARTESIAN_POINT('',(201.57290262541,533.722556589211,-35.0221601717607)) ;
#71716=CARTESIAN_POINT('',(202.637277625407,533.347556589211,-35.0221601717608)) ;
#71717=CARTESIAN_POINT('Origin',(202.262277625407,533.347556589211,-35.0221601717608)) ;
#71718=CARTESIAN_POINT('',(202.637277625407,529.59755658921,-35.0221601717608)) ;
#71719=CARTESIAN_POINT('',(202.637277625407,548.170681589221,-35.0221601717608)) ;
#71720=CARTESIAN_POINT('',(202.262277625407,529.22255658921,-35.0221601717608)) ;
#71721=CARTESIAN_POINT('Origin',(202.262277625407,529.59755658921,-35.0221601717608)) ;
#71722=CARTESIAN_POINT('',(201.559777625407,529.22255658921,-35.0221601717607)) ;
#71723=CARTESIAN_POINT('',(205.938476772278,529.22255658921,-35.0221601717609)) ;
#71724=CARTESIAN_POINT('',(201.184777625407,529.59755658921,-35.0221601717607)) ;
#71725=CARTESIAN_POINT('Origin',(201.559777625407,529.59755658921,-35.0221601717607)) ;
#71726=CARTESIAN_POINT('',(201.184777625407,533.347556589211,-35.0221601717607)) ;
#71727=CARTESIAN_POINT('',(201.184777625407,548.170681589221,-35.0221601717607)) ;
#71728=CARTESIAN_POINT('Origin',(201.559777625407,533.347556589211,-35.0221601717607)) ;
#71729=CARTESIAN_POINT('',(203.155186246464,531.472556589211,-35.0221601717609)) ;
#71730=CARTESIAN_POINT('Origin',(206.038527625407,531.472556589211,-35.0221601717609)) ;
#71731=CARTESIAN_POINT('Origin',(201.57290262541,533.722556589211,-35.2721601717607)) ;
#71732=CARTESIAN_POINT('',(201.559777625407,533.472556589211,-35.2721601717607)) ;
#71733=CARTESIAN_POINT('Origin',(201.559777625407,533.722556589211,-35.2721601717607)) ;
#71734=CARTESIAN_POINT('',(202.262277625407,533.472556589211,-35.2721601717608)) ;
#71735=CARTESIAN_POINT('',(201.57290262541,533.472556589211,-35.2721601717607)) ;
#71736=CARTESIAN_POINT('Origin',(202.262277625407,533.722556589211,-35.2721601717608)) ;
#71737=CARTESIAN_POINT('Origin',(202.262277625407,533.347556589211,-35.2721601717609)) ;
#71738=CARTESIAN_POINT('',(202.387277625407,533.347556589211,-35.2721601717609)) ;
#71739=CARTESIAN_POINT('Origin',(202.637277625407,533.347556589211,-35.2721601717609)) ;
#71740=CARTESIAN_POINT('Origin',(202.262277625407,533.347556589211,-35.2721601717609)) ;
#71741=CARTESIAN_POINT('Origin',(202.637277625407,548.170681589221,-35.2721601717608)) ;
#71742=CARTESIAN_POINT('',(202.387277625407,529.59755658921,-35.2721601717608)) ;
#71743=CARTESIAN_POINT('Origin',(202.637277625407,529.59755658921,-35.2721601717608)) ;
#71744=CARTESIAN_POINT('',(202.387277625407,548.170681589221,-35.2721601717608)) ;
#71745=CARTESIAN_POINT('Origin',(202.262277625407,529.59755658921,-35.2721601717609)) ;
#71746=CARTESIAN_POINT('',(202.262277625407,529.47255658921,-35.2721601717609)) ;
#71747=CARTESIAN_POINT('Origin',(202.262277625407,529.22255658921,-35.2721601717609)) ;
#71748=CARTESIAN_POINT('Origin',(202.262277625407,529.59755658921,-35.2721601717609)) ;
#71749=CARTESIAN_POINT('Origin',(205.938476772278,529.22255658921,-35.2721601717609)) ;
#71750=CARTESIAN_POINT('',(201.559777625407,529.47255658921,-35.2721601717607)) ;
#71751=CARTESIAN_POINT('Origin',(201.559777625407,529.22255658921,-35.2721601717607)) ;
#71752=CARTESIAN_POINT('',(205.938476772278,529.47255658921,-35.2721601717609)) ;
#71753=CARTESIAN_POINT('Origin',(201.559777625407,529.59755658921,-35.2721601717609)) ;
#71754=CARTESIAN_POINT('Origin',(201.184777625407,529.59755658921,-35.2721601717609)) ;
#71755=CARTESIAN_POINT('Origin',(201.559777625407,529.59755658921,-35.2721601717609)) ;
#71756=CARTESIAN_POINT('Origin',(201.184777625407,548.170681589221,-35.2721601717607)) ;
#71757=CARTESIAN_POINT('Origin',(201.184777625407,533.347556589211,-35.2721601717607)) ;
#71758=CARTESIAN_POINT('Origin',(201.559777625407,533.347556589211,-35.2721601717609)) ;
#71759=CARTESIAN_POINT('Origin',(201.559777625407,533.347556589211,-35.2721601717609)) ;
#71760=CARTESIAN_POINT('Origin',(202.262277625407,529.59755658921,-35.8624540214915)) ;
#71761=CARTESIAN_POINT('',(202.387277625407,529.59755658921,-39.2297700580612)) ;
#71762=CARTESIAN_POINT('',(202.387277625407,529.59755658921,-35.8624540214915)) ;
#71763=CARTESIAN_POINT('',(202.262277625407,529.47255658921,-39.2297700580612)) ;
#71764=CARTESIAN_POINT('Origin',(202.262277625407,529.59755658921,-39.2297700580612)) ;
#71765=CARTESIAN_POINT('',(202.262277625407,529.47255658921,-35.8624540214915)) ;
#71766=CARTESIAN_POINT('Origin',(202.387277625407,526.868806589211,-33.7667690928544)) ;
#71767=CARTESIAN_POINT('',(202.387277625407,533.347556589211,-39.2297700580612)) ;
#71768=CARTESIAN_POINT('',(202.387277625407,533.347556589211,-33.8937690928544)) ;
#71769=CARTESIAN_POINT('',(202.387277625407,532.171056589212,-39.2297700580612)) ;
#71770=CARTESIAN_POINT('',(202.387277625407,529.488181589211,-39.2297700580612)) ;
#71771=CARTESIAN_POINT('',(202.387277625407,531.982556589212,-39.4182700580611)) ;
#71772=CARTESIAN_POINT('Origin',(202.387277625407,532.171056589212,-39.4182700580612)) ;
#71773=CARTESIAN_POINT('',(202.387277625407,531.982556589212,-39.8669650424525)) ;
#71774=CARTESIAN_POINT('',(202.387277625407,530.962556589212,-39.4182700580611)) ;
#71775=CARTESIAN_POINT('',(202.387277625407,530.962556589212,-37.6444650424525)) ;
#71776=CARTESIAN_POINT('',(202.387277625407,530.774056589212,-39.2297700580612)) ;
#71777=CARTESIAN_POINT('Origin',(202.387277625407,530.774056589212,-39.4182700580611)) ;
#71778=CARTESIAN_POINT('',(202.387277625407,529.488181589211,-39.2297700580612)) ;
#71779=CARTESIAN_POINT('Origin',(202.262277625407,533.347556589211,-33.8937690928544)) ;
#71780=CARTESIAN_POINT('',(202.262277625407,533.472556589211,-39.2297700580612)) ;
#71781=CARTESIAN_POINT('',(202.262277625407,533.472556589211,-33.8937690928544)) ;
#71782=CARTESIAN_POINT('Origin',(202.262277625407,533.347556589211,-39.2297700580612)) ;
#71783=CARTESIAN_POINT('Origin',(197.307277625407,533.472556589211,-34.0207690928544)) ;
#71784=CARTESIAN_POINT('',(201.559777625407,533.472556589211,-39.2297700580612)) ;
#71785=CARTESIAN_POINT('',(201.559777625407,533.472556589211,-38.5610190928544)) ;
#71786=CARTESIAN_POINT('',(207.753027625407,533.472556589211,-39.2297700580612)) ;
#71787=CARTESIAN_POINT('Origin',(206.038425919142,529.47255658921,-37.9581389501285)) ;
#71788=CARTESIAN_POINT('',(201.559777625407,529.47255658921,-39.2297700580612)) ;
#71789=CARTESIAN_POINT('',(212.118601772275,529.47255658921,-39.2297700580611)) ;
#71790=CARTESIAN_POINT('',(201.559777625407,529.47255658921,-40.5297040214914)) ;
#71791=CARTESIAN_POINT('Origin',(201.559777625407,529.59755658921,-40.5297040214914)) ;
#71792=CARTESIAN_POINT('Origin',(201.559777625407,529.59755658921,-39.2297700580612)) ;
#71793=CARTESIAN_POINT('Origin',(201.559777625407,533.347556589211,-38.5610190928544)) ;
#71794=CARTESIAN_POINT('Origin',(201.559777625407,533.347556589211,-39.2297700580612)) ;
#71795=CARTESIAN_POINT('Origin',(206.038425919142,529.47255658921,-37.9581389501285)) ;
#71796=CARTESIAN_POINT('',(209.814777625407,529.47255658921,-39.2297690928544)) ;
#71797=CARTESIAN_POINT('',(212.118601772275,529.47255658921,-39.2297690928544)) ;
#71798=CARTESIAN_POINT('',(209.814777625407,529.47255658921,-40.5297040214914)) ;
#71799=CARTESIAN_POINT('Origin',(209.814777625407,529.59755658921,-40.5297040214914)) ;
#71800=CARTESIAN_POINT('',(209.689777625407,529.59755658921,-39.2297690928544)) ;
#71801=CARTESIAN_POINT('Origin',(209.814777625407,529.59755658921,-39.2297690928544)) ;
#71802=CARTESIAN_POINT('',(209.689777625407,529.59755658921,-40.5297040214914)) ;
#71803=CARTESIAN_POINT('Origin',(209.814777625407,533.347556589211,-38.5610190928544)) ;
#71804=CARTESIAN_POINT('',(209.689777625407,533.347556589211,-39.2297690928544)) ;
#71805=CARTESIAN_POINT('',(209.689777625407,533.347556589211,-38.5610190928544)) ;
#71806=CARTESIAN_POINT('Origin',(209.814777625407,533.347556589211,-39.2297690928544)) ;
#71807=CARTESIAN_POINT('Origin',(209.689777625407,526.868806589211,-43.1012690928544)) ;
#71808=CARTESIAN_POINT('',(209.689777625407,529.488181589211,-39.2297690928544)) ;
#71809=CARTESIAN_POINT('Origin',(202.466652625407,535.044431589211,-37.0052690928544)) ;
#71810=CARTESIAN_POINT('',(208.771027625407,531.472556589211,-37.0052690928544)) ;
#71811=CARTESIAN_POINT('Origin',(206.038527625407,531.472556589211,-37.0052690928544)) ;
#71812=CARTESIAN_POINT('Origin',(202.262277625407,531.982556589212,-39.8669650424525)) ;
#71813=CARTESIAN_POINT('Origin',(202.262277625407,531.982556589212,-39.4182700580611)) ;
#71814=CARTESIAN_POINT('Origin',(212.118601772275,529.59755658921,-39.2297700580611)) ;
#71815=CARTESIAN_POINT('',(201.559777625407,529.59755658921,-39.3547700580611)) ;
#71816=CARTESIAN_POINT('Origin',(201.559777625407,529.59755658921,-39.2297700580612)) ;
#71817=CARTESIAN_POINT('',(202.262277625407,529.59755658921,-39.3547700580611)) ;
#71818=CARTESIAN_POINT('Origin',(202.262277625407,529.59755658921,-39.2297700580612)) ;
#71819=CARTESIAN_POINT('',(212.118601772275,529.59755658921,-39.3547700580611)) ;
#71820=CARTESIAN_POINT('Origin',(202.262277625407,532.171056589212,-39.4182700580612)) ;
#71821=CARTESIAN_POINT('',(202.262277625407,532.171056589212,-39.3547700580612)) ;
#71822=CARTESIAN_POINT('Origin',(202.262277625407,532.171056589212,-39.4182700580612)) ;
#71823=CARTESIAN_POINT('Origin',(202.262277625407,532.171056589212,-39.2297700580612)) ;
#71824=CARTESIAN_POINT('Origin',(202.262277625407,529.488181589211,-39.2297700580612)) ;
#71825=CARTESIAN_POINT('',(202.262277625407,533.347556589211,-39.3547700580612)) ;
#71826=CARTESIAN_POINT('Origin',(202.262277625407,533.347556589211,-39.2297700580612)) ;
#71827=CARTESIAN_POINT('',(202.262277625407,529.488181589211,-39.3547700580611)) ;
#71828=CARTESIAN_POINT('Origin',(201.559777625407,532.171056589212,-39.4182700580612)) ;
#71829=CARTESIAN_POINT('',(201.559777625407,532.171056589212,-39.3547700580612)) ;
#71830=CARTESIAN_POINT('Origin',(201.559777625407,532.171056589212,-39.4182700580612)) ;
#71831=CARTESIAN_POINT('Origin',(201.559777625407,532.171056589212,-39.2297700580612)) ;
#71832=CARTESIAN_POINT('Origin',(202.262277625407,530.774056589212,-39.4182700580611)) ;
#71833=CARTESIAN_POINT('',(202.262277625407,530.837556589212,-39.4182700580611)) ;
#71834=CARTESIAN_POINT('',(202.262277625407,530.774056589212,-39.3547700580611)) ;
#71835=CARTESIAN_POINT('Origin',(202.262277625407,530.774056589212,-39.4182700580611)) ;
#71836=CARTESIAN_POINT('Origin',(202.262277625407,530.774056589212,-39.2297700580612)) ;
#71837=CARTESIAN_POINT('Origin',(202.262277625407,530.962556589212,-39.4182700580611)) ;
#71838=CARTESIAN_POINT('Origin',(202.262277625407,530.962556589212,-37.6444650424525)) ;
#71839=CARTESIAN_POINT('',(202.262277625407,530.837556589212,-37.6444650424525)) ;
#71840=CARTESIAN_POINT('Origin',(202.262277625407,529.488181589211,-39.2297700580612)) ;
#71841=CARTESIAN_POINT('Origin',(202.262277625407,529.59755658921,-39.2297700580612)) ;
#71842=CARTESIAN_POINT('',(202.262277625407,529.488181589211,-39.3547700580611)) ;
#71843=CARTESIAN_POINT('Origin',(201.559777625407,530.774056589212,-39.4182700580611)) ;
#71844=CARTESIAN_POINT('',(201.559777625407,530.774056589212,-39.3547700580611)) ;
#71845=CARTESIAN_POINT('Origin',(201.559777625407,530.774056589212,-39.4182700580611)) ;
#71846=CARTESIAN_POINT('Origin',(201.559777625407,530.774056589212,-39.2297700580612)) ;
#71847=CARTESIAN_POINT('Origin',(201.559777625407,529.488181589211,-39.2297700580612)) ;
#71848=CARTESIAN_POINT('Origin',(201.559777625407,529.59755658921,-39.2297700580612)) ;
#71849=CARTESIAN_POINT('',(201.559777625407,529.488181589211,-39.3547700580611)) ;
#71850=CARTESIAN_POINT('Origin',(219.024277625406,530.774056589212,-39.4182700580611)) ;
#71851=CARTESIAN_POINT('',(219.024277625406,530.774056589212,-39.3547700580611)) ;
#71852=CARTESIAN_POINT('',(219.024277625406,530.837556589212,-39.4182700580611)) ;
#71853=CARTESIAN_POINT('Origin',(201.559777625407,529.488181589211,-39.2297700580612)) ;
#71854=CARTESIAN_POINT('',(201.559777625407,533.347556589211,-39.3547700580611)) ;
#71855=CARTESIAN_POINT('Origin',(201.559777625407,533.347556589211,-39.2297700580612)) ;
#71856=CARTESIAN_POINT('',(201.559777625407,529.488181589211,-39.3547700580611)) ;
#71857=CARTESIAN_POINT('Origin',(218.198777625406,532.171056589212,-39.4182700580611)) ;
#71858=CARTESIAN_POINT('',(218.198777625406,532.171056589212,-39.3547700580611)) ;
#71859=CARTESIAN_POINT('Origin',(201.559777625407,529.59755658921,-39.2297700580612)) ;
#71860=CARTESIAN_POINT('Origin',(202.262277625407,529.59755658921,-39.2297700580612)) ;
#71861=CARTESIAN_POINT('Origin',(207.753027625407,533.347556589211,-39.2297700580612)) ;
#71862=CARTESIAN_POINT('Origin',(201.559777625407,533.347556589211,-39.2297700580612)) ;
#71863=CARTESIAN_POINT('',(207.753027625407,533.347556589211,-39.3547700580611)) ;
#71864=CARTESIAN_POINT('Origin',(202.262277625407,533.347556589211,-39.2297700580612)) ;
#71865=CARTESIAN_POINT('Origin',(201.559777625407,533.347556589211,-39.2297700580612)) ;
#71866=CARTESIAN_POINT('Origin',(202.262277625407,533.347556589211,-39.2297700580612)) ;
#71867=CARTESIAN_POINT('Origin',(219.849777625406,530.837556589212,-41.5221609920506)) ;
#71868=CARTESIAN_POINT('Origin',(218.198777625407,532.107556589211,-39.3547700580611)) ;
#71869=CARTESIAN_POINT('Origin',(218.198777625407,532.107556589211,-39.3547700580611)) ;
#71870=CARTESIAN_POINT('Origin',(218.198777625407,532.107556589211,-39.3547690928544)) ;
#71871=CARTESIAN_POINT('',(209.814777625407,533.347556589211,-39.3547690928544)) ;
#71872=CARTESIAN_POINT('',(209.814777625407,529.59755658921,-39.3547690928544)) ;
#71873=CARTESIAN_POINT('',(209.814777625407,529.488181589211,-39.3547690928544)) ;
#71874=CARTESIAN_POINT('',(210.517277625407,529.59755658921,-39.3547690928544)) ;
#71875=CARTESIAN_POINT('',(212.118601772274,529.59755658921,-39.3547690928544)) ;
#71876=CARTESIAN_POINT('',(210.517277625407,533.347556589211,-39.3547690928544)) ;
#71877=CARTESIAN_POINT('',(210.517277625407,529.488181589211,-39.3547690928544)) ;
#71878=CARTESIAN_POINT('',(207.753027625407,533.347556589211,-39.3547690928544)) ;
#71879=CARTESIAN_POINT('Origin',(209.814777625407,529.59755658921,-39.2297690928544)) ;
#71880=CARTESIAN_POINT('Origin',(209.814777625407,529.59755658921,-39.2297690928544)) ;
#71881=CARTESIAN_POINT('Origin',(209.814777625407,529.59755658921,-39.2297690928544)) ;
#71882=CARTESIAN_POINT('Origin',(209.814777625407,533.347556589211,-39.2297690928544)) ;
#71883=CARTESIAN_POINT('Origin',(209.814777625407,533.347556589211,-39.2297690928544)) ;
#71884=CARTESIAN_POINT('Origin',(209.814777625407,533.347556589211,-39.2297690928544)) ;
#71885=CARTESIAN_POINT('Origin',(209.814777625407,529.488181589211,-39.2297690928544)) ;
#71886=CARTESIAN_POINT('Origin',(207.753027625407,533.347556589211,-39.2297690928544)) ;
#71887=CARTESIAN_POINT('Origin',(210.517277625407,533.347556589211,-39.2297690928544)) ;
#71888=CARTESIAN_POINT('Origin',(212.118601772274,529.59755658921,-39.2297690928544)) ;
#71889=CARTESIAN_POINT('Origin',(210.517277625407,529.59755658921,-39.2297690928544)) ;
#71890=CARTESIAN_POINT('Origin',(210.517277625407,529.488181589211,-39.2297690928544)) ;
#71891=CARTESIAN_POINT('Origin',(210.517277625407,529.59755658921,-39.2297690928544)) ;
#71892=CARTESIAN_POINT('Origin',(210.517277625407,533.347556589211,-39.2297690928544)) ;
#71893=CARTESIAN_POINT('Origin',(210.517277625407,529.59755658921,-39.2297690928544)) ;
#71894=CARTESIAN_POINT('Origin',(210.517277625407,533.347556589211,-39.2297690928544)) ;
#71895=CARTESIAN_POINT('Origin',(202.262277625408,541.482556589212,-39.8669650424525)) ;
#71896=CARTESIAN_POINT('Origin',(202.262277625408,541.482556589212,-39.4182700580611)) ;
#71897=CARTESIAN_POINT('Origin',(212.118601772276,539.09755658921,-39.2297700580611)) ;
#71898=CARTESIAN_POINT('',(201.559777625409,538.97255658921,-39.2297700580612)) ;
#71899=CARTESIAN_POINT('',(201.559777625409,539.09755658921,-39.3547700580611)) ;
#71900=CARTESIAN_POINT('Origin',(201.559777625409,539.09755658921,-39.2297700580612)) ;
#71901=CARTESIAN_POINT('',(212.118601772276,538.97255658921,-39.2297700580611)) ;
#71902=CARTESIAN_POINT('',(202.262277625408,539.09755658921,-39.3547700580611)) ;
#71903=CARTESIAN_POINT('Origin',(202.262277625408,539.09755658921,-39.2297700580612)) ;
#71904=CARTESIAN_POINT('',(212.118601772276,539.09755658921,-39.3547700580611)) ;
#71905=CARTESIAN_POINT('Origin',(202.262277625408,541.671056589212,-39.4182700580612)) ;
#71906=CARTESIAN_POINT('',(202.262277625408,541.671056589212,-39.3547700580612)) ;
#71907=CARTESIAN_POINT('Origin',(202.262277625408,541.671056589212,-39.4182700580612)) ;
#71908=CARTESIAN_POINT('Origin',(202.262277625408,541.671056589212,-39.2297700580612)) ;
#71909=CARTESIAN_POINT('Origin',(202.262277625408,538.988181589211,-39.2297700580612)) ;
#71910=CARTESIAN_POINT('',(202.262277625408,542.847556589211,-39.3547700580612)) ;
#71911=CARTESIAN_POINT('Origin',(202.262277625408,542.847556589211,-39.2297700580612)) ;
#71912=CARTESIAN_POINT('',(202.262277625408,538.988181589211,-39.3547700580611)) ;
#71913=CARTESIAN_POINT('Origin',(201.559777625409,541.671056589212,-39.4182700580612)) ;
#71914=CARTESIAN_POINT('',(201.559777625409,541.671056589212,-39.3547700580612)) ;
#71915=CARTESIAN_POINT('Origin',(201.559777625409,541.671056589212,-39.4182700580612)) ;
#71916=CARTESIAN_POINT('Origin',(201.559777625409,541.671056589212,-39.2297700580612)) ;
#71917=CARTESIAN_POINT('Origin',(202.262277625408,540.274056589212,-39.4182700580611)) ;
#71918=CARTESIAN_POINT('',(202.262277625408,540.337556589212,-39.4182700580611)) ;
#71919=CARTESIAN_POINT('',(202.262277625408,540.274056589212,-39.3547700580611)) ;
#71920=CARTESIAN_POINT('Origin',(202.262277625408,540.274056589212,-39.4182700580611)) ;
#71921=CARTESIAN_POINT('Origin',(202.262277625408,540.274056589212,-39.2297700580612)) ;
#71922=CARTESIAN_POINT('Origin',(202.262277625408,540.462556589212,-39.4182700580611)) ;
#71923=CARTESIAN_POINT('Origin',(202.262277625408,540.462556589212,-37.6444650424525)) ;
#71924=CARTESIAN_POINT('',(202.262277625408,540.337556589212,-37.6444650424525)) ;
#71925=CARTESIAN_POINT('Origin',(202.262277625408,538.988181589211,-39.2297700580612)) ;
#71926=CARTESIAN_POINT('Origin',(202.262277625408,539.09755658921,-39.2297700580612)) ;
#71927=CARTESIAN_POINT('',(202.262277625408,538.988181589211,-39.3547700580611)) ;
#71928=CARTESIAN_POINT('Origin',(201.559777625409,540.274056589212,-39.4182700580611)) ;
#71929=CARTESIAN_POINT('',(201.559777625409,540.274056589212,-39.3547700580611)) ;
#71930=CARTESIAN_POINT('Origin',(201.559777625409,540.274056589212,-39.4182700580611)) ;
#71931=CARTESIAN_POINT('Origin',(201.559777625409,540.274056589212,-39.2297700580612)) ;
#71932=CARTESIAN_POINT('Origin',(201.559777625409,538.988181589211,-39.2297700580612)) ;
#71933=CARTESIAN_POINT('Origin',(201.559777625409,539.09755658921,-39.2297700580612)) ;
#71934=CARTESIAN_POINT('',(201.559777625409,538.988181589211,-39.3547700580611)) ;
#71935=CARTESIAN_POINT('Origin',(219.024277625408,540.274056589212,-39.4182700580611)) ;
#71936=CARTESIAN_POINT('',(219.024277625408,540.274056589212,-39.3547700580611)) ;
#71937=CARTESIAN_POINT('',(219.024277625408,540.337556589212,-39.4182700580611)) ;
#71938=CARTESIAN_POINT('Origin',(201.559777625409,538.988181589211,-39.2297700580612)) ;
#71939=CARTESIAN_POINT('',(201.559777625409,542.847556589211,-39.3547700580611)) ;
#71940=CARTESIAN_POINT('Origin',(201.559777625409,542.847556589211,-39.2297700580612)) ;
#71941=CARTESIAN_POINT('',(201.559777625409,538.988181589211,-39.3547700580611)) ;
#71942=CARTESIAN_POINT('Origin',(218.198777625408,541.671056589212,-39.4182700580611)) ;
#71943=CARTESIAN_POINT('',(218.198777625408,541.671056589212,-39.3547700580611)) ;
#71944=CARTESIAN_POINT('Origin',(201.559777625409,539.09755658921,-39.2297700580612)) ;
#71945=CARTESIAN_POINT('Origin',(201.559777625409,539.09755658921,-39.2297700580612)) ;
#71946=CARTESIAN_POINT('Origin',(202.262277625408,539.09755658921,-39.2297700580612)) ;
#71947=CARTESIAN_POINT('Origin',(207.753027625408,542.847556589211,-39.2297700580612)) ;
#71948=CARTESIAN_POINT('Origin',(201.559777625409,542.847556589211,-39.2297700580612)) ;
#71949=CARTESIAN_POINT('',(207.753027625408,542.847556589211,-39.3547700580611)) ;
#71950=CARTESIAN_POINT('Origin',(202.262277625408,542.847556589211,-39.2297700580612)) ;
#71951=CARTESIAN_POINT('Origin',(201.559777625409,542.847556589211,-39.2297700580612)) ;
#71952=CARTESIAN_POINT('Origin',(201.559777625409,542.847556589211,-39.2297700580612)) ;
#71953=CARTESIAN_POINT('Origin',(202.262277625408,542.847556589211,-39.2297700580612)) ;
#71954=CARTESIAN_POINT('Origin',(219.849777625407,540.337556589212,-41.5221609920506)) ;
#71955=CARTESIAN_POINT('Origin',(218.198777625408,541.607556589211,-39.3547700580611)) ;
#71956=CARTESIAN_POINT('Origin',(218.198777625408,541.607556589211,-39.3547700580611)) ;
#71957=CARTESIAN_POINT('Origin',(218.198777625408,541.607556589211,-39.3547690928544)) ;
#71958=CARTESIAN_POINT('',(209.814777625408,542.847556589211,-39.3547690928544)) ;
#71959=CARTESIAN_POINT('',(209.814777625408,539.09755658921,-39.3547690928544)) ;
#71960=CARTESIAN_POINT('',(209.814777625408,538.988181589211,-39.3547690928544)) ;
#71961=CARTESIAN_POINT('',(210.517277625409,539.09755658921,-39.3547690928544)) ;
#71962=CARTESIAN_POINT('',(212.118601772276,539.09755658921,-39.3547690928544)) ;
#71963=CARTESIAN_POINT('',(210.517277625409,542.847556589211,-39.3547690928544)) ;
#71964=CARTESIAN_POINT('',(210.517277625409,538.988181589211,-39.3547690928544)) ;
#71965=CARTESIAN_POINT('',(207.753027625408,542.847556589211,-39.3547690928544)) ;
#71966=CARTESIAN_POINT('Origin',(209.814777625408,539.09755658921,-39.2297690928544)) ;
#71967=CARTESIAN_POINT('',(209.814777625408,538.97255658921,-39.2297690928544)) ;
#71968=CARTESIAN_POINT('Origin',(209.814777625408,539.09755658921,-39.2297690928544)) ;
#71969=CARTESIAN_POINT('',(209.689777625408,539.09755658921,-39.2297690928544)) ;
#71970=CARTESIAN_POINT('Origin',(209.814777625408,539.09755658921,-39.2297690928544)) ;
#71971=CARTESIAN_POINT('Origin',(209.814777625408,539.09755658921,-39.2297690928544)) ;
#71972=CARTESIAN_POINT('Origin',(209.814777625408,542.847556589211,-39.2297690928544)) ;
#71973=CARTESIAN_POINT('',(209.689777625408,542.847556589211,-39.2297690928544)) ;
#71974=CARTESIAN_POINT('Origin',(209.814777625408,542.847556589211,-39.2297690928544)) ;
#71975=CARTESIAN_POINT('Origin',(209.814777625408,542.847556589211,-39.2297690928544)) ;
#71976=CARTESIAN_POINT('Origin',(209.814777625408,542.847556589211,-39.2297690928544)) ;
#71977=CARTESIAN_POINT('Origin',(209.814777625408,538.988181589211,-39.2297690928544)) ;
#71978=CARTESIAN_POINT('',(209.689777625408,538.988181589211,-39.2297690928544)) ;
#71979=CARTESIAN_POINT('Origin',(207.753027625408,542.847556589211,-39.2297690928544)) ;
#71980=CARTESIAN_POINT('Origin',(210.517277625409,542.847556589211,-39.2297690928544)) ;
#71981=CARTESIAN_POINT('Origin',(212.118601772276,539.09755658921,-39.2297690928544)) ;
#71982=CARTESIAN_POINT('',(212.118601772276,538.97255658921,-39.2297690928544)) ;
#71983=CARTESIAN_POINT('Origin',(210.517277625409,539.09755658921,-39.2297690928544)) ;
#71984=CARTESIAN_POINT('Origin',(210.517277625409,538.988181589211,-39.2297690928544)) ;
#71985=CARTESIAN_POINT('Origin',(210.517277625409,539.09755658921,-39.2297690928544)) ;
#71986=CARTESIAN_POINT('Origin',(210.517277625409,542.847556589211,-39.2297690928544)) ;
#71987=CARTESIAN_POINT('Origin',(210.517277625409,539.09755658921,-39.2297690928544)) ;
#71988=CARTESIAN_POINT('Origin',(210.517277625409,542.847556589211,-39.2297690928544)) ;
#71989=CARTESIAN_POINT('Origin',(202.26227762541,550.982556589212,-39.8669650424525)) ;
#71990=CARTESIAN_POINT('Origin',(202.26227762541,550.982556589212,-39.4182700580611)) ;
#71991=CARTESIAN_POINT('Origin',(212.118601772278,548.59755658921,-39.2297700580611)) ;
#71992=CARTESIAN_POINT('',(201.55977762541,548.47255658921,-39.2297700580612)) ;
#71993=CARTESIAN_POINT('',(201.55977762541,548.59755658921,-39.3547700580611)) ;
#71994=CARTESIAN_POINT('Origin',(201.55977762541,548.59755658921,-39.2297700580612)) ;
#71995=CARTESIAN_POINT('',(212.118601772278,548.47255658921,-39.2297700580611)) ;
#71996=CARTESIAN_POINT('',(202.26227762541,548.59755658921,-39.3547700580611)) ;
#71997=CARTESIAN_POINT('Origin',(202.26227762541,548.59755658921,-39.2297700580612)) ;
#71998=CARTESIAN_POINT('',(212.118601772278,548.59755658921,-39.3547700580611)) ;
#71999=CARTESIAN_POINT('Origin',(202.26227762541,551.171056589212,-39.4182700580612)) ;
#72000=CARTESIAN_POINT('',(202.26227762541,551.171056589212,-39.3547700580612)) ;
#72001=CARTESIAN_POINT('Origin',(202.26227762541,551.171056589212,-39.4182700580612)) ;
#72002=CARTESIAN_POINT('Origin',(202.26227762541,551.171056589212,-39.2297700580612)) ;
#72003=CARTESIAN_POINT('Origin',(202.26227762541,548.488181589211,-39.2297700580612)) ;
#72004=CARTESIAN_POINT('',(202.26227762541,552.347556589211,-39.3547700580612)) ;
#72005=CARTESIAN_POINT('Origin',(202.26227762541,552.347556589211,-39.2297700580612)) ;
#72006=CARTESIAN_POINT('',(202.26227762541,548.488181589211,-39.3547700580611)) ;
#72007=CARTESIAN_POINT('Origin',(201.55977762541,551.171056589212,-39.4182700580612)) ;
#72008=CARTESIAN_POINT('',(201.55977762541,551.171056589212,-39.3547700580612)) ;
#72009=CARTESIAN_POINT('Origin',(201.55977762541,551.171056589212,-39.4182700580612)) ;
#72010=CARTESIAN_POINT('Origin',(201.55977762541,551.171056589212,-39.2297700580612)) ;
#72011=CARTESIAN_POINT('Origin',(202.26227762541,549.774056589212,-39.4182700580611)) ;
#72012=CARTESIAN_POINT('',(202.26227762541,549.837556589212,-39.4182700580611)) ;
#72013=CARTESIAN_POINT('',(202.26227762541,549.774056589212,-39.3547700580611)) ;
#72014=CARTESIAN_POINT('Origin',(202.26227762541,549.774056589212,-39.4182700580611)) ;
#72015=CARTESIAN_POINT('Origin',(202.26227762541,549.774056589212,-39.2297700580612)) ;
#72016=CARTESIAN_POINT('Origin',(202.26227762541,549.962556589212,-39.4182700580611)) ;
#72017=CARTESIAN_POINT('Origin',(202.26227762541,549.962556589212,-37.6444650424525)) ;
#72018=CARTESIAN_POINT('',(202.26227762541,549.837556589212,-37.6444650424525)) ;
#72019=CARTESIAN_POINT('Origin',(202.26227762541,548.488181589211,-39.2297700580612)) ;
#72020=CARTESIAN_POINT('Origin',(202.26227762541,548.59755658921,-39.2297700580612)) ;
#72021=CARTESIAN_POINT('',(202.26227762541,548.488181589211,-39.3547700580611)) ;
#72022=CARTESIAN_POINT('Origin',(201.55977762541,549.774056589212,-39.4182700580611)) ;
#72023=CARTESIAN_POINT('',(201.55977762541,549.774056589212,-39.3547700580611)) ;
#72024=CARTESIAN_POINT('Origin',(201.55977762541,549.774056589212,-39.4182700580611)) ;
#72025=CARTESIAN_POINT('Origin',(201.55977762541,549.774056589212,-39.2297700580612)) ;
#72026=CARTESIAN_POINT('Origin',(201.55977762541,548.488181589211,-39.2297700580612)) ;
#72027=CARTESIAN_POINT('Origin',(201.55977762541,548.59755658921,-39.2297700580612)) ;
#72028=CARTESIAN_POINT('',(201.55977762541,548.488181589211,-39.3547700580611)) ;
#72029=CARTESIAN_POINT('Origin',(219.024277625409,549.774056589212,-39.4182700580611)) ;
#72030=CARTESIAN_POINT('',(219.024277625409,549.774056589212,-39.3547700580611)) ;
#72031=CARTESIAN_POINT('',(219.024277625409,549.837556589212,-39.4182700580611)) ;
#72032=CARTESIAN_POINT('Origin',(201.55977762541,548.488181589211,-39.2297700580612)) ;
#72033=CARTESIAN_POINT('',(201.55977762541,552.347556589211,-39.3547700580611)) ;
#72034=CARTESIAN_POINT('Origin',(201.55977762541,552.347556589211,-39.2297700580612)) ;
#72035=CARTESIAN_POINT('',(201.55977762541,548.488181589211,-39.3547700580611)) ;
#72036=CARTESIAN_POINT('Origin',(218.198777625409,551.171056589212,-39.4182700580611)) ;
#72037=CARTESIAN_POINT('',(218.198777625409,551.171056589212,-39.3547700580611)) ;
#72038=CARTESIAN_POINT('Origin',(201.55977762541,548.59755658921,-39.2297700580612)) ;
#72039=CARTESIAN_POINT('Origin',(201.55977762541,548.59755658921,-39.2297700580612)) ;
#72040=CARTESIAN_POINT('Origin',(202.26227762541,548.59755658921,-39.2297700580612)) ;
#72041=CARTESIAN_POINT('Origin',(207.75302762541,552.347556589211,-39.2297700580612)) ;
#72042=CARTESIAN_POINT('Origin',(201.55977762541,552.347556589211,-39.2297700580612)) ;
#72043=CARTESIAN_POINT('',(207.75302762541,552.347556589211,-39.3547700580611)) ;
#72044=CARTESIAN_POINT('Origin',(202.26227762541,552.347556589211,-39.2297700580612)) ;
#72045=CARTESIAN_POINT('Origin',(201.55977762541,552.347556589211,-39.2297700580612)) ;
#72046=CARTESIAN_POINT('Origin',(201.55977762541,552.347556589211,-39.2297700580612)) ;
#72047=CARTESIAN_POINT('Origin',(202.26227762541,552.347556589211,-39.2297700580612)) ;
#72048=CARTESIAN_POINT('Origin',(219.849777625409,549.837556589212,-41.5221609920506)) ;
#72049=CARTESIAN_POINT('Origin',(218.19877762541,551.107556589211,-39.3547700580611)) ;
#72050=CARTESIAN_POINT('Origin',(218.19877762541,551.107556589211,-39.3547700580611)) ;
#72051=CARTESIAN_POINT('Origin',(218.19877762541,551.107556589211,-39.3547690928544)) ;
#72052=CARTESIAN_POINT('',(209.81477762541,552.347556589211,-39.3547690928544)) ;
#72053=CARTESIAN_POINT('',(209.81477762541,548.59755658921,-39.3547690928544)) ;
#72054=CARTESIAN_POINT('',(209.81477762541,548.488181589211,-39.3547690928544)) ;
#72055=CARTESIAN_POINT('',(210.51727762541,548.59755658921,-39.3547690928544)) ;
#72056=CARTESIAN_POINT('',(212.118601772278,548.59755658921,-39.3547690928544)) ;
#72057=CARTESIAN_POINT('',(210.51727762541,552.347556589211,-39.3547690928544)) ;
#72058=CARTESIAN_POINT('',(210.51727762541,548.488181589211,-39.3547690928544)) ;
#72059=CARTESIAN_POINT('',(207.75302762541,552.347556589211,-39.3547690928544)) ;
#72060=CARTESIAN_POINT('Origin',(209.81477762541,548.59755658921,-39.2297690928544)) ;
#72061=CARTESIAN_POINT('',(209.81477762541,548.47255658921,-39.2297690928544)) ;
#72062=CARTESIAN_POINT('Origin',(209.81477762541,548.59755658921,-39.2297690928544)) ;
#72063=CARTESIAN_POINT('',(209.68977762541,548.59755658921,-39.2297690928544)) ;
#72064=CARTESIAN_POINT('Origin',(209.81477762541,548.59755658921,-39.2297690928544)) ;
#72065=CARTESIAN_POINT('Origin',(209.81477762541,548.59755658921,-39.2297690928544)) ;
#72066=CARTESIAN_POINT('Origin',(209.81477762541,552.347556589211,-39.2297690928544)) ;
#72067=CARTESIAN_POINT('',(209.68977762541,552.347556589211,-39.2297690928544)) ;
#72068=CARTESIAN_POINT('Origin',(209.81477762541,552.347556589211,-39.2297690928544)) ;
#72069=CARTESIAN_POINT('Origin',(209.81477762541,552.347556589211,-39.2297690928544)) ;
#72070=CARTESIAN_POINT('Origin',(209.81477762541,552.347556589211,-39.2297690928544)) ;
#72071=CARTESIAN_POINT('Origin',(209.81477762541,548.488181589211,-39.2297690928544)) ;
#72072=CARTESIAN_POINT('',(209.68977762541,548.488181589211,-39.2297690928544)) ;
#72073=CARTESIAN_POINT('Origin',(207.75302762541,552.347556589211,-39.2297690928544)) ;
#72074=CARTESIAN_POINT('Origin',(210.51727762541,552.347556589211,-39.2297690928544)) ;
#72075=CARTESIAN_POINT('Origin',(212.118601772278,548.59755658921,-39.2297690928544)) ;
#72076=CARTESIAN_POINT('',(212.118601772278,548.47255658921,-39.2297690928544)) ;
#72077=CARTESIAN_POINT('Origin',(210.51727762541,548.59755658921,-39.2297690928544)) ;
#72078=CARTESIAN_POINT('Origin',(210.51727762541,548.488181589211,-39.2297690928544)) ;
#72079=CARTESIAN_POINT('Origin',(210.51727762541,548.59755658921,-39.2297690928544)) ;
#72080=CARTESIAN_POINT('Origin',(210.51727762541,552.347556589211,-39.2297690928544)) ;
#72081=CARTESIAN_POINT('Origin',(210.51727762541,548.59755658921,-39.2297690928544)) ;
#72082=CARTESIAN_POINT('Origin',(210.51727762541,552.347556589211,-39.2297690928544)) ;
#72083=CARTESIAN_POINT('Origin',(202.262277625412,560.482556589212,-39.8669650424525)) ;
#72084=CARTESIAN_POINT('Origin',(202.262277625412,560.482556589212,-39.4182700580611)) ;
#72085=CARTESIAN_POINT('Origin',(212.118601772279,558.097556589211,-39.2297700580611)) ;
#72086=CARTESIAN_POINT('',(201.559777625412,557.97255658921,-39.2297700580612)) ;
#72087=CARTESIAN_POINT('',(201.559777625412,558.097556589211,-39.3547700580611)) ;
#72088=CARTESIAN_POINT('Origin',(201.559777625412,558.097556589211,-39.2297700580612)) ;
#72089=CARTESIAN_POINT('',(212.11860177228,557.97255658921,-39.2297700580611)) ;
#72090=CARTESIAN_POINT('',(202.262277625412,558.09755658921,-39.3547700580611)) ;
#72091=CARTESIAN_POINT('Origin',(202.262277625412,558.097556589211,-39.2297700580612)) ;
#72092=CARTESIAN_POINT('',(212.118601772279,558.097556589211,-39.3547700580611)) ;
#72093=CARTESIAN_POINT('Origin',(202.262277625412,560.671056589212,-39.4182700580612)) ;
#72094=CARTESIAN_POINT('',(202.262277625412,560.671056589212,-39.3547700580612)) ;
#72095=CARTESIAN_POINT('Origin',(202.262277625412,560.671056589212,-39.4182700580612)) ;
#72096=CARTESIAN_POINT('Origin',(202.262277625412,560.671056589212,-39.2297700580612)) ;
#72097=CARTESIAN_POINT('Origin',(202.262277625412,557.988181589211,-39.2297700580612)) ;
#72098=CARTESIAN_POINT('',(202.262277625412,561.847556589211,-39.3547700580612)) ;
#72099=CARTESIAN_POINT('Origin',(202.262277625412,561.847556589211,-39.2297700580612)) ;
#72100=CARTESIAN_POINT('',(202.262277625412,557.988181589211,-39.3547700580611)) ;
#72101=CARTESIAN_POINT('Origin',(201.559777625412,560.671056589212,-39.4182700580612)) ;
#72102=CARTESIAN_POINT('',(201.559777625412,560.671056589212,-39.3547700580612)) ;
#72103=CARTESIAN_POINT('Origin',(201.559777625412,560.671056589212,-39.4182700580612)) ;
#72104=CARTESIAN_POINT('Origin',(201.559777625412,560.671056589212,-39.2297700580612)) ;
#72105=CARTESIAN_POINT('Origin',(202.262277625412,559.274056589212,-39.4182700580611)) ;
#72106=CARTESIAN_POINT('',(202.262277625412,559.337556589212,-39.4182700580611)) ;
#72107=CARTESIAN_POINT('',(202.262277625412,559.274056589212,-39.3547700580611)) ;
#72108=CARTESIAN_POINT('Origin',(202.262277625412,559.274056589212,-39.4182700580611)) ;
#72109=CARTESIAN_POINT('Origin',(202.262277625412,559.274056589212,-39.2297700580612)) ;
#72110=CARTESIAN_POINT('Origin',(202.262277625412,559.462556589212,-39.4182700580611)) ;
#72111=CARTESIAN_POINT('Origin',(202.262277625412,559.462556589212,-37.6444650424525)) ;
#72112=CARTESIAN_POINT('',(202.262277625412,559.337556589212,-37.6444650424525)) ;
#72113=CARTESIAN_POINT('Origin',(202.262277625412,557.988181589211,-39.2297700580612)) ;
#72114=CARTESIAN_POINT('Origin',(202.262277625412,558.09755658921,-39.2297700580612)) ;
#72115=CARTESIAN_POINT('',(202.262277625412,557.988181589211,-39.3547700580611)) ;
#72116=CARTESIAN_POINT('Origin',(201.559777625412,559.274056589212,-39.4182700580611)) ;
#72117=CARTESIAN_POINT('',(201.559777625412,559.274056589212,-39.3547700580611)) ;
#72118=CARTESIAN_POINT('Origin',(201.559777625412,559.274056589212,-39.4182700580611)) ;
#72119=CARTESIAN_POINT('Origin',(201.559777625412,559.274056589212,-39.2297700580612)) ;
#72120=CARTESIAN_POINT('Origin',(201.559777625412,557.988181589211,-39.2297700580612)) ;
#72121=CARTESIAN_POINT('Origin',(201.559777625412,558.097556589211,-39.2297700580612)) ;
#72122=CARTESIAN_POINT('',(201.559777625412,557.988181589211,-39.3547700580611)) ;
#72123=CARTESIAN_POINT('Origin',(219.024277625411,559.274056589212,-39.4182700580611)) ;
#72124=CARTESIAN_POINT('',(219.024277625411,559.274056589212,-39.3547700580611)) ;
#72125=CARTESIAN_POINT('',(219.024277625411,559.337556589212,-39.4182700580611)) ;
#72126=CARTESIAN_POINT('Origin',(201.559777625412,557.988181589211,-39.2297700580612)) ;
#72127=CARTESIAN_POINT('',(201.559777625412,561.847556589211,-39.3547700580611)) ;
#72128=CARTESIAN_POINT('Origin',(201.559777625412,561.847556589211,-39.2297700580612)) ;
#72129=CARTESIAN_POINT('',(201.559777625412,557.988181589211,-39.3547700580611)) ;
#72130=CARTESIAN_POINT('Origin',(218.198777625411,560.671056589212,-39.4182700580611)) ;
#72131=CARTESIAN_POINT('',(218.198777625411,560.671056589212,-39.3547700580611)) ;
#72132=CARTESIAN_POINT('Origin',(201.559777625412,558.097556589211,-39.2297700580612)) ;
#72133=CARTESIAN_POINT('Origin',(201.559777625412,558.097556589211,-39.2297700580612)) ;
#72134=CARTESIAN_POINT('Origin',(202.262277625412,558.09755658921,-39.2297700580612)) ;
#72135=CARTESIAN_POINT('Origin',(207.753027625412,561.847556589211,-39.2297700580612)) ;
#72136=CARTESIAN_POINT('Origin',(201.559777625412,561.847556589211,-39.2297700580612)) ;
#72137=CARTESIAN_POINT('',(207.753027625412,561.847556589211,-39.3547700580611)) ;
#72138=CARTESIAN_POINT('Origin',(202.262277625412,561.847556589211,-39.2297700580612)) ;
#72139=CARTESIAN_POINT('Origin',(201.559777625412,561.847556589211,-39.2297700580612)) ;
#72140=CARTESIAN_POINT('Origin',(201.559777625412,561.847556589211,-39.2297700580612)) ;
#72141=CARTESIAN_POINT('Origin',(202.262277625412,561.847556589211,-39.2297700580612)) ;
#72142=CARTESIAN_POINT('Origin',(219.849777625411,559.337556589212,-41.5221609920506)) ;
#72143=CARTESIAN_POINT('Origin',(218.198777625412,560.607556589211,-39.3547700580611)) ;
#72144=CARTESIAN_POINT('Origin',(218.198777625412,560.607556589211,-39.3547700580611)) ;
#72145=CARTESIAN_POINT('Origin',(218.198777625412,560.607556589211,-39.3547690928544)) ;
#72146=CARTESIAN_POINT('',(209.814777625412,561.847556589211,-39.3547690928544)) ;
#72147=CARTESIAN_POINT('',(209.814777625412,558.097556589211,-39.3547690928544)) ;
#72148=CARTESIAN_POINT('',(209.814777625412,557.988181589211,-39.3547690928544)) ;
#72149=CARTESIAN_POINT('',(210.517277625412,558.097556589211,-39.3547690928544)) ;
#72150=CARTESIAN_POINT('',(212.118601772279,558.097556589211,-39.3547690928544)) ;
#72151=CARTESIAN_POINT('',(210.517277625412,561.847556589211,-39.3547690928544)) ;
#72152=CARTESIAN_POINT('',(210.517277625412,557.988181589211,-39.3547690928544)) ;
#72153=CARTESIAN_POINT('',(207.753027625412,561.847556589211,-39.3547690928544)) ;
#72154=CARTESIAN_POINT('Origin',(209.814777625412,558.097556589211,-39.2297690928544)) ;
#72155=CARTESIAN_POINT('',(209.814777625412,557.97255658921,-39.2297690928544)) ;
#72156=CARTESIAN_POINT('Origin',(209.814777625412,558.097556589211,-39.2297690928544)) ;
#72157=CARTESIAN_POINT('',(209.689777625412,558.097556589211,-39.2297690928544)) ;
#72158=CARTESIAN_POINT('Origin',(209.814777625412,558.097556589211,-39.2297690928544)) ;
#72159=CARTESIAN_POINT('Origin',(209.814777625412,558.097556589211,-39.2297690928544)) ;
#72160=CARTESIAN_POINT('Origin',(209.814777625412,561.847556589211,-39.2297690928544)) ;
#72161=CARTESIAN_POINT('',(209.689777625412,561.847556589211,-39.2297690928544)) ;
#72162=CARTESIAN_POINT('Origin',(209.814777625412,561.847556589211,-39.2297690928544)) ;
#72163=CARTESIAN_POINT('Origin',(209.814777625412,561.847556589211,-39.2297690928544)) ;
#72164=CARTESIAN_POINT('Origin',(209.814777625412,561.847556589211,-39.2297690928544)) ;
#72165=CARTESIAN_POINT('Origin',(209.814777625412,557.988181589211,-39.2297690928544)) ;
#72166=CARTESIAN_POINT('',(209.689777625412,557.988181589211,-39.2297690928544)) ;
#72167=CARTESIAN_POINT('Origin',(207.753027625412,561.847556589211,-39.2297690928544)) ;
#72168=CARTESIAN_POINT('Origin',(210.517277625412,561.847556589211,-39.2297690928544)) ;
#72169=CARTESIAN_POINT('Origin',(212.118601772279,558.097556589211,-39.2297690928544)) ;
#72170=CARTESIAN_POINT('',(212.118601772279,557.97255658921,-39.2297690928544)) ;
#72171=CARTESIAN_POINT('Origin',(210.517277625412,558.097556589211,-39.2297690928544)) ;
#72172=CARTESIAN_POINT('Origin',(210.517277625412,557.988181589211,-39.2297690928544)) ;
#72173=CARTESIAN_POINT('Origin',(210.517277625412,558.097556589211,-39.2297690928544)) ;
#72174=CARTESIAN_POINT('Origin',(210.517277625412,561.847556589211,-39.2297690928544)) ;
#72175=CARTESIAN_POINT('Origin',(210.517277625412,558.097556589211,-39.2297690928544)) ;
#72176=CARTESIAN_POINT('Origin',(210.517277625412,561.847556589211,-39.2297690928544)) ;
#72177=CARTESIAN_POINT('Origin',(202.262277625413,569.982556589212,-39.8669650424525)) ;
#72178=CARTESIAN_POINT('Origin',(202.262277625413,569.982556589212,-39.4182700580611)) ;
#72179=CARTESIAN_POINT('Origin',(212.118601772281,567.59755658921,-39.2297700580611)) ;
#72180=CARTESIAN_POINT('',(201.559777625414,567.47255658921,-39.2297700580612)) ;
#72181=CARTESIAN_POINT('',(201.559777625414,567.59755658921,-39.3547700580611)) ;
#72182=CARTESIAN_POINT('Origin',(201.559777625414,567.59755658921,-39.2297700580612)) ;
#72183=CARTESIAN_POINT('',(212.118601772281,567.47255658921,-39.2297700580611)) ;
#72184=CARTESIAN_POINT('',(202.262277625413,567.59755658921,-39.3547700580611)) ;
#72185=CARTESIAN_POINT('Origin',(202.262277625413,567.59755658921,-39.2297700580612)) ;
#72186=CARTESIAN_POINT('',(212.118601772281,567.59755658921,-39.3547700580611)) ;
#72187=CARTESIAN_POINT('Origin',(202.262277625413,570.171056589212,-39.4182700580612)) ;
#72188=CARTESIAN_POINT('',(202.262277625413,570.171056589212,-39.3547700580612)) ;
#72189=CARTESIAN_POINT('Origin',(202.262277625413,570.171056589212,-39.4182700580612)) ;
#72190=CARTESIAN_POINT('Origin',(202.262277625413,570.171056589212,-39.2297700580612)) ;
#72191=CARTESIAN_POINT('Origin',(202.262277625413,567.488181589211,-39.2297700580612)) ;
#72192=CARTESIAN_POINT('',(202.262277625413,571.347556589211,-39.3547700580612)) ;
#72193=CARTESIAN_POINT('Origin',(202.262277625413,571.347556589211,-39.2297700580612)) ;
#72194=CARTESIAN_POINT('',(202.262277625413,567.488181589211,-39.3547700580611)) ;
#72195=CARTESIAN_POINT('Origin',(201.559777625414,570.171056589212,-39.4182700580612)) ;
#72196=CARTESIAN_POINT('',(201.559777625414,570.171056589212,-39.3547700580612)) ;
#72197=CARTESIAN_POINT('Origin',(201.559777625414,570.171056589212,-39.4182700580612)) ;
#72198=CARTESIAN_POINT('Origin',(201.559777625414,570.171056589212,-39.2297700580612)) ;
#72199=CARTESIAN_POINT('Origin',(202.262277625413,568.774056589212,-39.4182700580611)) ;
#72200=CARTESIAN_POINT('',(202.262277625413,568.837556589212,-39.4182700580611)) ;
#72201=CARTESIAN_POINT('',(202.262277625413,568.774056589212,-39.3547700580611)) ;
#72202=CARTESIAN_POINT('Origin',(202.262277625413,568.774056589212,-39.4182700580611)) ;
#72203=CARTESIAN_POINT('Origin',(202.262277625413,568.774056589212,-39.2297700580612)) ;
#72204=CARTESIAN_POINT('Origin',(202.262277625413,568.962556589212,-39.4182700580611)) ;
#72205=CARTESIAN_POINT('Origin',(202.262277625413,568.962556589212,-37.6444650424525)) ;
#72206=CARTESIAN_POINT('',(202.262277625413,568.837556589212,-37.6444650424525)) ;
#72207=CARTESIAN_POINT('Origin',(202.262277625413,567.488181589211,-39.2297700580612)) ;
#72208=CARTESIAN_POINT('Origin',(202.262277625413,567.59755658921,-39.2297700580612)) ;
#72209=CARTESIAN_POINT('',(202.262277625413,567.488181589211,-39.3547700580611)) ;
#72210=CARTESIAN_POINT('Origin',(201.559777625414,568.774056589212,-39.4182700580611)) ;
#72211=CARTESIAN_POINT('',(201.559777625414,568.774056589212,-39.3547700580611)) ;
#72212=CARTESIAN_POINT('Origin',(201.559777625414,568.774056589212,-39.4182700580611)) ;
#72213=CARTESIAN_POINT('Origin',(201.559777625414,568.774056589212,-39.2297700580612)) ;
#72214=CARTESIAN_POINT('Origin',(201.559777625414,567.488181589211,-39.2297700580612)) ;
#72215=CARTESIAN_POINT('Origin',(201.559777625414,567.59755658921,-39.2297700580612)) ;
#72216=CARTESIAN_POINT('',(201.559777625414,567.488181589211,-39.3547700580611)) ;
#72217=CARTESIAN_POINT('Origin',(219.024277625413,568.774056589212,-39.4182700580611)) ;
#72218=CARTESIAN_POINT('',(219.024277625413,568.774056589212,-39.3547700580611)) ;
#72219=CARTESIAN_POINT('',(219.024277625413,568.837556589212,-39.4182700580611)) ;
#72220=CARTESIAN_POINT('Origin',(201.559777625414,567.488181589211,-39.2297700580612)) ;
#72221=CARTESIAN_POINT('',(201.559777625414,571.347556589211,-39.3547700580611)) ;
#72222=CARTESIAN_POINT('Origin',(201.559777625414,571.347556589211,-39.2297700580612)) ;
#72223=CARTESIAN_POINT('',(201.559777625414,567.488181589211,-39.3547700580611)) ;
#72224=CARTESIAN_POINT('Origin',(218.198777625413,570.171056589212,-39.4182700580611)) ;
#72225=CARTESIAN_POINT('',(218.198777625413,570.171056589212,-39.3547700580611)) ;
#72226=CARTESIAN_POINT('Origin',(201.559777625414,567.59755658921,-39.2297700580612)) ;
#72227=CARTESIAN_POINT('Origin',(201.559777625414,567.59755658921,-39.2297700580612)) ;
#72228=CARTESIAN_POINT('Origin',(202.262277625413,567.59755658921,-39.2297700580612)) ;
#72229=CARTESIAN_POINT('Origin',(207.753027625413,571.347556589211,-39.2297700580612)) ;
#72230=CARTESIAN_POINT('Origin',(201.559777625414,571.347556589211,-39.2297700580612)) ;
#72231=CARTESIAN_POINT('',(207.753027625413,571.347556589211,-39.3547700580611)) ;
#72232=CARTESIAN_POINT('Origin',(202.262277625413,571.347556589211,-39.2297700580612)) ;
#72233=CARTESIAN_POINT('Origin',(201.559777625414,571.347556589211,-39.2297700580612)) ;
#72234=CARTESIAN_POINT('Origin',(201.559777625414,571.347556589211,-39.2297700580612)) ;
#72235=CARTESIAN_POINT('Origin',(202.262277625413,571.347556589211,-39.2297700580612)) ;
#72236=CARTESIAN_POINT('Origin',(219.849777625412,568.837556589212,-41.5221609920506)) ;
#72237=CARTESIAN_POINT('Origin',(218.198777625413,570.107556589211,-39.3547700580611)) ;
#72238=CARTESIAN_POINT('Origin',(218.198777625413,570.107556589211,-39.3547700580611)) ;
#72239=CARTESIAN_POINT('Origin',(218.198777625413,570.107556589211,-39.3547690928544)) ;
#72240=CARTESIAN_POINT('',(209.814777625413,571.347556589211,-39.3547690928544)) ;
#72241=CARTESIAN_POINT('',(209.814777625413,567.59755658921,-39.3547690928544)) ;
#72242=CARTESIAN_POINT('',(209.814777625413,567.488181589211,-39.3547690928544)) ;
#72243=CARTESIAN_POINT('',(210.517277625414,567.59755658921,-39.3547690928544)) ;
#72244=CARTESIAN_POINT('',(212.118601772281,567.59755658921,-39.3547690928544)) ;
#72245=CARTESIAN_POINT('',(210.517277625414,571.347556589211,-39.3547690928544)) ;
#72246=CARTESIAN_POINT('',(210.517277625414,567.488181589211,-39.3547690928544)) ;
#72247=CARTESIAN_POINT('',(207.753027625413,571.347556589211,-39.3547690928544)) ;
#72248=CARTESIAN_POINT('Origin',(209.814777625413,567.59755658921,-39.2297690928544)) ;
#72249=CARTESIAN_POINT('',(209.814777625413,567.47255658921,-39.2297690928544)) ;
#72250=CARTESIAN_POINT('Origin',(209.814777625413,567.59755658921,-39.2297690928544)) ;
#72251=CARTESIAN_POINT('',(209.689777625413,567.59755658921,-39.2297690928544)) ;
#72252=CARTESIAN_POINT('Origin',(209.814777625413,567.59755658921,-39.2297690928544)) ;
#72253=CARTESIAN_POINT('Origin',(209.814777625413,567.59755658921,-39.2297690928544)) ;
#72254=CARTESIAN_POINT('Origin',(209.814777625413,571.347556589211,-39.2297690928544)) ;
#72255=CARTESIAN_POINT('',(209.689777625413,571.347556589211,-39.2297690928544)) ;
#72256=CARTESIAN_POINT('Origin',(209.814777625413,571.347556589211,-39.2297690928544)) ;
#72257=CARTESIAN_POINT('Origin',(209.814777625413,571.347556589211,-39.2297690928544)) ;
#72258=CARTESIAN_POINT('Origin',(209.814777625413,571.347556589211,-39.2297690928544)) ;
#72259=CARTESIAN_POINT('Origin',(209.814777625413,567.488181589211,-39.2297690928544)) ;
#72260=CARTESIAN_POINT('',(209.689777625413,567.488181589211,-39.2297690928544)) ;
#72261=CARTESIAN_POINT('Origin',(207.753027625413,571.347556589211,-39.2297690928544)) ;
#72262=CARTESIAN_POINT('Origin',(210.517277625414,571.347556589211,-39.2297690928544)) ;
#72263=CARTESIAN_POINT('Origin',(212.118601772281,567.59755658921,-39.2297690928544)) ;
#72264=CARTESIAN_POINT('',(212.118601772281,567.47255658921,-39.2297690928544)) ;
#72265=CARTESIAN_POINT('Origin',(210.517277625414,567.59755658921,-39.2297690928544)) ;
#72266=CARTESIAN_POINT('Origin',(210.517277625414,567.488181589211,-39.2297690928544)) ;
#72267=CARTESIAN_POINT('Origin',(210.517277625414,567.59755658921,-39.2297690928544)) ;
#72268=CARTESIAN_POINT('Origin',(210.517277625414,571.347556589211,-39.2297690928544)) ;
#72269=CARTESIAN_POINT('Origin',(210.517277625414,567.59755658921,-39.2297690928544)) ;
#72270=CARTESIAN_POINT('Origin',(210.517277625414,571.347556589211,-39.2297690928544)) ;
#72271=CARTESIAN_POINT('Origin',(202.262277625415,579.482556589212,-39.8669650424525)) ;
#72272=CARTESIAN_POINT('Origin',(202.262277625415,579.482556589212,-39.4182700580611)) ;
#72273=CARTESIAN_POINT('Origin',(212.118601772283,577.097556589211,-39.2297700580611)) ;
#72274=CARTESIAN_POINT('',(201.559777625416,576.972556589211,-39.2297700580612)) ;
#72275=CARTESIAN_POINT('',(201.559777625415,577.097556589211,-39.3547700580611)) ;
#72276=CARTESIAN_POINT('Origin',(201.559777625415,577.097556589211,-39.2297700580612)) ;
#72277=CARTESIAN_POINT('',(212.118601772283,576.972556589211,-39.2297700580611)) ;
#72278=CARTESIAN_POINT('',(202.262277625415,577.097556589211,-39.3547700580611)) ;
#72279=CARTESIAN_POINT('Origin',(202.262277625415,577.097556589211,-39.2297700580612)) ;
#72280=CARTESIAN_POINT('',(212.118601772283,577.097556589211,-39.3547700580611)) ;
#72281=CARTESIAN_POINT('Origin',(202.262277625415,579.671056589212,-39.4182700580612)) ;
#72282=CARTESIAN_POINT('',(202.262277625415,579.671056589212,-39.3547700580612)) ;
#72283=CARTESIAN_POINT('Origin',(202.262277625415,579.671056589212,-39.4182700580612)) ;
#72284=CARTESIAN_POINT('Origin',(202.262277625415,579.671056589212,-39.2297700580612)) ;
#72285=CARTESIAN_POINT('Origin',(202.262277625415,576.988181589211,-39.2297700580612)) ;
#72286=CARTESIAN_POINT('',(202.262277625415,580.847556589211,-39.3547700580612)) ;
#72287=CARTESIAN_POINT('Origin',(202.262277625415,580.847556589211,-39.2297700580612)) ;
#72288=CARTESIAN_POINT('',(202.262277625415,576.988181589211,-39.3547700580611)) ;
#72289=CARTESIAN_POINT('Origin',(201.559777625415,579.671056589212,-39.4182700580612)) ;
#72290=CARTESIAN_POINT('',(201.559777625415,579.671056589212,-39.3547700580612)) ;
#72291=CARTESIAN_POINT('Origin',(201.559777625415,579.671056589212,-39.4182700580612)) ;
#72292=CARTESIAN_POINT('Origin',(201.559777625415,579.671056589212,-39.2297700580612)) ;
#72293=CARTESIAN_POINT('Origin',(202.262277625415,578.274056589212,-39.4182700580611)) ;
#72294=CARTESIAN_POINT('',(202.262277625415,578.337556589212,-39.4182700580611)) ;
#72295=CARTESIAN_POINT('',(202.262277625415,578.274056589212,-39.3547700580611)) ;
#72296=CARTESIAN_POINT('Origin',(202.262277625415,578.274056589212,-39.4182700580611)) ;
#72297=CARTESIAN_POINT('Origin',(202.262277625415,578.274056589212,-39.2297700580612)) ;
#72298=CARTESIAN_POINT('Origin',(202.262277625415,578.462556589212,-39.4182700580611)) ;
#72299=CARTESIAN_POINT('Origin',(202.262277625415,578.462556589212,-37.6444650424525)) ;
#72300=CARTESIAN_POINT('',(202.262277625415,578.337556589212,-37.6444650424525)) ;
#72301=CARTESIAN_POINT('Origin',(202.262277625415,576.988181589211,-39.2297700580612)) ;
#72302=CARTESIAN_POINT('Origin',(202.262277625415,577.097556589211,-39.2297700580612)) ;
#72303=CARTESIAN_POINT('',(202.262277625415,576.988181589211,-39.3547700580611)) ;
#72304=CARTESIAN_POINT('Origin',(201.559777625415,578.274056589212,-39.4182700580611)) ;
#72305=CARTESIAN_POINT('',(201.559777625415,578.274056589212,-39.3547700580611)) ;
#72306=CARTESIAN_POINT('Origin',(201.559777625415,578.274056589212,-39.4182700580611)) ;
#72307=CARTESIAN_POINT('Origin',(201.559777625415,578.274056589212,-39.2297700580612)) ;
#72308=CARTESIAN_POINT('Origin',(201.559777625415,576.988181589211,-39.2297700580612)) ;
#72309=CARTESIAN_POINT('Origin',(201.559777625415,577.097556589211,-39.2297700580612)) ;
#72310=CARTESIAN_POINT('',(201.559777625415,576.988181589211,-39.3547700580611)) ;
#72311=CARTESIAN_POINT('Origin',(219.024277625414,578.274056589212,-39.4182700580611)) ;
#72312=CARTESIAN_POINT('',(219.024277625414,578.274056589212,-39.3547700580611)) ;
#72313=CARTESIAN_POINT('',(219.024277625414,578.337556589212,-39.4182700580611)) ;
#72314=CARTESIAN_POINT('Origin',(201.559777625415,576.988181589211,-39.2297700580612)) ;
#72315=CARTESIAN_POINT('',(201.559777625415,580.847556589211,-39.3547700580611)) ;
#72316=CARTESIAN_POINT('Origin',(201.559777625415,580.847556589211,-39.2297700580612)) ;
#72317=CARTESIAN_POINT('',(201.559777625415,576.988181589211,-39.3547700580611)) ;
#72318=CARTESIAN_POINT('Origin',(218.198777625414,579.671056589212,-39.4182700580611)) ;
#72319=CARTESIAN_POINT('',(218.198777625414,579.671056589212,-39.3547700580611)) ;
#72320=CARTESIAN_POINT('Origin',(201.559777625415,577.097556589211,-39.2297700580612)) ;
#72321=CARTESIAN_POINT('Origin',(201.559777625415,577.097556589211,-39.2297700580612)) ;
#72322=CARTESIAN_POINT('Origin',(202.262277625415,577.097556589211,-39.2297700580612)) ;
#72323=CARTESIAN_POINT('Origin',(207.753027625415,580.847556589211,-39.2297700580612)) ;
#72324=CARTESIAN_POINT('Origin',(201.559777625415,580.847556589211,-39.2297700580612)) ;
#72325=CARTESIAN_POINT('',(207.753027625415,580.847556589211,-39.3547700580611)) ;
#72326=CARTESIAN_POINT('Origin',(202.262277625415,580.847556589211,-39.2297700580612)) ;
#72327=CARTESIAN_POINT('Origin',(201.559777625415,580.847556589211,-39.2297700580612)) ;
#72328=CARTESIAN_POINT('Origin',(201.559777625415,580.847556589211,-39.2297700580612)) ;
#72329=CARTESIAN_POINT('Origin',(202.262277625415,580.847556589211,-39.2297700580612)) ;
#72330=CARTESIAN_POINT('Origin',(219.849777625414,578.337556589212,-41.5221609920506)) ;
#72331=CARTESIAN_POINT('Origin',(218.198777625415,579.607556589211,-39.3547700580611)) ;
#72332=CARTESIAN_POINT('Origin',(218.198777625415,579.607556589211,-39.3547700580611)) ;
#72333=CARTESIAN_POINT('Origin',(218.198777625415,579.607556589211,-39.3547690928544)) ;
#72334=CARTESIAN_POINT('',(209.814777625415,580.847556589211,-39.3547690928544)) ;
#72335=CARTESIAN_POINT('',(209.814777625415,577.097556589211,-39.3547690928544)) ;
#72336=CARTESIAN_POINT('',(209.814777625415,576.988181589211,-39.3547690928544)) ;
#72337=CARTESIAN_POINT('',(210.517277625416,577.097556589211,-39.3547690928544)) ;
#72338=CARTESIAN_POINT('',(212.118601772283,577.097556589211,-39.3547690928544)) ;
#72339=CARTESIAN_POINT('',(210.517277625416,580.847556589211,-39.3547690928544)) ;
#72340=CARTESIAN_POINT('',(210.517277625416,576.988181589211,-39.3547690928544)) ;
#72341=CARTESIAN_POINT('',(207.753027625415,580.847556589211,-39.3547690928544)) ;
#72342=CARTESIAN_POINT('Origin',(209.814777625415,577.097556589211,-39.2297690928544)) ;
#72343=CARTESIAN_POINT('',(209.814777625415,576.972556589211,-39.2297690928544)) ;
#72344=CARTESIAN_POINT('Origin',(209.814777625415,577.097556589211,-39.2297690928544)) ;
#72345=CARTESIAN_POINT('',(209.689777625415,577.097556589211,-39.2297690928544)) ;
#72346=CARTESIAN_POINT('Origin',(209.814777625415,577.097556589211,-39.2297690928544)) ;
#72347=CARTESIAN_POINT('Origin',(209.814777625415,577.097556589211,-39.2297690928544)) ;
#72348=CARTESIAN_POINT('Origin',(209.814777625415,580.847556589211,-39.2297690928544)) ;
#72349=CARTESIAN_POINT('',(209.689777625415,580.847556589211,-39.2297690928544)) ;
#72350=CARTESIAN_POINT('Origin',(209.814777625415,580.847556589211,-39.2297690928544)) ;
#72351=CARTESIAN_POINT('Origin',(209.814777625415,580.847556589211,-39.2297690928544)) ;
#72352=CARTESIAN_POINT('Origin',(209.814777625415,580.847556589211,-39.2297690928544)) ;
#72353=CARTESIAN_POINT('Origin',(209.814777625415,576.988181589211,-39.2297690928544)) ;
#72354=CARTESIAN_POINT('',(209.689777625415,576.988181589211,-39.2297690928544)) ;
#72355=CARTESIAN_POINT('Origin',(207.753027625415,580.847556589211,-39.2297690928544)) ;
#72356=CARTESIAN_POINT('Origin',(210.517277625416,580.847556589211,-39.2297690928544)) ;
#72357=CARTESIAN_POINT('Origin',(212.118601772283,577.097556589211,-39.2297690928544)) ;
#72358=CARTESIAN_POINT('',(212.118601772283,576.972556589211,-39.2297690928544)) ;
#72359=CARTESIAN_POINT('Origin',(210.517277625416,577.097556589211,-39.2297690928544)) ;
#72360=CARTESIAN_POINT('Origin',(210.517277625416,576.988181589211,-39.2297690928544)) ;
#72361=CARTESIAN_POINT('Origin',(210.517277625416,577.097556589211,-39.2297690928544)) ;
#72362=CARTESIAN_POINT('Origin',(210.517277625416,580.847556589211,-39.2297690928544)) ;
#72363=CARTESIAN_POINT('Origin',(210.517277625416,577.097556589211,-39.2297690928544)) ;
#72364=CARTESIAN_POINT('Origin',(210.517277625416,580.847556589211,-39.2297690928544)) ;
#72365=CARTESIAN_POINT('Origin',(202.262277625416,588.982556589212,-39.8669650424525)) ;
#72366=CARTESIAN_POINT('Origin',(202.262277625416,588.982556589212,-39.4182700580611)) ;
#72367=CARTESIAN_POINT('Origin',(212.118601772284,586.597556589211,-39.2297700580611)) ;
#72368=CARTESIAN_POINT('',(201.559777625417,586.472556589211,-39.2297700580612)) ;
#72369=CARTESIAN_POINT('',(201.559777625417,586.597556589211,-39.3547700580611)) ;
#72370=CARTESIAN_POINT('Origin',(201.559777625417,586.597556589211,-39.2297700580612)) ;
#72371=CARTESIAN_POINT('',(212.118601772284,586.472556589211,-39.2297700580611)) ;
#72372=CARTESIAN_POINT('',(202.262277625417,586.597556589211,-39.3547700580611)) ;
#72373=CARTESIAN_POINT('Origin',(202.262277625417,586.597556589211,-39.2297700580612)) ;
#72374=CARTESIAN_POINT('',(212.118601772284,586.597556589211,-39.3547700580611)) ;
#72375=CARTESIAN_POINT('Origin',(202.262277625416,589.171056589212,-39.4182700580612)) ;
#72376=CARTESIAN_POINT('',(202.262277625417,589.171056589212,-39.3547700580612)) ;
#72377=CARTESIAN_POINT('Origin',(202.262277625417,589.171056589212,-39.4182700580612)) ;
#72378=CARTESIAN_POINT('Origin',(202.262277625417,589.171056589212,-39.2297700580612)) ;
#72379=CARTESIAN_POINT('Origin',(202.262277625417,586.488181589211,-39.2297700580612)) ;
#72380=CARTESIAN_POINT('',(202.262277625417,590.347556589211,-39.3547700580612)) ;
#72381=CARTESIAN_POINT('Origin',(202.262277625417,590.347556589211,-39.2297700580612)) ;
#72382=CARTESIAN_POINT('',(202.262277625417,586.488181589211,-39.3547700580611)) ;
#72383=CARTESIAN_POINT('Origin',(201.559777625417,589.171056589212,-39.4182700580612)) ;
#72384=CARTESIAN_POINT('',(201.559777625417,589.171056589212,-39.3547700580612)) ;
#72385=CARTESIAN_POINT('Origin',(201.559777625417,589.171056589212,-39.4182700580612)) ;
#72386=CARTESIAN_POINT('Origin',(201.559777625417,589.171056589212,-39.2297700580612)) ;
#72387=CARTESIAN_POINT('Origin',(202.262277625417,587.774056589212,-39.4182700580611)) ;
#72388=CARTESIAN_POINT('',(202.262277625417,587.837556589212,-39.4182700580611)) ;
#72389=CARTESIAN_POINT('',(202.262277625417,587.774056589212,-39.3547700580611)) ;
#72390=CARTESIAN_POINT('Origin',(202.262277625417,587.774056589212,-39.4182700580611)) ;
#72391=CARTESIAN_POINT('Origin',(202.262277625417,587.774056589212,-39.2297700580612)) ;
#72392=CARTESIAN_POINT('Origin',(202.262277625417,587.962556589212,-39.4182700580611)) ;
#72393=CARTESIAN_POINT('Origin',(202.262277625417,587.962556589212,-37.6444650424525)) ;
#72394=CARTESIAN_POINT('',(202.262277625417,587.837556589212,-37.6444650424525)) ;
#72395=CARTESIAN_POINT('Origin',(202.262277625417,586.488181589211,-39.2297700580612)) ;
#72396=CARTESIAN_POINT('Origin',(202.262277625417,586.597556589211,-39.2297700580612)) ;
#72397=CARTESIAN_POINT('',(202.262277625417,586.488181589211,-39.3547700580611)) ;
#72398=CARTESIAN_POINT('Origin',(201.559777625417,587.774056589212,-39.4182700580611)) ;
#72399=CARTESIAN_POINT('',(201.559777625417,587.774056589212,-39.3547700580611)) ;
#72400=CARTESIAN_POINT('Origin',(201.559777625417,587.774056589212,-39.4182700580611)) ;
#72401=CARTESIAN_POINT('Origin',(201.559777625417,587.774056589212,-39.2297700580612)) ;
#72402=CARTESIAN_POINT('Origin',(201.559777625417,586.488181589211,-39.2297700580612)) ;
#72403=CARTESIAN_POINT('Origin',(201.559777625417,586.597556589211,-39.2297700580612)) ;
#72404=CARTESIAN_POINT('',(201.559777625417,586.488181589211,-39.3547700580611)) ;
#72405=CARTESIAN_POINT('Origin',(219.024277625416,587.774056589212,-39.4182700580611)) ;
#72406=CARTESIAN_POINT('',(219.024277625416,587.774056589212,-39.3547700580611)) ;
#72407=CARTESIAN_POINT('',(219.024277625416,587.837556589212,-39.4182700580611)) ;
#72408=CARTESIAN_POINT('Origin',(201.559777625417,586.488181589211,-39.2297700580612)) ;
#72409=CARTESIAN_POINT('',(201.559777625417,590.347556589211,-39.3547700580611)) ;
#72410=CARTESIAN_POINT('Origin',(201.559777625417,590.347556589211,-39.2297700580612)) ;
#72411=CARTESIAN_POINT('',(201.559777625417,586.488181589211,-39.3547700580611)) ;
#72412=CARTESIAN_POINT('Origin',(218.198777625416,589.171056589212,-39.4182700580611)) ;
#72413=CARTESIAN_POINT('',(218.198777625416,589.171056589212,-39.3547700580611)) ;
#72414=CARTESIAN_POINT('Origin',(201.559777625417,586.597556589211,-39.2297700580612)) ;
#72415=CARTESIAN_POINT('Origin',(201.559777625417,586.597556589211,-39.2297700580612)) ;
#72416=CARTESIAN_POINT('Origin',(202.262277625417,586.597556589211,-39.2297700580612)) ;
#72417=CARTESIAN_POINT('Origin',(207.753027625417,590.347556589211,-39.2297700580612)) ;
#72418=CARTESIAN_POINT('Origin',(201.559777625417,590.347556589211,-39.2297700580612)) ;
#72419=CARTESIAN_POINT('',(207.753027625417,590.347556589211,-39.3547700580611)) ;
#72420=CARTESIAN_POINT('Origin',(202.262277625417,590.347556589211,-39.2297700580612)) ;
#72421=CARTESIAN_POINT('Origin',(201.559777625417,590.347556589211,-39.2297700580612)) ;
#72422=CARTESIAN_POINT('Origin',(201.559777625417,590.347556589211,-39.2297700580612)) ;
#72423=CARTESIAN_POINT('Origin',(202.262277625417,590.347556589211,-39.2297700580612)) ;
#72424=CARTESIAN_POINT('Origin',(219.849777625416,587.837556589212,-41.5221609920506)) ;
#72425=CARTESIAN_POINT('Origin',(218.198777625417,589.107556589211,-39.3547700580611)) ;
#72426=CARTESIAN_POINT('Origin',(218.198777625417,589.107556589211,-39.3547700580611)) ;
#72427=CARTESIAN_POINT('Origin',(218.198777625417,589.107556589211,-39.3547690928544)) ;
#72428=CARTESIAN_POINT('',(209.814777625417,590.347556589211,-39.3547690928544)) ;
#72429=CARTESIAN_POINT('',(209.814777625417,586.597556589211,-39.3547690928544)) ;
#72430=CARTESIAN_POINT('',(209.814777625417,586.488181589211,-39.3547690928544)) ;
#72431=CARTESIAN_POINT('',(210.517277625417,586.597556589211,-39.3547690928544)) ;
#72432=CARTESIAN_POINT('',(212.118601772284,586.597556589211,-39.3547690928544)) ;
#72433=CARTESIAN_POINT('',(210.517277625417,590.347556589211,-39.3547690928544)) ;
#72434=CARTESIAN_POINT('',(210.517277625417,586.488181589211,-39.3547690928544)) ;
#72435=CARTESIAN_POINT('',(207.753027625417,590.347556589211,-39.3547690928544)) ;
#72436=CARTESIAN_POINT('Origin',(209.814777625417,586.597556589211,-39.2297690928544)) ;
#72437=CARTESIAN_POINT('',(209.814777625417,586.472556589211,-39.2297690928544)) ;
#72438=CARTESIAN_POINT('Origin',(209.814777625417,586.597556589211,-39.2297690928544)) ;
#72439=CARTESIAN_POINT('',(209.689777625417,586.597556589211,-39.2297690928544)) ;
#72440=CARTESIAN_POINT('Origin',(209.814777625417,586.597556589211,-39.2297690928544)) ;
#72441=CARTESIAN_POINT('Origin',(209.814777625417,586.597556589211,-39.2297690928544)) ;
#72442=CARTESIAN_POINT('Origin',(209.814777625417,590.347556589211,-39.2297690928544)) ;
#72443=CARTESIAN_POINT('',(209.689777625417,590.347556589211,-39.2297690928544)) ;
#72444=CARTESIAN_POINT('Origin',(209.814777625417,590.347556589211,-39.2297690928544)) ;
#72445=CARTESIAN_POINT('Origin',(209.814777625417,590.347556589211,-39.2297690928544)) ;
#72446=CARTESIAN_POINT('Origin',(209.814777625417,590.347556589211,-39.2297690928544)) ;
#72447=CARTESIAN_POINT('Origin',(209.814777625417,586.488181589211,-39.2297690928544)) ;
#72448=CARTESIAN_POINT('',(209.689777625417,586.488181589211,-39.2297690928544)) ;
#72449=CARTESIAN_POINT('Origin',(207.753027625417,590.347556589211,-39.2297690928544)) ;
#72450=CARTESIAN_POINT('Origin',(210.517277625417,590.347556589211,-39.2297690928544)) ;
#72451=CARTESIAN_POINT('Origin',(212.118601772284,586.597556589211,-39.2297690928544)) ;
#72452=CARTESIAN_POINT('',(212.118601772284,586.472556589211,-39.2297690928544)) ;
#72453=CARTESIAN_POINT('Origin',(210.517277625417,586.597556589211,-39.2297690928544)) ;
#72454=CARTESIAN_POINT('Origin',(210.517277625417,586.488181589211,-39.2297690928544)) ;
#72455=CARTESIAN_POINT('Origin',(210.517277625417,586.597556589211,-39.2297690928544)) ;
#72456=CARTESIAN_POINT('Origin',(210.517277625417,590.347556589211,-39.2297690928544)) ;
#72457=CARTESIAN_POINT('Origin',(210.517277625417,586.597556589211,-39.2297690928544)) ;
#72458=CARTESIAN_POINT('Origin',(210.517277625417,590.347556589211,-39.2297690928544)) ;
#72459=CARTESIAN_POINT('Origin',(202.262277625418,598.482556589212,-39.8669650424525)) ;
#72460=CARTESIAN_POINT('Origin',(202.262277625418,598.482556589212,-39.4182700580611)) ;
#72461=CARTESIAN_POINT('Origin',(212.118601772286,596.097556589211,-39.2297700580611)) ;
#72462=CARTESIAN_POINT('',(201.559777625419,595.972556589211,-39.2297700580612)) ;
#72463=CARTESIAN_POINT('',(201.559777625419,596.097556589211,-39.3547700580611)) ;
#72464=CARTESIAN_POINT('Origin',(201.559777625419,596.097556589211,-39.2297700580612)) ;
#72465=CARTESIAN_POINT('',(212.118601772286,595.972556589211,-39.2297700580611)) ;
#72466=CARTESIAN_POINT('',(202.262277625418,596.097556589211,-39.3547700580611)) ;
#72467=CARTESIAN_POINT('Origin',(202.262277625418,596.097556589211,-39.2297700580612)) ;
#72468=CARTESIAN_POINT('',(212.118601772286,596.097556589211,-39.3547700580611)) ;
#72469=CARTESIAN_POINT('Origin',(202.262277625418,598.671056589212,-39.4182700580612)) ;
#72470=CARTESIAN_POINT('',(202.262277625418,598.671056589212,-39.3547700580612)) ;
#72471=CARTESIAN_POINT('Origin',(202.262277625418,598.671056589212,-39.4182700580612)) ;
#72472=CARTESIAN_POINT('Origin',(202.262277625418,598.671056589212,-39.2297700580612)) ;
#72473=CARTESIAN_POINT('Origin',(202.262277625418,595.988181589211,-39.2297700580612)) ;
#72474=CARTESIAN_POINT('',(202.262277625418,599.847556589211,-39.3547700580612)) ;
#72475=CARTESIAN_POINT('Origin',(202.262277625418,599.847556589211,-39.2297700580612)) ;
#72476=CARTESIAN_POINT('',(202.262277625418,595.988181589211,-39.3547700580611)) ;
#72477=CARTESIAN_POINT('Origin',(201.559777625419,598.671056589212,-39.4182700580612)) ;
#72478=CARTESIAN_POINT('',(201.559777625419,598.671056589212,-39.3547700580612)) ;
#72479=CARTESIAN_POINT('Origin',(201.559777625419,598.671056589212,-39.4182700580612)) ;
#72480=CARTESIAN_POINT('Origin',(201.559777625419,598.671056589212,-39.2297700580612)) ;
#72481=CARTESIAN_POINT('Origin',(202.262277625418,597.274056589212,-39.4182700580611)) ;
#72482=CARTESIAN_POINT('',(202.262277625418,597.337556589212,-39.4182700580611)) ;
#72483=CARTESIAN_POINT('',(202.262277625418,597.274056589212,-39.3547700580611)) ;
#72484=CARTESIAN_POINT('Origin',(202.262277625418,597.274056589212,-39.4182700580611)) ;
#72485=CARTESIAN_POINT('Origin',(202.262277625418,597.274056589212,-39.2297700580612)) ;
#72486=CARTESIAN_POINT('Origin',(202.262277625418,597.462556589212,-39.4182700580611)) ;
#72487=CARTESIAN_POINT('Origin',(202.262277625418,597.462556589212,-37.6444650424525)) ;
#72488=CARTESIAN_POINT('',(202.262277625418,597.337556589212,-37.6444650424525)) ;
#72489=CARTESIAN_POINT('Origin',(202.262277625418,595.988181589211,-39.2297700580612)) ;
#72490=CARTESIAN_POINT('Origin',(202.262277625418,596.097556589211,-39.2297700580612)) ;
#72491=CARTESIAN_POINT('',(202.262277625418,595.988181589211,-39.3547700580611)) ;
#72492=CARTESIAN_POINT('Origin',(201.559777625419,597.274056589212,-39.4182700580611)) ;
#72493=CARTESIAN_POINT('',(201.559777625419,597.274056589212,-39.3547700580611)) ;
#72494=CARTESIAN_POINT('Origin',(201.559777625419,597.274056589212,-39.4182700580611)) ;
#72495=CARTESIAN_POINT('Origin',(201.559777625419,597.274056589212,-39.2297700580612)) ;
#72496=CARTESIAN_POINT('Origin',(201.559777625419,595.988181589211,-39.2297700580612)) ;
#72497=CARTESIAN_POINT('Origin',(201.559777625419,596.097556589211,-39.2297700580612)) ;
#72498=CARTESIAN_POINT('',(201.559777625419,595.988181589211,-39.3547700580611)) ;
#72499=CARTESIAN_POINT('Origin',(219.024277625418,597.274056589212,-39.4182700580611)) ;
#72500=CARTESIAN_POINT('',(219.024277625418,597.274056589212,-39.3547700580611)) ;
#72501=CARTESIAN_POINT('',(219.024277625418,597.337556589212,-39.4182700580611)) ;
#72502=CARTESIAN_POINT('Origin',(201.559777625419,595.988181589211,-39.2297700580612)) ;
#72503=CARTESIAN_POINT('',(201.559777625419,599.847556589211,-39.3547700580611)) ;
#72504=CARTESIAN_POINT('Origin',(201.559777625419,599.847556589211,-39.2297700580612)) ;
#72505=CARTESIAN_POINT('',(201.559777625419,595.988181589211,-39.3547700580611)) ;
#72506=CARTESIAN_POINT('Origin',(218.198777625418,598.671056589212,-39.4182700580611)) ;
#72507=CARTESIAN_POINT('',(218.198777625418,598.671056589212,-39.3547700580611)) ;
#72508=CARTESIAN_POINT('Origin',(201.559777625419,596.097556589211,-39.2297700580612)) ;
#72509=CARTESIAN_POINT('Origin',(201.559777625419,596.097556589211,-39.2297700580612)) ;
#72510=CARTESIAN_POINT('Origin',(202.262277625418,596.097556589211,-39.2297700580612)) ;
#72511=CARTESIAN_POINT('Origin',(207.753027625418,599.847556589211,-39.2297700580612)) ;
#72512=CARTESIAN_POINT('Origin',(201.559777625419,599.847556589211,-39.2297700580612)) ;
#72513=CARTESIAN_POINT('',(207.753027625418,599.847556589211,-39.3547700580611)) ;
#72514=CARTESIAN_POINT('Origin',(202.262277625418,599.847556589211,-39.2297700580612)) ;
#72515=CARTESIAN_POINT('Origin',(201.559777625419,599.847556589211,-39.2297700580612)) ;
#72516=CARTESIAN_POINT('Origin',(201.559777625419,599.847556589211,-39.2297700580612)) ;
#72517=CARTESIAN_POINT('Origin',(202.262277625418,599.847556589211,-39.2297700580612)) ;
#72518=CARTESIAN_POINT('Origin',(219.849777625417,597.337556589212,-41.5221609920506)) ;
#72519=CARTESIAN_POINT('Origin',(218.198777625418,598.607556589211,-39.3547700580611)) ;
#72520=CARTESIAN_POINT('Origin',(218.198777625418,598.607556589211,-39.3547700580611)) ;
#72521=CARTESIAN_POINT('Origin',(218.198777625418,598.607556589211,-39.3547690928544)) ;
#72522=CARTESIAN_POINT('',(209.814777625418,599.847556589211,-39.3547690928544)) ;
#72523=CARTESIAN_POINT('',(209.814777625418,596.097556589211,-39.3547690928544)) ;
#72524=CARTESIAN_POINT('',(209.814777625418,595.988181589211,-39.3547690928544)) ;
#72525=CARTESIAN_POINT('',(210.517277625419,596.097556589211,-39.3547690928544)) ;
#72526=CARTESIAN_POINT('',(212.118601772286,596.097556589211,-39.3547690928544)) ;
#72527=CARTESIAN_POINT('',(210.517277625419,599.847556589211,-39.3547690928544)) ;
#72528=CARTESIAN_POINT('',(210.517277625419,595.988181589211,-39.3547690928544)) ;
#72529=CARTESIAN_POINT('',(207.753027625418,599.847556589211,-39.3547690928544)) ;
#72530=CARTESIAN_POINT('Origin',(209.814777625418,596.097556589211,-39.2297690928544)) ;
#72531=CARTESIAN_POINT('',(209.814777625418,595.972556589211,-39.2297690928544)) ;
#72532=CARTESIAN_POINT('Origin',(209.814777625418,596.097556589211,-39.2297690928544)) ;
#72533=CARTESIAN_POINT('',(209.689777625418,596.097556589211,-39.2297690928544)) ;
#72534=CARTESIAN_POINT('Origin',(209.814777625418,596.097556589211,-39.2297690928544)) ;
#72535=CARTESIAN_POINT('Origin',(209.814777625418,596.097556589211,-39.2297690928544)) ;
#72536=CARTESIAN_POINT('Origin',(209.814777625418,599.847556589211,-39.2297690928544)) ;
#72537=CARTESIAN_POINT('',(209.689777625418,599.847556589211,-39.2297690928544)) ;
#72538=CARTESIAN_POINT('Origin',(209.814777625418,599.847556589211,-39.2297690928544)) ;
#72539=CARTESIAN_POINT('Origin',(209.814777625418,599.847556589211,-39.2297690928544)) ;
#72540=CARTESIAN_POINT('Origin',(209.814777625418,599.847556589211,-39.2297690928544)) ;
#72541=CARTESIAN_POINT('Origin',(209.814777625418,595.988181589211,-39.2297690928544)) ;
#72542=CARTESIAN_POINT('',(209.689777625418,595.988181589211,-39.2297690928544)) ;
#72543=CARTESIAN_POINT('Origin',(207.753027625418,599.847556589211,-39.2297690928544)) ;
#72544=CARTESIAN_POINT('Origin',(210.517277625419,599.847556589211,-39.2297690928544)) ;
#72545=CARTESIAN_POINT('Origin',(212.118601772286,596.097556589211,-39.2297690928544)) ;
#72546=CARTESIAN_POINT('',(212.118601772286,595.972556589211,-39.2297690928544)) ;
#72547=CARTESIAN_POINT('Origin',(210.517277625419,596.097556589211,-39.2297690928544)) ;
#72548=CARTESIAN_POINT('Origin',(210.517277625419,595.988181589211,-39.2297690928544)) ;
#72549=CARTESIAN_POINT('Origin',(210.517277625419,596.097556589211,-39.2297690928544)) ;
#72550=CARTESIAN_POINT('Origin',(210.517277625419,599.847556589211,-39.2297690928544)) ;
#72551=CARTESIAN_POINT('Origin',(210.517277625419,596.097556589211,-39.2297690928544)) ;
#72552=CARTESIAN_POINT('Origin',(210.517277625419,599.847556589211,-39.2297690928544)) ;
#72553=CARTESIAN_POINT('Origin',(202.26227762542,607.982556589212,-39.8669650424525)) ;
#72554=CARTESIAN_POINT('Origin',(202.26227762542,607.982556589212,-39.4182700580611)) ;
#72555=CARTESIAN_POINT('Origin',(212.118601772288,605.597556589211,-39.2297700580611)) ;
#72556=CARTESIAN_POINT('',(201.55977762542,605.472556589211,-39.2297700580612)) ;
#72557=CARTESIAN_POINT('',(201.55977762542,605.597556589211,-39.3547700580611)) ;
#72558=CARTESIAN_POINT('Origin',(201.55977762542,605.597556589211,-39.2297700580612)) ;
#72559=CARTESIAN_POINT('',(212.118601772288,605.472556589211,-39.2297700580611)) ;
#72560=CARTESIAN_POINT('',(202.26227762542,605.597556589211,-39.3547700580611)) ;
#72561=CARTESIAN_POINT('Origin',(202.26227762542,605.597556589211,-39.2297700580612)) ;
#72562=CARTESIAN_POINT('',(212.118601772288,605.597556589211,-39.3547700580611)) ;
#72563=CARTESIAN_POINT('Origin',(202.26227762542,608.171056589212,-39.4182700580612)) ;
#72564=CARTESIAN_POINT('',(202.26227762542,608.171056589212,-39.3547700580612)) ;
#72565=CARTESIAN_POINT('Origin',(202.26227762542,608.171056589212,-39.4182700580612)) ;
#72566=CARTESIAN_POINT('Origin',(202.26227762542,608.171056589212,-39.2297700580612)) ;
#72567=CARTESIAN_POINT('Origin',(202.26227762542,605.488181589211,-39.2297700580612)) ;
#72568=CARTESIAN_POINT('',(202.26227762542,609.347556589211,-39.3547700580612)) ;
#72569=CARTESIAN_POINT('Origin',(202.26227762542,609.347556589211,-39.2297700580612)) ;
#72570=CARTESIAN_POINT('',(202.26227762542,605.488181589211,-39.3547700580611)) ;
#72571=CARTESIAN_POINT('Origin',(201.55977762542,608.171056589212,-39.4182700580612)) ;
#72572=CARTESIAN_POINT('',(201.55977762542,608.171056589212,-39.3547700580612)) ;
#72573=CARTESIAN_POINT('Origin',(201.55977762542,608.171056589212,-39.4182700580612)) ;
#72574=CARTESIAN_POINT('Origin',(201.55977762542,608.171056589212,-39.2297700580612)) ;
#72575=CARTESIAN_POINT('Origin',(202.26227762542,606.774056589212,-39.4182700580611)) ;
#72576=CARTESIAN_POINT('',(202.26227762542,606.837556589212,-39.4182700580611)) ;
#72577=CARTESIAN_POINT('',(202.26227762542,606.774056589212,-39.3547700580611)) ;
#72578=CARTESIAN_POINT('Origin',(202.26227762542,606.774056589212,-39.4182700580611)) ;
#72579=CARTESIAN_POINT('Origin',(202.26227762542,606.774056589212,-39.2297700580612)) ;
#72580=CARTESIAN_POINT('Origin',(202.26227762542,606.962556589212,-39.4182700580611)) ;
#72581=CARTESIAN_POINT('Origin',(202.26227762542,606.962556589212,-37.6444650424525)) ;
#72582=CARTESIAN_POINT('',(202.26227762542,606.837556589212,-37.6444650424525)) ;
#72583=CARTESIAN_POINT('Origin',(202.26227762542,605.488181589211,-39.2297700580612)) ;
#72584=CARTESIAN_POINT('Origin',(202.26227762542,605.597556589211,-39.2297700580612)) ;
#72585=CARTESIAN_POINT('',(202.26227762542,605.488181589211,-39.3547700580611)) ;
#72586=CARTESIAN_POINT('Origin',(201.55977762542,606.774056589212,-39.4182700580611)) ;
#72587=CARTESIAN_POINT('',(201.55977762542,606.774056589212,-39.3547700580611)) ;
#72588=CARTESIAN_POINT('Origin',(201.55977762542,606.774056589212,-39.4182700580611)) ;
#72589=CARTESIAN_POINT('Origin',(201.55977762542,606.774056589212,-39.2297700580612)) ;
#72590=CARTESIAN_POINT('Origin',(201.55977762542,605.488181589211,-39.2297700580612)) ;
#72591=CARTESIAN_POINT('Origin',(201.55977762542,605.597556589211,-39.2297700580612)) ;
#72592=CARTESIAN_POINT('',(201.55977762542,605.488181589211,-39.3547700580611)) ;
#72593=CARTESIAN_POINT('Origin',(219.024277625419,606.774056589212,-39.4182700580611)) ;
#72594=CARTESIAN_POINT('',(219.024277625419,606.774056589212,-39.3547700580611)) ;
#72595=CARTESIAN_POINT('',(219.024277625419,606.837556589212,-39.4182700580611)) ;
#72596=CARTESIAN_POINT('Origin',(201.55977762542,605.488181589211,-39.2297700580612)) ;
#72597=CARTESIAN_POINT('',(201.55977762542,609.347556589211,-39.3547700580611)) ;
#72598=CARTESIAN_POINT('Origin',(201.55977762542,609.347556589211,-39.2297700580612)) ;
#72599=CARTESIAN_POINT('',(201.55977762542,605.488181589211,-39.3547700580611)) ;
#72600=CARTESIAN_POINT('Origin',(218.198777625419,608.171056589212,-39.4182700580611)) ;
#72601=CARTESIAN_POINT('',(218.198777625419,608.171056589212,-39.3547700580611)) ;
#72602=CARTESIAN_POINT('Origin',(201.55977762542,605.597556589211,-39.2297700580612)) ;
#72603=CARTESIAN_POINT('Origin',(201.55977762542,605.597556589211,-39.2297700580612)) ;
#72604=CARTESIAN_POINT('Origin',(202.26227762542,605.597556589211,-39.2297700580612)) ;
#72605=CARTESIAN_POINT('Origin',(207.75302762542,609.347556589211,-39.2297700580612)) ;
#72606=CARTESIAN_POINT('Origin',(201.55977762542,609.347556589211,-39.2297700580612)) ;
#72607=CARTESIAN_POINT('',(207.75302762542,609.347556589211,-39.3547700580611)) ;
#72608=CARTESIAN_POINT('Origin',(202.26227762542,609.347556589211,-39.2297700580612)) ;
#72609=CARTESIAN_POINT('Origin',(201.55977762542,609.347556589211,-39.2297700580612)) ;
#72610=CARTESIAN_POINT('Origin',(201.55977762542,609.347556589211,-39.2297700580612)) ;
#72611=CARTESIAN_POINT('Origin',(202.26227762542,609.347556589211,-39.2297700580612)) ;
#72612=CARTESIAN_POINT('Origin',(219.849777625419,606.837556589212,-41.5221609920506)) ;
#72613=CARTESIAN_POINT('Origin',(218.19877762542,608.107556589211,-39.3547700580611)) ;
#72614=CARTESIAN_POINT('Origin',(218.19877762542,608.107556589211,-39.3547700580611)) ;
#72615=CARTESIAN_POINT('Origin',(218.19877762542,608.107556589211,-39.3547690928544)) ;
#72616=CARTESIAN_POINT('',(209.81477762542,609.347556589211,-39.3547690928544)) ;
#72617=CARTESIAN_POINT('',(209.81477762542,605.597556589211,-39.3547690928544)) ;
#72618=CARTESIAN_POINT('',(209.81477762542,605.488181589211,-39.3547690928544)) ;
#72619=CARTESIAN_POINT('',(210.51727762542,605.597556589211,-39.3547690928544)) ;
#72620=CARTESIAN_POINT('',(212.118601772288,605.597556589211,-39.3547690928544)) ;
#72621=CARTESIAN_POINT('',(210.51727762542,609.347556589211,-39.3547690928544)) ;
#72622=CARTESIAN_POINT('',(210.51727762542,605.488181589211,-39.3547690928544)) ;
#72623=CARTESIAN_POINT('',(207.75302762542,609.347556589211,-39.3547690928544)) ;
#72624=CARTESIAN_POINT('Origin',(209.81477762542,605.597556589211,-39.2297690928544)) ;
#72625=CARTESIAN_POINT('',(209.81477762542,605.472556589211,-39.2297690928544)) ;
#72626=CARTESIAN_POINT('Origin',(209.81477762542,605.597556589211,-39.2297690928544)) ;
#72627=CARTESIAN_POINT('',(209.68977762542,605.597556589211,-39.2297690928544)) ;
#72628=CARTESIAN_POINT('Origin',(209.81477762542,605.597556589211,-39.2297690928544)) ;
#72629=CARTESIAN_POINT('Origin',(209.81477762542,605.597556589211,-39.2297690928544)) ;
#72630=CARTESIAN_POINT('Origin',(209.81477762542,609.347556589211,-39.2297690928544)) ;
#72631=CARTESIAN_POINT('',(209.68977762542,609.347556589211,-39.2297690928544)) ;
#72632=CARTESIAN_POINT('Origin',(209.81477762542,609.347556589211,-39.2297690928544)) ;
#72633=CARTESIAN_POINT('Origin',(209.81477762542,609.347556589211,-39.2297690928544)) ;
#72634=CARTESIAN_POINT('Origin',(209.81477762542,609.347556589211,-39.2297690928544)) ;
#72635=CARTESIAN_POINT('Origin',(209.81477762542,605.488181589211,-39.2297690928544)) ;
#72636=CARTESIAN_POINT('',(209.68977762542,605.488181589211,-39.2297690928544)) ;
#72637=CARTESIAN_POINT('Origin',(207.75302762542,609.347556589211,-39.2297690928544)) ;
#72638=CARTESIAN_POINT('Origin',(210.51727762542,609.347556589211,-39.2297690928544)) ;
#72639=CARTESIAN_POINT('Origin',(212.118601772288,605.597556589211,-39.2297690928544)) ;
#72640=CARTESIAN_POINT('',(212.118601772288,605.472556589211,-39.2297690928544)) ;
#72641=CARTESIAN_POINT('Origin',(210.51727762542,605.597556589211,-39.2297690928544)) ;
#72642=CARTESIAN_POINT('Origin',(210.51727762542,605.488181589211,-39.2297690928544)) ;
#72643=CARTESIAN_POINT('Origin',(210.51727762542,605.597556589211,-39.2297690928544)) ;
#72644=CARTESIAN_POINT('Origin',(210.51727762542,609.347556589211,-39.2297690928544)) ;
#72645=CARTESIAN_POINT('Origin',(210.51727762542,605.597556589211,-39.2297690928544)) ;
#72646=CARTESIAN_POINT('Origin',(210.51727762542,609.347556589211,-39.2297690928544)) ;
#72647=CARTESIAN_POINT('Origin',(199.088527625413,569.472556589217,-34.0221601717606)) ;
#72648=CARTESIAN_POINT('',(199.088527625421,611.548005939917,-41.5221601717606)) ;
#72649=CARTESIAN_POINT('',(199.088527625419,603.397107238494,-41.5221601717606)) ;
#72650=CARTESIAN_POINT('Origin',(199.088527625413,569.472556589217,-34.0221601717606)) ;
#72651=CARTESIAN_POINT('',(199.088527625417,593.897107238495,-41.5221601717606)) ;
#72652=CARTESIAN_POINT('',(199.088527625419,602.048005939937,-41.5221601717606)) ;
#72653=CARTESIAN_POINT('Origin',(199.088527625413,569.472556589217,-34.0221601717606)) ;
#72654=CARTESIAN_POINT('',(199.088527625416,584.397107238494,-41.5221601717606)) ;
#72655=CARTESIAN_POINT('',(199.088527625417,592.548005939937,-41.5221601717606)) ;
#72656=CARTESIAN_POINT('Origin',(199.088527625413,569.472556589217,-34.0221601717606)) ;
#72657=CARTESIAN_POINT('',(199.088527625414,574.897107238494,-41.5221601717606)) ;
#72658=CARTESIAN_POINT('',(199.088527625416,583.048005939937,-41.5221601717606)) ;
#72659=CARTESIAN_POINT('Origin',(199.088527625413,569.472556589217,-34.0221601717606)) ;
#72660=CARTESIAN_POINT('',(199.088527625412,565.397107238498,-41.5221601717606)) ;
#72661=CARTESIAN_POINT('',(199.088527625414,573.548005939937,-41.5221601717606)) ;
#72662=CARTESIAN_POINT('Origin',(199.088527625413,569.472556589217,-34.0221601717606)) ;
#72663=CARTESIAN_POINT('',(199.088527625411,555.897107238498,-41.5221601717606)) ;
#72664=CARTESIAN_POINT('',(199.088527625412,564.04800593993,-41.5221601717606)) ;
#72665=CARTESIAN_POINT('Origin',(199.088527625413,569.472556589217,-34.0221601717606)) ;
#72666=CARTESIAN_POINT('',(199.088527625409,546.397107238498,-41.5221601717606)) ;
#72667=CARTESIAN_POINT('',(199.088527625411,554.54800593993,-41.5221601717606)) ;
#72668=CARTESIAN_POINT('Origin',(199.088527625413,569.472556589217,-34.0221601717606)) ;
#72669=CARTESIAN_POINT('',(199.088527625407,536.897107238498,-41.5221601717606)) ;
#72670=CARTESIAN_POINT('',(199.088527625409,545.04800593993,-41.5221601717606)) ;
#72671=CARTESIAN_POINT('Origin',(199.088527625413,569.472556589217,-34.0221601717606)) ;
#72672=CARTESIAN_POINT('',(199.088527625406,527.397107238498,-41.5221601717606)) ;
#72673=CARTESIAN_POINT('',(199.088527625407,535.54800593993,-41.5221601717606)) ;
#72674=CARTESIAN_POINT('Origin',(199.088527625416,584.397107238494,-41.5221601717606)) ;
#72675=CARTESIAN_POINT('',(212.588527625416,584.397107238492,-38.2721601717612)) ;
#72676=CARTESIAN_POINT('Origin',(212.588527625417,592.548005939935,-41.5221601717612)) ;
#72677=CARTESIAN_POINT('',(212.588527625417,592.548005939935,-38.2721601717612)) ;
#72678=CARTESIAN_POINT('Origin',(212.588527625411,554.548005939928,-41.5221601717612)) ;
#72679=CARTESIAN_POINT('',(212.588527625411,554.548005939928,-38.2721601717612)) ;
#72680=CARTESIAN_POINT('Origin',(199.088527625409,546.397107238498,-41.5221601717606)) ;
#72681=CARTESIAN_POINT('',(212.588527625409,546.397107238495,-38.2721601717612)) ;
#72682=CARTESIAN_POINT('Origin',(212.588527625409,545.048005939928,-41.5221601717612)) ;
#72683=CARTESIAN_POINT('',(212.588527625409,545.048005939928,-38.2721601717612)) ;
#72684=CARTESIAN_POINT('Origin',(199.088527625407,536.897107238498,-41.5221601717606)) ;
#72685=CARTESIAN_POINT('',(212.588527625408,536.897107238495,-38.2721601717612)) ;
#72686=CARTESIAN_POINT('Origin',(199.088527625414,574.897107238495,-41.5221601717606)) ;
#72687=CARTESIAN_POINT('',(212.588527625414,574.897107238492,-38.2721601717612)) ;
#72688=CARTESIAN_POINT('Origin',(212.588527625416,583.048005939935,-41.5221601717612)) ;
#72689=CARTESIAN_POINT('',(212.588527625416,583.048005939935,-38.2721601717612)) ;
#72690=CARTESIAN_POINT('Origin',(199.088527625417,593.897107238495,-41.5221601717606)) ;
#72691=CARTESIAN_POINT('',(212.588527625418,593.897107238492,-38.2721601717612)) ;
#72692=CARTESIAN_POINT('Origin',(212.588527625419,602.048005939935,-41.5221601717612)) ;
#72693=CARTESIAN_POINT('',(212.588527625419,602.048005939935,-38.2721601717612)) ;
#72694=CARTESIAN_POINT('Origin',(212.588527625412,564.048005939928,-41.5221601717612)) ;
#72695=CARTESIAN_POINT('',(212.588527625412,564.048005939928,-38.2721601717612)) ;
#72696=CARTESIAN_POINT('Origin',(199.088527625411,555.897107238498,-41.5221601717606)) ;
#72697=CARTESIAN_POINT('',(212.588527625411,555.897107238495,-38.2721601717612)) ;
#72698=CARTESIAN_POINT('Origin',(212.588527625407,535.548005939928,-41.5221601717612)) ;
#72699=CARTESIAN_POINT('',(212.588527625407,535.548005939928,-38.2721601717612)) ;
#72700=CARTESIAN_POINT('Origin',(199.088527625406,527.397107238498,-41.5221601717606)) ;
#72701=CARTESIAN_POINT('',(212.588527625406,527.397107238495,-38.2721601717612)) ;
#72702=CARTESIAN_POINT('Origin',(212.588527625414,573.548005939935,-41.5221601717612)) ;
#72703=CARTESIAN_POINT('',(212.588527625414,573.548005939935,-38.2721601717612)) ;
#72704=CARTESIAN_POINT('Origin',(199.088527625412,565.397107238498,-41.5221601717606)) ;
#72705=CARTESIAN_POINT('',(212.588527625413,565.397107238495,-38.2721601717612)) ;
#72706=CARTESIAN_POINT('Origin',(199.088527625419,603.397107238494,-41.5221601717606)) ;
#72707=CARTESIAN_POINT('',(212.588527625419,603.397107238492,-38.2721601717612)) ;
#72708=CARTESIAN_POINT('Origin',(212.58852762542,611.548005939915,-41.5221601717612)) ;
#72709=CARTESIAN_POINT('',(212.588527625421,611.548005939915,-38.2721601717612)) ;
#72710=CARTESIAN_POINT('Origin',(211.838527625423,621.71816687483,-26.5221601717612)) ;
#72711=CARTESIAN_POINT('',(199.088527625407,535.696374002382,-26.5221601716848)) ;
#72712=CARTESIAN_POINT('',(211.838533909042,535.6963740129,-26.52216017177)) ;
#72713=CARTESIAN_POINT('',(199.838521341308,535.696374013642,-26.5221601717606)) ;
#72714=CARTESIAN_POINT('',(211.838533909108,536.74873917605,-26.52216017177)) ;
#72715=CARTESIAN_POINT('',(211.838533909108,536.74873916479,-26.5221601717612)) ;
#72716=CARTESIAN_POINT('',(199.088527625408,536.748739186608,-26.5221601717606)) ;
#72717=CARTESIAN_POINT('',(204.838527625408,536.748739186607,-26.5221601717609)) ;
#72718=CARTESIAN_POINT('',(199.088527625409,545.196374002382,-26.5221601716848)) ;
#72719=CARTESIAN_POINT('',(199.088527625421,612.748739186625,-26.5221601717606)) ;
#72720=CARTESIAN_POINT('',(211.838533909044,545.1963740129,-26.52216017177)) ;
#72721=CARTESIAN_POINT('',(199.83852134131,545.196374013642,-26.5221601717606)) ;
#72722=CARTESIAN_POINT('',(211.83853390911,546.24873917605,-26.52216017177)) ;
#72723=CARTESIAN_POINT('',(211.83853390911,546.24873916479,-26.5221601717612)) ;
#72724=CARTESIAN_POINT('',(199.08852762541,546.248739186608,-26.5221601717606)) ;
#72725=CARTESIAN_POINT('',(204.83852762541,546.248739186607,-26.5221601717609)) ;
#72726=CARTESIAN_POINT('',(199.088527625411,554.696374002382,-26.5221601716848)) ;
#72727=CARTESIAN_POINT('',(199.088527625421,612.748739186625,-26.5221601717606)) ;
#72728=CARTESIAN_POINT('',(211.838533909045,554.6963740129,-26.52216017177)) ;
#72729=CARTESIAN_POINT('',(199.838521341311,554.696374013642,-26.5221601717606)) ;
#72730=CARTESIAN_POINT('',(211.838533909111,555.74873917605,-26.52216017177)) ;
#72731=CARTESIAN_POINT('',(211.838533909111,555.74873916479,-26.5221601717612)) ;
#72732=CARTESIAN_POINT('',(199.088527625411,555.748739186608,-26.5221601717606)) ;
#72733=CARTESIAN_POINT('',(204.838527625411,555.748739186607,-26.5221601717609)) ;
#72734=CARTESIAN_POINT('',(199.088527625412,564.196374002382,-26.5221601716848)) ;
#72735=CARTESIAN_POINT('',(199.088527625421,612.748739186625,-26.5221601717606)) ;
#72736=CARTESIAN_POINT('',(211.838533909047,564.1963740129,-26.5221601717699)) ;
#72737=CARTESIAN_POINT('',(199.838521341313,564.196374013642,-26.5221601717606)) ;
#72738=CARTESIAN_POINT('',(211.838533909113,565.24873917605,-26.52216017177)) ;
#72739=CARTESIAN_POINT('',(211.838533909113,565.24873916479,-26.5221601717612)) ;
#72740=CARTESIAN_POINT('',(199.088527625413,565.248739186608,-26.5221601717606)) ;
#72741=CARTESIAN_POINT('',(204.838527625413,565.248739186607,-26.5221601717609)) ;
#72742=CARTESIAN_POINT('',(199.088527625414,573.696374002382,-26.5221601716848)) ;
#72743=CARTESIAN_POINT('',(199.088527625421,612.748739186625,-26.5221601717606)) ;
#72744=CARTESIAN_POINT('',(211.838533909049,573.6963740129,-26.5221601717699)) ;
#72745=CARTESIAN_POINT('',(199.838521341315,573.696374013642,-26.5221601717606)) ;
#72746=CARTESIAN_POINT('',(211.838533909115,574.74873916553,-26.52216017177)) ;
#72747=CARTESIAN_POINT('',(211.838533909115,574.74873916479,-26.5221601717612)) ;
#72748=CARTESIAN_POINT('',(199.088527625415,574.748739176051,-26.5221601716848)) ;
#72749=CARTESIAN_POINT('',(199.838521396415,574.748739164792,-26.5221601717606)) ;
#72750=CARTESIAN_POINT('',(199.088527625416,583.196374002382,-26.5221601716848)) ;
#72751=CARTESIAN_POINT('',(199.088527625421,612.748739186625,-26.5221601717606)) ;
#72752=CARTESIAN_POINT('',(211.838533909051,583.1963740129,-26.5221601717699)) ;
#72753=CARTESIAN_POINT('',(199.838521341316,583.196374013642,-26.5221601717606)) ;
#72754=CARTESIAN_POINT('',(211.838533909116,584.24873916553,-26.52216017177)) ;
#72755=CARTESIAN_POINT('',(211.838533909116,584.24873916479,-26.5221601717612)) ;
#72756=CARTESIAN_POINT('',(199.088527625416,584.248739176051,-26.5221601716848)) ;
#72757=CARTESIAN_POINT('',(199.838521396416,584.248739164792,-26.5221601717606)) ;
#72758=CARTESIAN_POINT('',(199.088527625417,592.696374002382,-26.5221601716848)) ;
#72759=CARTESIAN_POINT('',(199.088527625421,612.748739186625,-26.5221601717606)) ;
#72760=CARTESIAN_POINT('',(211.838533909052,592.6963740129,-26.5221601717699)) ;
#72761=CARTESIAN_POINT('',(199.838521341318,592.696374013642,-26.5221601717606)) ;
#72762=CARTESIAN_POINT('',(211.838533909118,593.74873916553,-26.52216017177)) ;
#72763=CARTESIAN_POINT('',(211.838533909118,593.74873916479,-26.5221601717612)) ;
#72764=CARTESIAN_POINT('',(199.088527625418,593.748739176051,-26.5221601716848)) ;
#72765=CARTESIAN_POINT('',(199.838521396418,593.748739164792,-26.5221601717606)) ;
#72766=CARTESIAN_POINT('',(199.088527625419,602.196374002382,-26.5221601716848)) ;
#72767=CARTESIAN_POINT('',(199.088527625421,612.748739186625,-26.5221601717606)) ;
#72768=CARTESIAN_POINT('',(211.838533909054,602.1963740129,-26.52216017177)) ;
#72769=CARTESIAN_POINT('',(199.83852134132,602.196374013642,-26.5221601717606)) ;
#72770=CARTESIAN_POINT('',(211.83853390912,603.24873916553,-26.52216017177)) ;
#72771=CARTESIAN_POINT('',(211.83853390912,603.24873916479,-26.5221601717612)) ;
#72772=CARTESIAN_POINT('',(199.08852762542,603.248739176051,-26.5221601716848)) ;
#72773=CARTESIAN_POINT('',(199.83852134132,603.248739164792,-26.5221601717606)) ;
#72774=CARTESIAN_POINT('',(199.088527625421,611.696374002377,-26.5221601716849)) ;
#72775=CARTESIAN_POINT('',(199.088527625421,612.748739186625,-26.5221601717606)) ;
#72776=CARTESIAN_POINT('',(211.838533909055,611.69637401289,-26.52216017177)) ;
#72777=CARTESIAN_POINT('',(199.838521341321,611.696374013632,-26.5221601717606)) ;
#72778=CARTESIAN_POINT('',(211.838533909121,612.748739176079,-26.52216017177)) ;
#72779=CARTESIAN_POINT('',(211.838533909121,612.74873916483,-26.5221601717612)) ;
#72780=CARTESIAN_POINT('',(194.588527625421,612.748739186625,-26.5221601717604)) ;
#72781=CARTESIAN_POINT('',(199.088527625421,612.748739186625,-26.5221601717606)) ;
#72782=CARTESIAN_POINT('',(194.588527625406,526.196373991821,-26.5221601717604)) ;
#72783=CARTESIAN_POINT('',(194.588527625421,612.748739186625,-26.5221601717604)) ;
#72784=CARTESIAN_POINT('',(211.838533909041,526.196374002377,-26.52216017177)) ;
#72785=CARTESIAN_POINT('',(199.088527625406,526.19637399182,-26.5221601717606)) ;
#72786=CARTESIAN_POINT('',(211.838533909106,527.24873917605,-26.52216017177)) ;
#72787=CARTESIAN_POINT('',(211.838533909106,527.24873916479,-26.5221601717612)) ;
#72788=CARTESIAN_POINT('',(199.088527625406,527.248739186608,-26.5221601717606)) ;
#72789=CARTESIAN_POINT('',(204.838527625406,527.248739186607,-26.5221601717609)) ;
#72790=CARTESIAN_POINT('',(199.088527625421,612.748739186625,-26.5221601717606)) ;
#72791=CARTESIAN_POINT('Origin',(211.838527625423,621.71816687483,-27.2721601717612)) ;
#72792=CARTESIAN_POINT('',(212.588527625408,535.68328258344,-27.2721664559512)) ;
#72793=CARTESIAN_POINT('Origin',(211.83852762055,535.683282730381,-27.2721601756534)) ;
#72794=CARTESIAN_POINT('',(212.588527625408,536.76183059499,-27.2721664560112)) ;
#72795=CARTESIAN_POINT('',(212.588527625408,535.68328258344,-27.2721664559512)) ;
#72796=CARTESIAN_POINT('Origin',(211.838527620551,536.761830448045,-27.2721601756523)) ;
#72797=CARTESIAN_POINT('Origin',(197.838527625408,535.722556589213,-25.0221601717606)) ;
#72798=CARTESIAN_POINT('',(199.088527625407,535.548005939932,-35.0221601717606)) ;
#72799=CARTESIAN_POINT('',(212.588527625407,535.539278407464,-35.5221601717612)) ;
#72800=CARTESIAN_POINT('',(206.096960845768,535.652589127089,-29.0305933921213)) ;
#72801=CARTESIAN_POINT('',(212.588527625408,535.68328258344,-27.2721664559512)) ;
#72802=CARTESIAN_POINT('Origin',(211.838527625423,621.71816687483,-27.2721601717612)) ;
#72803=CARTESIAN_POINT('',(212.588527625409,545.18328258344,-27.2721664559512)) ;
#72804=CARTESIAN_POINT('',(212.58852762541,546.26183059499,-27.2721664560112)) ;
#72805=CARTESIAN_POINT('',(212.588527625409,545.18328258344,-27.2721664559512)) ;
#72806=CARTESIAN_POINT('Origin',(211.838527620553,546.261830448045,-27.2721601756518)) ;
#72807=CARTESIAN_POINT('Origin',(211.838527620552,545.183282730381,-27.2721601756526)) ;
#72808=CARTESIAN_POINT('Origin',(211.838527625423,621.71816687483,-27.2721601717612)) ;
#72809=CARTESIAN_POINT('',(212.588527625411,554.68328258344,-27.2721664559512)) ;
#72810=CARTESIAN_POINT('Origin',(211.838527620553,554.683282730381,-27.2721601756534)) ;
#72811=CARTESIAN_POINT('',(212.588527625411,555.76183059499,-27.2721664560112)) ;
#72812=CARTESIAN_POINT('',(212.588527625411,554.68328258344,-27.2721664559512)) ;
#72813=CARTESIAN_POINT('Origin',(211.838527620554,555.761830448045,-27.2721601756524)) ;
#72814=CARTESIAN_POINT('Origin',(211.838527625423,621.71816687483,-27.2721601717612)) ;
#72815=CARTESIAN_POINT('',(212.588527625413,564.18328258344,-27.2721664559512)) ;
#72816=CARTESIAN_POINT('Origin',(211.838527620556,564.183282730381,-27.2721601756519)) ;
#72817=CARTESIAN_POINT('',(212.588527625413,565.26183059499,-27.2721664560112)) ;
#72818=CARTESIAN_POINT('',(212.588527625413,564.18328258344,-27.2721664559512)) ;
#72819=CARTESIAN_POINT('Origin',(211.838527620555,565.261830448045,-27.2721601756536)) ;
#72820=CARTESIAN_POINT('Origin',(211.838527625423,621.71816687483,-27.2721601717612)) ;
#72821=CARTESIAN_POINT('',(212.588527625415,573.68328258343,-27.2721664559512)) ;
#72822=CARTESIAN_POINT('',(212.588527625415,574.76183059499,-27.2721664560112)) ;
#72823=CARTESIAN_POINT('',(212.588527625415,573.68328258344,-27.2721664559512)) ;
#72824=CARTESIAN_POINT('Origin',(211.838527620558,574.761830448045,-27.2721601756523)) ;
#72825=CARTESIAN_POINT('Origin',(211.838527620555,573.683282730364,-27.2721601756541)) ;
#72826=CARTESIAN_POINT('Origin',(211.838527625423,621.71816687483,-27.2721601717612)) ;
#72827=CARTESIAN_POINT('',(212.588527625416,583.18328258344,-27.2721664559512)) ;
#72828=CARTESIAN_POINT('',(212.588527625416,584.26183059499,-27.2721664560112)) ;
#72829=CARTESIAN_POINT('',(212.588527625416,583.18328258344,-27.2721664559512)) ;
#72830=CARTESIAN_POINT('Origin',(211.83852762056,584.261830448045,-27.2721601756523)) ;
#72831=CARTESIAN_POINT('Origin',(211.838527620558,583.183282730381,-27.2721601756534)) ;
#72832=CARTESIAN_POINT('Origin',(211.838527625423,621.71816687483,-27.2721601717612)) ;
#72833=CARTESIAN_POINT('',(212.588527625418,592.68328258344,-27.2721664559512)) ;
#72834=CARTESIAN_POINT('',(212.588527625418,593.76183059499,-27.2721664560112)) ;
#72835=CARTESIAN_POINT('',(212.588527625418,592.68328258344,-27.2721664559512)) ;
#72836=CARTESIAN_POINT('Origin',(211.838527620561,593.761830448045,-27.2721601756523)) ;
#72837=CARTESIAN_POINT('Origin',(211.838527620559,592.683282730381,-27.2721601756542)) ;
#72838=CARTESIAN_POINT('Origin',(211.838527625423,621.71816687483,-27.2721601717612)) ;
#72839=CARTESIAN_POINT('',(212.588527625419,602.18328258344,-27.2721664559512)) ;
#72840=CARTESIAN_POINT('Origin',(211.838527620561,602.183282730381,-27.2721601756535)) ;
#72841=CARTESIAN_POINT('',(212.58852762542,603.26183059499,-27.2721664560112)) ;
#72842=CARTESIAN_POINT('',(212.588527625419,602.18328258344,-27.2721664559512)) ;
#72843=CARTESIAN_POINT('Origin',(211.838527620563,603.261830448045,-27.2721601756519)) ;
#72844=CARTESIAN_POINT('Origin',(211.838527625423,621.71816687483,-27.2721601717612)) ;
#72845=CARTESIAN_POINT('',(212.588527625421,611.68328258343,-27.2721664559512)) ;
#72846=CARTESIAN_POINT('',(212.588527625421,612.76183059503,-27.2721664560112)) ;
#72847=CARTESIAN_POINT('',(212.588527625421,611.68328258343,-27.2721664559512)) ;
#72848=CARTESIAN_POINT('Origin',(211.838527620563,612.761830448138,-27.2721601756519)) ;
#72849=CARTESIAN_POINT('Origin',(211.838527620567,611.683282730347,-27.2721601756485)) ;
#72850=CARTESIAN_POINT('Origin',(197.838527625406,527.449472433283,-38.0221601717605)) ;
#72851=CARTESIAN_POINT('',(212.588527625406,527.26183059499,-27.2721664560112)) ;
#72852=CARTESIAN_POINT('Origin',(211.838527620549,527.261830448045,-27.2721601756523)) ;
#72853=CARTESIAN_POINT('',(212.588527625406,527.405834770959,-35.5221601717612)) ;
#72854=CARTESIAN_POINT('',(212.588527625406,527.3971072385,-35.0221601717612)) ;
#72855=CARTESIAN_POINT('',(209.49143822564,527.351774874399,-32.4250707719951)) ;
#72856=CARTESIAN_POINT('',(199.088527625406,527.261830594102,-27.2721664048106)) ;
#72857=CARTESIAN_POINT('Origin',(211.838527625423,621.71816687483,-27.2721601717612)) ;
#72858=CARTESIAN_POINT('',(212.588527625406,526.18328258344,-27.2721664559512)) ;
#72859=CARTESIAN_POINT('',(212.588527625406,526.18328258344,-27.2721664559512)) ;
#72860=CARTESIAN_POINT('Origin',(211.838527620549,526.183282730381,-27.2721601756526)) ;
#72861=CARTESIAN_POINT('Origin',(212.33852762541,547.97255658922,-35.2721601717612)) ;
#72862=CARTESIAN_POINT('',(212.58852762541,547.97255658922,-35.5221601717612)) ;
#72863=CARTESIAN_POINT('Origin',(212.33852762541,547.97255658922,-35.2721601717612)) ;
#72864=CARTESIAN_POINT('',(212.088527625408,536.897107238495,-35.0221601717612)) ;
#72865=CARTESIAN_POINT('',(212.588527625408,536.905834770959,-35.5221601717612)) ;
#72866=CARTESIAN_POINT('',(209.449988760834,536.851051371299,-32.3836213071874)) ;
#72867=CARTESIAN_POINT('',(212.588527625409,545.039278407464,-35.5221601717612)) ;
#72868=CARTESIAN_POINT('',(212.58852762541,547.97255658922,-35.5221601717612)) ;
#72869=CARTESIAN_POINT('',(212.088527625409,545.048005939928,-35.0221601717612)) ;
#72870=CARTESIAN_POINT('',(206.138410310577,545.15186562399,-29.0720428569291)) ;
#72871=CARTESIAN_POINT('',(212.08852762541,547.97255658922,-35.0221601717612)) ;
#72872=CARTESIAN_POINT('Origin',(212.33852762541,547.97255658922,-35.2721601717612)) ;
#72873=CARTESIAN_POINT('',(212.088527625409,546.397107238495,-35.0221601717612)) ;
#72874=CARTESIAN_POINT('',(212.588527625409,546.405834770959,-35.5221601717612)) ;
#72875=CARTESIAN_POINT('',(209.408539296028,546.3503278682,-32.3421718423797)) ;
#72876=CARTESIAN_POINT('',(212.588527625411,554.539278407464,-35.5221601717612)) ;
#72877=CARTESIAN_POINT('',(212.58852762541,547.97255658922,-35.5221601717612)) ;
#72878=CARTESIAN_POINT('',(212.088527625411,554.548005939928,-35.0221601717612)) ;
#72879=CARTESIAN_POINT('',(206.179859775386,554.65114212089,-29.1134923217368)) ;
#72880=CARTESIAN_POINT('',(212.08852762541,547.97255658922,-35.0221601717612)) ;
#72881=CARTESIAN_POINT('Origin',(212.33852762541,547.97255658922,-35.2721601717612)) ;
#72882=CARTESIAN_POINT('',(212.088527625411,555.897107238495,-35.0221601717612)) ;
#72883=CARTESIAN_POINT('',(212.588527625411,555.90583477096,-35.5221601717612)) ;
#72884=CARTESIAN_POINT('',(209.367089831222,555.8496043651,-32.300722377572)) ;
#72885=CARTESIAN_POINT('',(212.588527625412,564.039278407464,-35.5221601717612)) ;
#72886=CARTESIAN_POINT('',(212.58852762541,547.97255658922,-35.5221601717612)) ;
#72887=CARTESIAN_POINT('',(212.088527625412,564.048005939928,-35.0221601717612)) ;
#72888=CARTESIAN_POINT('',(206.221309240196,564.150418617791,-29.1549417865445)) ;
#72889=CARTESIAN_POINT('',(212.08852762541,547.97255658922,-35.0221601717612)) ;
#72890=CARTESIAN_POINT('Origin',(212.33852762541,547.97255658922,-35.2721601717612)) ;
#72891=CARTESIAN_POINT('',(212.088527625413,565.397107238495,-35.0221601717612)) ;
#72892=CARTESIAN_POINT('',(212.588527625413,565.405834770959,-35.5221601717612)) ;
#72893=CARTESIAN_POINT('',(209.325640366416,565.348880862001,-32.2592729127642)) ;
#72894=CARTESIAN_POINT('',(212.588527625414,573.53927840747,-35.5221601717612)) ;
#72895=CARTESIAN_POINT('',(212.58852762541,547.97255658922,-35.5221601717612)) ;
#72896=CARTESIAN_POINT('',(212.088527625414,573.548005939935,-35.0221601717612)) ;
#72897=CARTESIAN_POINT('',(209.513253733442,573.592957512927,-32.4468862797886)) ;
#72898=CARTESIAN_POINT('',(212.08852762541,547.97255658922,-35.0221601717612)) ;
#72899=CARTESIAN_POINT('Origin',(212.33852762541,547.97255658922,-35.2721601717612)) ;
#72900=CARTESIAN_POINT('',(212.088527625414,574.897107238492,-35.0221601717612)) ;
#72901=CARTESIAN_POINT('',(212.588527625414,574.905834770956,-35.5221601717612)) ;
#72902=CARTESIAN_POINT('',(206.033695873173,574.791419757129,-28.9673284195202)) ;
#72903=CARTESIAN_POINT('',(212.588527625416,583.039278407471,-35.5221601717612)) ;
#72904=CARTESIAN_POINT('',(212.58852762541,547.97255658922,-35.5221601717612)) ;
#72905=CARTESIAN_POINT('',(212.088527625416,583.048005939935,-35.0221601717612)) ;
#72906=CARTESIAN_POINT('',(209.554703198251,583.092234009828,-32.4883357445963)) ;
#72907=CARTESIAN_POINT('',(212.08852762541,547.97255658922,-35.0221601717612)) ;
#72908=CARTESIAN_POINT('Origin',(212.33852762541,547.97255658922,-35.2721601717612)) ;
#72909=CARTESIAN_POINT('',(212.088527625416,584.397107238492,-35.0221601717612)) ;
#72910=CARTESIAN_POINT('',(212.588527625416,584.405834770956,-35.5221601717612)) ;
#72911=CARTESIAN_POINT('',(205.992246408367,584.290696254029,-28.9258789547125)) ;
#72912=CARTESIAN_POINT('',(212.588527625417,592.539278407471,-35.5221601717612)) ;
#72913=CARTESIAN_POINT('',(212.58852762541,547.97255658922,-35.5221601717612)) ;
#72914=CARTESIAN_POINT('',(212.088527625417,592.548005939935,-35.0221601717612)) ;
#72915=CARTESIAN_POINT('',(209.59615266306,592.591510506729,-32.529785209404)) ;
#72916=CARTESIAN_POINT('',(212.08852762541,547.97255658922,-35.0221601717612)) ;
#72917=CARTESIAN_POINT('Origin',(212.33852762541,547.97255658922,-35.2721601717612)) ;
#72918=CARTESIAN_POINT('',(212.088527625418,593.897107238492,-35.0221601717612)) ;
#72919=CARTESIAN_POINT('',(212.588527625418,593.905834770956,-35.5221601717612)) ;
#72920=CARTESIAN_POINT('',(205.950796943561,593.78997275093,-28.8844294899048)) ;
#72921=CARTESIAN_POINT('',(212.588527625419,602.039278407471,-35.5221601717612)) ;
#72922=CARTESIAN_POINT('',(212.58852762541,547.97255658922,-35.5221601717612)) ;
#72923=CARTESIAN_POINT('',(212.088527625419,602.048005939935,-35.0221601717612)) ;
#72924=CARTESIAN_POINT('',(209.63760212787,602.090787003629,-32.5712346742117)) ;
#72925=CARTESIAN_POINT('',(212.08852762541,547.97255658922,-35.0221601717612)) ;
#72926=CARTESIAN_POINT('Origin',(212.33852762541,547.97255658922,-35.2721601717612)) ;
#72927=CARTESIAN_POINT('',(212.088527625419,603.397107238492,-35.0221601717612)) ;
#72928=CARTESIAN_POINT('',(212.588527625419,603.405834770956,-35.5221601717612)) ;
#72929=CARTESIAN_POINT('',(205.909347478755,603.28924924783,-28.842980025097)) ;
#72930=CARTESIAN_POINT('',(212.588527625421,611.539278407451,-35.5221601717612)) ;
#72931=CARTESIAN_POINT('',(212.58852762541,547.97255658922,-35.5221601717612)) ;
#72932=CARTESIAN_POINT('',(212.088527625421,611.548005939915,-35.0221601717612)) ;
#72933=CARTESIAN_POINT('',(209.679051592679,611.59006350051,-32.6126841390194)) ;
#72934=CARTESIAN_POINT('',(212.08852762541,547.97255658922,-35.0221601717612)) ;
#72935=CARTESIAN_POINT('Origin',(197.838527625406,526.222556589213,-25.0221601717606)) ;
#72936=CARTESIAN_POINT('',(212.588527625406,526.18328258344,-27.2721664559512)) ;
#72937=CARTESIAN_POINT('',(194.588527625405,525.934548017903,-41.5221601717604)) ;
#72938=CARTESIAN_POINT('Origin',(197.838527625408,536.949472433283,-38.0221601717605)) ;
#72939=CARTESIAN_POINT('',(212.588527625408,536.8971072385,-35.0221601717612)) ;
#72940=CARTESIAN_POINT('',(199.088527625408,536.897107238499,-35.0221601717606)) ;
#72941=CARTESIAN_POINT('',(201.838527625408,536.897107238497,-35.0221601717607)) ;
#72942=CARTESIAN_POINT('',(199.088527625408,536.761830595002,-27.2721664563906)) ;
#72943=CARTESIAN_POINT('Origin',(197.83852762541,545.222556589213,-25.0221601717606)) ;
#72944=CARTESIAN_POINT('',(199.088527625409,545.048005939932,-35.0221601717606)) ;
#72945=CARTESIAN_POINT('',(199.088527625409,545.048005939932,-35.0221601717606)) ;
#72946=CARTESIAN_POINT('',(201.838527625409,545.04800593993,-35.0221601717607)) ;
#72947=CARTESIAN_POINT('',(212.588527625409,545.18328258344,-27.2721664559512)) ;
#72948=CARTESIAN_POINT('Origin',(197.838527625409,546.449472433283,-38.0221601717605)) ;
#72949=CARTESIAN_POINT('',(212.588527625409,546.3971072385,-35.0221601717612)) ;
#72950=CARTESIAN_POINT('',(199.088527625409,546.3971072385,-35.0221601717606)) ;
#72951=CARTESIAN_POINT('',(201.838527625409,546.397107238497,-35.0221601717607)) ;
#72952=CARTESIAN_POINT('',(199.08852762541,546.261830594102,-27.2721664048106)) ;
#72953=CARTESIAN_POINT('Origin',(197.838527625411,554.722556589213,-25.0221601717605)) ;
#72954=CARTESIAN_POINT('',(199.088527625411,554.548005939932,-35.0221601717606)) ;
#72955=CARTESIAN_POINT('',(199.088527625411,554.548005939932,-35.0221601717606)) ;
#72956=CARTESIAN_POINT('',(201.838527625411,554.54800593993,-35.0221601717607)) ;
#72957=CARTESIAN_POINT('',(212.588527625411,554.68328258344,-27.2721664559512)) ;
#72958=CARTESIAN_POINT('Origin',(197.838527625411,555.949472433283,-38.0221601717606)) ;
#72959=CARTESIAN_POINT('',(212.588527625411,555.8971072385,-35.0221601717612)) ;
#72960=CARTESIAN_POINT('',(199.088527625411,555.897107238499,-35.0221601717606)) ;
#72961=CARTESIAN_POINT('',(201.838527625411,555.897107238497,-35.0221601717607)) ;
#72962=CARTESIAN_POINT('',(199.088527625411,555.761830595002,-27.2721664563906)) ;
#72963=CARTESIAN_POINT('Origin',(197.838527625413,564.222556589213,-25.0221601717605)) ;
#72964=CARTESIAN_POINT('',(199.088527625412,564.048005939932,-35.0221601717606)) ;
#72965=CARTESIAN_POINT('',(199.088527625412,564.048005939932,-35.0221601717606)) ;
#72966=CARTESIAN_POINT('',(201.838527625412,564.04800593993,-35.0221601717607)) ;
#72967=CARTESIAN_POINT('',(212.588527625413,564.18328258344,-27.2721664559512)) ;
#72968=CARTESIAN_POINT('Origin',(197.838527625413,565.449472433283,-38.0221601717606)) ;
#72969=CARTESIAN_POINT('',(212.588527625413,565.3971072385,-35.0221601717612)) ;
#72970=CARTESIAN_POINT('',(199.088527625413,565.397107238499,-35.0221601717606)) ;
#72971=CARTESIAN_POINT('',(201.838527625413,565.397107238497,-35.0221601717607)) ;
#72972=CARTESIAN_POINT('',(199.088527625413,565.261830595002,-27.2721664563906)) ;
#72973=CARTESIAN_POINT('Origin',(197.838527625414,573.495640745153,-38.0221601717606)) ;
#72974=CARTESIAN_POINT('',(199.088527625414,573.548005939932,-35.0221601717606)) ;
#72975=CARTESIAN_POINT('',(199.088527625414,573.548005939932,-35.0221601717606)) ;
#72976=CARTESIAN_POINT('',(201.838527625414,573.548005939937,-35.0221601717607)) ;
#72977=CARTESIAN_POINT('',(212.588527625415,573.68328258344,-27.2721664559512)) ;
#72978=CARTESIAN_POINT('Origin',(197.838527625415,574.722556589213,-25.0221601717605)) ;
#72979=CARTESIAN_POINT('',(212.588527625414,574.8971072385,-35.0221601717612)) ;
#72980=CARTESIAN_POINT('',(199.088527625414,574.897107238499,-35.0221601717606)) ;
#72981=CARTESIAN_POINT('',(201.838527625414,574.897107238494,-35.0221601717607)) ;
#72982=CARTESIAN_POINT('',(199.088527625415,574.761830594102,-27.2721664048106)) ;
#72983=CARTESIAN_POINT('Origin',(197.838527625416,582.995640745153,-38.0221601717605)) ;
#72984=CARTESIAN_POINT('',(199.088527625416,583.048005939932,-35.0221601717606)) ;
#72985=CARTESIAN_POINT('',(199.088527625416,583.048005939932,-35.0221601717606)) ;
#72986=CARTESIAN_POINT('',(201.838527625416,583.048005939937,-35.0221601717607)) ;
#72987=CARTESIAN_POINT('',(212.588527625416,583.18328258344,-27.2721664559512)) ;
#72988=CARTESIAN_POINT('Origin',(197.838527625416,584.222556589213,-25.0221601717606)) ;
#72989=CARTESIAN_POINT('',(212.588527625416,584.3971072385,-35.0221601717612)) ;
#72990=CARTESIAN_POINT('',(199.088527625416,584.3971072385,-35.0221601717606)) ;
#72991=CARTESIAN_POINT('',(201.838527625416,584.397107238494,-35.0221601717607)) ;
#72992=CARTESIAN_POINT('',(199.088527625416,584.261830594102,-27.2721664048106)) ;
#72993=CARTESIAN_POINT('Origin',(197.838527625417,592.495640745153,-38.0221601717606)) ;
#72994=CARTESIAN_POINT('',(199.088527625417,592.548005939932,-35.0221601717606)) ;
#72995=CARTESIAN_POINT('',(199.088527625417,592.548005939932,-35.0221601717606)) ;
#72996=CARTESIAN_POINT('',(201.838527625417,592.548005939937,-35.0221601717607)) ;
#72997=CARTESIAN_POINT('',(212.588527625418,592.68328258344,-27.2721664559512)) ;
#72998=CARTESIAN_POINT('Origin',(197.838527625418,593.722556589213,-25.0221601717605)) ;
#72999=CARTESIAN_POINT('',(212.588527625418,593.8971072385,-35.0221601717612)) ;
#73000=CARTESIAN_POINT('',(199.088527625418,593.8971072385,-35.0221601717606)) ;
#73001=CARTESIAN_POINT('',(201.838527625418,593.897107238494,-35.0221601717607)) ;
#73002=CARTESIAN_POINT('',(199.088527625418,593.761830594102,-27.2721664048106)) ;
#73003=CARTESIAN_POINT('Origin',(197.838527625419,601.995640745153,-38.0221601717605)) ;
#73004=CARTESIAN_POINT('',(199.088527625419,602.048005939932,-35.0221601717606)) ;
#73005=CARTESIAN_POINT('',(199.088527625419,602.048005939932,-35.0221601717606)) ;
#73006=CARTESIAN_POINT('',(201.838527625419,602.048005939937,-35.0221601717607)) ;
#73007=CARTESIAN_POINT('',(212.588527625419,602.18328258344,-27.2721664559512)) ;
#73008=CARTESIAN_POINT('Origin',(197.83852762542,603.222556589213,-25.0221601717605)) ;
#73009=CARTESIAN_POINT('',(212.588527625419,603.3971072385,-35.0221601717612)) ;
#73010=CARTESIAN_POINT('',(199.088527625419,603.397107238499,-35.0221601717606)) ;
#73011=CARTESIAN_POINT('',(201.838527625419,603.397107238494,-35.0221601717607)) ;
#73012=CARTESIAN_POINT('',(199.08852762542,603.261830595002,-27.2721664563906)) ;
#73013=CARTESIAN_POINT('Origin',(197.838527625421,611.495640745133,-38.0221601717605)) ;
#73014=CARTESIAN_POINT('',(199.088527625421,611.548005939932,-35.0221601717606)) ;
#73015=CARTESIAN_POINT('',(199.088527625421,611.548005939932,-35.0221601717606)) ;
#73016=CARTESIAN_POINT('',(201.838527625421,611.548005939917,-35.0221601717607)) ;
#73017=CARTESIAN_POINT('',(212.588527625421,611.68328258343,-27.2721664559512)) ;
#73018=CARTESIAN_POINT('Origin',(199.088527625413,569.472556589217,-34.0221601717606)) ;
#73019=CARTESIAN_POINT('Origin',(194.588527625414,569.472556589218,-34.0221601717604)) ;
#73020=CARTESIAN_POINT('',(194.588527625421,612.748739186625,-26.5221601717604)) ;
#73021=CARTESIAN_POINT('Origin',(199.088527625413,569.472556589217,-34.0221601717606)) ;
#73022=CARTESIAN_POINT('',(199.08852762541,547.972556589222,-35.0221601717606)) ;
#73023=CARTESIAN_POINT('Origin',(199.088527625413,569.472556589217,-34.0221601717606)) ;
#73024=CARTESIAN_POINT('',(199.08852762541,547.972556589222,-35.0221601717606)) ;
#73025=CARTESIAN_POINT('Origin',(199.088527625413,569.472556589217,-34.0221601717606)) ;
#73026=CARTESIAN_POINT('',(199.08852762541,547.972556589222,-35.0221601717606)) ;
#73027=CARTESIAN_POINT('Origin',(199.088527625413,569.472556589217,-34.0221601717606)) ;
#73028=CARTESIAN_POINT('',(199.08852762541,547.972556589222,-35.0221601717606)) ;
#73029=CARTESIAN_POINT('Origin',(199.088527625413,569.472556589217,-34.0221601717606)) ;
#73030=CARTESIAN_POINT('',(199.08852762541,547.972556589222,-35.0221601717606)) ;
#73031=CARTESIAN_POINT('Origin',(199.088527625413,569.472556589217,-34.0221601717606)) ;
#73032=CARTESIAN_POINT('',(199.08852762541,547.972556589222,-35.0221601717606)) ;
#73033=CARTESIAN_POINT('Origin',(199.088527625413,569.472556589217,-34.0221601717606)) ;
#73034=CARTESIAN_POINT('',(199.08852762541,547.972556589222,-35.0221601717606)) ;
#73035=CARTESIAN_POINT('Origin',(199.088527625413,569.472556589217,-34.0221601717606)) ;
#73036=CARTESIAN_POINT('',(199.08852762541,547.972556589222,-35.0221601717606)) ;
#73037=CARTESIAN_POINT('Origin',(205.838527625413,569.472556589231,-35.0221601717609)) ;
#73038=CARTESIAN_POINT('',(203.155186246477,607.472556589211,-35.0221601717609)) ;
#73039=CARTESIAN_POINT('Origin',(206.03852762542,607.472556589211,-35.0221601717609)) ;
#73040=CARTESIAN_POINT('Origin',(206.03852762542,607.472556589211,-35.0982690928543)) ;
#73041=CARTESIAN_POINT('',(208.89602762542,607.472556589211,-35.0982690928543)) ;
#73042=CARTESIAN_POINT('',(203.18102762542,607.472556589211,-35.0982690928543)) ;
#73043=CARTESIAN_POINT('Origin',(206.03852762542,607.472556589211,-35.0982690928543)) ;
#73044=CARTESIAN_POINT('Origin',(206.03852762542,607.472556589211,-35.0982690928543)) ;
#73045=CARTESIAN_POINT('Origin',(203.05602762542,607.472556589211,-35.0982690928543)) ;
#73046=CARTESIAN_POINT('Origin',(206.03852762542,607.472556589211,-34.9732690928544)) ;
#73047=CARTESIAN_POINT('',(208.89602762542,607.472556589211,-36.8802690928544)) ;
#73048=CARTESIAN_POINT('Origin',(206.03852762542,607.472556589211,-36.8802690928544)) ;
#73049=CARTESIAN_POINT('',(208.89602762542,607.472556589211,-34.9732690928544)) ;
#73050=CARTESIAN_POINT('Origin',(206.03852762542,607.472556589211,-36.8802690928544)) ;
#73051=CARTESIAN_POINT('Origin',(208.77102762542,607.472556589211,-36.8802690928544)) ;
#73052=CARTESIAN_POINT('Origin',(206.038425919156,605.472556589211,-37.9581389501285)) ;
#73053=CARTESIAN_POINT('',(201.55977762542,605.472556589211,-40.5297040214914)) ;
#73054=CARTESIAN_POINT('Origin',(201.55977762542,605.597556589211,-40.5297040214914)) ;
#73055=CARTESIAN_POINT('Origin',(205.838527625413,569.472556589231,-35.0221601717609)) ;
#73056=CARTESIAN_POINT('',(203.155186246476,597.972556589211,-35.0221601717609)) ;
#73057=CARTESIAN_POINT('Origin',(206.038527625418,597.972556589211,-35.0221601717609)) ;
#73058=CARTESIAN_POINT('Origin',(206.038527625418,597.972556589211,-35.0982690928543)) ;
#73059=CARTESIAN_POINT('',(208.896027625418,597.972556589211,-35.0982690928543)) ;
#73060=CARTESIAN_POINT('',(203.181027625418,597.972556589211,-35.0982690928543)) ;
#73061=CARTESIAN_POINT('Origin',(206.038527625418,597.972556589211,-35.0982690928543)) ;
#73062=CARTESIAN_POINT('Origin',(206.038527625418,597.972556589211,-35.0982690928543)) ;
#73063=CARTESIAN_POINT('Origin',(203.056027625418,597.972556589211,-35.0982690928543)) ;
#73064=CARTESIAN_POINT('Origin',(206.038527625418,597.972556589211,-34.9732690928544)) ;
#73065=CARTESIAN_POINT('',(208.896027625418,597.972556589211,-36.8802690928544)) ;
#73066=CARTESIAN_POINT('Origin',(206.038527625418,597.972556589211,-36.8802690928544)) ;
#73067=CARTESIAN_POINT('',(208.896027625418,597.972556589211,-34.9732690928544)) ;
#73068=CARTESIAN_POINT('Origin',(206.038527625418,597.972556589211,-36.8802690928544)) ;
#73069=CARTESIAN_POINT('Origin',(208.771027625418,597.972556589211,-36.8802690928544)) ;
#73070=CARTESIAN_POINT('Origin',(206.038425919154,595.972556589211,-37.9581389501285)) ;
#73071=CARTESIAN_POINT('',(201.559777625419,595.972556589211,-40.5297040214914)) ;
#73072=CARTESIAN_POINT('Origin',(201.559777625419,596.097556589211,-40.5297040214914)) ;
#73073=CARTESIAN_POINT('Origin',(205.838527625413,569.472556589231,-35.0221601717609)) ;
#73074=CARTESIAN_POINT('',(203.155186246474,588.472556589211,-35.0221601717609)) ;
#73075=CARTESIAN_POINT('Origin',(206.038527625417,588.472556589211,-35.0221601717609)) ;
#73076=CARTESIAN_POINT('Origin',(206.038527625417,588.472556589211,-35.0982690928543)) ;
#73077=CARTESIAN_POINT('',(208.896027625417,588.472556589211,-35.0982690928543)) ;
#73078=CARTESIAN_POINT('',(203.181027625417,588.472556589211,-35.0982690928543)) ;
#73079=CARTESIAN_POINT('Origin',(206.038527625417,588.472556589211,-35.0982690928543)) ;
#73080=CARTESIAN_POINT('Origin',(206.038527625417,588.472556589211,-35.0982690928543)) ;
#73081=CARTESIAN_POINT('Origin',(203.056027625417,588.472556589211,-35.0982690928543)) ;
#73082=CARTESIAN_POINT('Origin',(206.038527625417,588.472556589211,-34.9732690928544)) ;
#73083=CARTESIAN_POINT('',(208.896027625417,588.472556589211,-36.8802690928544)) ;
#73084=CARTESIAN_POINT('Origin',(206.038527625417,588.472556589211,-36.8802690928544)) ;
#73085=CARTESIAN_POINT('',(208.896027625417,588.472556589211,-34.9732690928544)) ;
#73086=CARTESIAN_POINT('Origin',(206.038527625417,588.472556589211,-36.8802690928544)) ;
#73087=CARTESIAN_POINT('Origin',(208.771027625417,588.472556589211,-36.8802690928544)) ;
#73088=CARTESIAN_POINT('Origin',(206.038425919152,586.472556589211,-37.9581389501285)) ;
#73089=CARTESIAN_POINT('',(201.559777625417,586.472556589211,-40.5297040214914)) ;
#73090=CARTESIAN_POINT('Origin',(201.559777625417,586.597556589211,-40.5297040214914)) ;
#73091=CARTESIAN_POINT('Origin',(205.838527625413,569.472556589231,-35.0221601717609)) ;
#73092=CARTESIAN_POINT('',(203.155186246472,578.972556589211,-35.0221601717609)) ;
#73093=CARTESIAN_POINT('Origin',(206.038527625415,578.972556589211,-35.0221601717609)) ;
#73094=CARTESIAN_POINT('Origin',(206.038527625415,578.972556589211,-35.0982690928543)) ;
#73095=CARTESIAN_POINT('',(208.896027625415,578.972556589211,-35.0982690928543)) ;
#73096=CARTESIAN_POINT('',(203.181027625415,578.972556589211,-35.0982690928543)) ;
#73097=CARTESIAN_POINT('Origin',(206.038527625415,578.972556589211,-35.0982690928543)) ;
#73098=CARTESIAN_POINT('Origin',(206.038527625415,578.972556589211,-35.0982690928543)) ;
#73099=CARTESIAN_POINT('Origin',(203.056027625415,578.972556589211,-35.0982690928543)) ;
#73100=CARTESIAN_POINT('Origin',(206.038527625415,578.972556589211,-34.9732690928544)) ;
#73101=CARTESIAN_POINT('',(208.896027625415,578.972556589211,-36.8802690928544)) ;
#73102=CARTESIAN_POINT('Origin',(206.038527625415,578.972556589211,-36.8802690928544)) ;
#73103=CARTESIAN_POINT('',(208.896027625415,578.972556589211,-34.9732690928544)) ;
#73104=CARTESIAN_POINT('Origin',(206.038527625415,578.972556589211,-36.8802690928544)) ;
#73105=CARTESIAN_POINT('Origin',(208.771027625415,578.972556589211,-36.8802690928544)) ;
#73106=CARTESIAN_POINT('Origin',(206.038425919151,576.972556589211,-37.9581389501285)) ;
#73107=CARTESIAN_POINT('',(201.559777625416,576.972556589211,-40.5297040214914)) ;
#73108=CARTESIAN_POINT('Origin',(201.559777625415,577.097556589211,-40.5297040214914)) ;
#73109=CARTESIAN_POINT('Origin',(205.838527625413,569.472556589231,-35.0221601717609)) ;
#73110=CARTESIAN_POINT('',(203.155186246471,569.472556589211,-35.0221601717609)) ;
#73111=CARTESIAN_POINT('Origin',(206.038527625413,569.472556589211,-35.0221601717609)) ;
#73112=CARTESIAN_POINT('Origin',(206.038527625413,569.472556589211,-35.0982690928543)) ;
#73113=CARTESIAN_POINT('',(208.896027625413,569.472556589211,-35.0982690928543)) ;
#73114=CARTESIAN_POINT('',(203.181027625413,569.472556589211,-35.0982690928543)) ;
#73115=CARTESIAN_POINT('Origin',(206.038527625413,569.472556589211,-35.0982690928543)) ;
#73116=CARTESIAN_POINT('Origin',(206.038527625413,569.472556589211,-35.0982690928543)) ;
#73117=CARTESIAN_POINT('Origin',(203.056027625413,569.472556589211,-35.0982690928543)) ;
#73118=CARTESIAN_POINT('Origin',(206.038527625413,569.472556589211,-34.9732690928544)) ;
#73119=CARTESIAN_POINT('',(208.896027625413,569.472556589211,-36.8802690928544)) ;
#73120=CARTESIAN_POINT('Origin',(206.038527625413,569.472556589211,-36.8802690928544)) ;
#73121=CARTESIAN_POINT('',(208.896027625413,569.472556589211,-34.9732690928544)) ;
#73122=CARTESIAN_POINT('Origin',(206.038527625413,569.472556589211,-36.8802690928544)) ;
#73123=CARTESIAN_POINT('Origin',(208.771027625413,569.472556589211,-36.8802690928544)) ;
#73124=CARTESIAN_POINT('Origin',(206.038425919149,567.47255658921,-37.9581389501285)) ;
#73125=CARTESIAN_POINT('',(201.559777625414,567.47255658921,-40.5297040214914)) ;
#73126=CARTESIAN_POINT('Origin',(201.559777625414,567.59755658921,-40.5297040214914)) ;
#73127=CARTESIAN_POINT('Origin',(205.838527625413,569.472556589231,-35.0221601717609)) ;
#73128=CARTESIAN_POINT('',(203.155186246469,559.972556589211,-35.0221601717609)) ;
#73129=CARTESIAN_POINT('Origin',(206.038527625412,559.972556589211,-35.0221601717609)) ;
#73130=CARTESIAN_POINT('Origin',(206.038527625412,559.972556589211,-35.0982690928543)) ;
#73131=CARTESIAN_POINT('',(208.896027625412,559.972556589211,-35.0982690928543)) ;
#73132=CARTESIAN_POINT('',(203.181027625412,559.972556589211,-35.0982690928543)) ;
#73133=CARTESIAN_POINT('Origin',(206.038527625412,559.972556589211,-35.0982690928543)) ;
#73134=CARTESIAN_POINT('Origin',(206.038527625412,559.972556589211,-35.0982690928543)) ;
#73135=CARTESIAN_POINT('Origin',(203.056027625412,559.972556589211,-35.0982690928543)) ;
#73136=CARTESIAN_POINT('Origin',(206.038527625412,559.972556589211,-34.9732690928544)) ;
#73137=CARTESIAN_POINT('',(208.896027625412,559.972556589211,-36.8802690928544)) ;
#73138=CARTESIAN_POINT('Origin',(206.038527625412,559.972556589211,-36.8802690928544)) ;
#73139=CARTESIAN_POINT('',(208.896027625412,559.972556589211,-34.9732690928544)) ;
#73140=CARTESIAN_POINT('Origin',(206.038527625412,559.972556589211,-36.8802690928544)) ;
#73141=CARTESIAN_POINT('Origin',(208.771027625412,559.972556589211,-36.8802690928544)) ;
#73142=CARTESIAN_POINT('Origin',(206.038425919147,557.97255658921,-37.9581389501285)) ;
#73143=CARTESIAN_POINT('',(201.559777625412,557.97255658921,-40.5297040214914)) ;
#73144=CARTESIAN_POINT('Origin',(201.559777625412,558.097556589211,-40.5297040214914)) ;
#73145=CARTESIAN_POINT('Origin',(205.838527625413,569.472556589231,-35.0221601717609)) ;
#73146=CARTESIAN_POINT('',(203.155186246467,550.472556589211,-35.0221601717609)) ;
#73147=CARTESIAN_POINT('Origin',(206.03852762541,550.472556589211,-35.0221601717609)) ;
#73148=CARTESIAN_POINT('Origin',(206.03852762541,550.472556589211,-35.0982690928543)) ;
#73149=CARTESIAN_POINT('',(208.89602762541,550.472556589211,-35.0982690928543)) ;
#73150=CARTESIAN_POINT('',(203.18102762541,550.472556589211,-35.0982690928543)) ;
#73151=CARTESIAN_POINT('Origin',(206.03852762541,550.472556589211,-35.0982690928543)) ;
#73152=CARTESIAN_POINT('Origin',(206.03852762541,550.472556589211,-35.0982690928543)) ;
#73153=CARTESIAN_POINT('Origin',(203.05602762541,550.472556589211,-35.0982690928543)) ;
#73154=CARTESIAN_POINT('Origin',(206.03852762541,550.472556589211,-34.9732690928544)) ;
#73155=CARTESIAN_POINT('',(208.89602762541,550.472556589211,-36.8802690928544)) ;
#73156=CARTESIAN_POINT('Origin',(206.03852762541,550.472556589211,-36.8802690928544)) ;
#73157=CARTESIAN_POINT('',(208.89602762541,550.472556589211,-34.9732690928544)) ;
#73158=CARTESIAN_POINT('Origin',(206.03852762541,550.472556589211,-36.8802690928544)) ;
#73159=CARTESIAN_POINT('Origin',(208.77102762541,550.472556589211,-36.8802690928544)) ;
#73160=CARTESIAN_POINT('Origin',(206.038425919146,548.47255658921,-37.9581389501285)) ;
#73161=CARTESIAN_POINT('',(201.55977762541,548.47255658921,-40.5297040214914)) ;
#73162=CARTESIAN_POINT('Origin',(201.55977762541,548.59755658921,-40.5297040214914)) ;
#73163=CARTESIAN_POINT('Origin',(205.838527625413,569.472556589231,-35.0221601717609)) ;
#73164=CARTESIAN_POINT('',(203.155186246466,540.972556589211,-35.0221601717609)) ;
#73165=CARTESIAN_POINT('Origin',(206.038527625408,540.972556589211,-35.0221601717609)) ;
#73166=CARTESIAN_POINT('Origin',(206.038527625408,540.972556589211,-35.0982690928543)) ;
#73167=CARTESIAN_POINT('',(208.896027625408,540.972556589211,-35.0982690928543)) ;
#73168=CARTESIAN_POINT('',(203.181027625408,540.972556589211,-35.0982690928543)) ;
#73169=CARTESIAN_POINT('Origin',(206.038527625408,540.972556589211,-35.0982690928543)) ;
#73170=CARTESIAN_POINT('Origin',(206.038527625408,540.972556589211,-35.0982690928543)) ;
#73171=CARTESIAN_POINT('Origin',(203.056027625408,540.972556589211,-35.0982690928543)) ;
#73172=CARTESIAN_POINT('Origin',(206.038527625408,540.972556589211,-34.9732690928544)) ;
#73173=CARTESIAN_POINT('',(208.896027625408,540.972556589211,-36.8802690928544)) ;
#73174=CARTESIAN_POINT('Origin',(206.038527625408,540.972556589211,-36.8802690928544)) ;
#73175=CARTESIAN_POINT('',(208.896027625408,540.972556589211,-34.9732690928544)) ;
#73176=CARTESIAN_POINT('Origin',(206.038527625408,540.972556589211,-36.8802690928544)) ;
#73177=CARTESIAN_POINT('Origin',(208.771027625408,540.972556589211,-36.8802690928544)) ;
#73178=CARTESIAN_POINT('Origin',(206.038425919144,538.97255658921,-37.9581389501285)) ;
#73179=CARTESIAN_POINT('',(201.559777625409,538.97255658921,-40.5297040214914)) ;
#73180=CARTESIAN_POINT('Origin',(201.559777625409,539.09755658921,-40.5297040214914)) ;
#73181=CARTESIAN_POINT('Origin',(206.038527625407,531.472556589211,-35.0982690928543)) ;
#73182=CARTESIAN_POINT('',(208.896027625407,531.472556589211,-35.0982690928543)) ;
#73183=CARTESIAN_POINT('',(203.181027625407,531.472556589211,-35.0982690928543)) ;
#73184=CARTESIAN_POINT('Origin',(206.038527625407,531.472556589211,-35.0982690928543)) ;
#73185=CARTESIAN_POINT('Origin',(206.038527625407,531.472556589211,-35.0982690928543)) ;
#73186=CARTESIAN_POINT('Origin',(203.056027625407,531.472556589211,-35.0982690928543)) ;
#73187=CARTESIAN_POINT('Origin',(206.038527625407,531.472556589211,-34.9732690928544)) ;
#73188=CARTESIAN_POINT('',(208.896027625407,531.472556589211,-36.8802690928544)) ;
#73189=CARTESIAN_POINT('Origin',(206.038527625407,531.472556589211,-36.8802690928544)) ;
#73190=CARTESIAN_POINT('',(208.896027625407,531.472556589211,-34.9732690928544)) ;
#73191=CARTESIAN_POINT('Origin',(206.038527625407,531.472556589211,-36.8802690928544)) ;
#73192=CARTESIAN_POINT('Origin',(208.771027625407,531.472556589211,-36.8802690928544)) ;
#73193=CARTESIAN_POINT('Origin',(197.838527625421,612.722556589233,-25.0221601717606)) ;
#73194=CARTESIAN_POINT('',(212.588527625421,613.01056516053,-41.5221601717612)) ;
#73195=CARTESIAN_POINT('Origin',(212.588527625406,526.47255658921,-35.0221601717612)) ;
#73196=CARTESIAN_POINT('Origin',(209.81477762542,609.347556589211,-38.5610190928544)) ;
#73197=CARTESIAN_POINT('',(209.68977762542,609.347556589211,-38.5610190928544)) ;
#73198=CARTESIAN_POINT('Origin',(209.68977762542,602.868806589211,-43.1012690928544)) ;
#73199=CARTESIAN_POINT('',(209.68977762542,605.597556589211,-40.5297040214914)) ;
#73200=CARTESIAN_POINT('Origin',(209.81477762542,605.597556589211,-40.5297040214914)) ;
#73201=CARTESIAN_POINT('',(209.81477762542,605.472556589211,-40.5297040214914)) ;
#73202=CARTESIAN_POINT('Origin',(206.038425919156,605.472556589211,-37.9581389501285)) ;
#73203=CARTESIAN_POINT('Origin',(201.55977762542,609.347556589211,-38.5610190928544)) ;
#73204=CARTESIAN_POINT('Origin',(209.814777625418,599.847556589211,-38.5610190928544)) ;
#73205=CARTESIAN_POINT('',(209.689777625418,599.847556589211,-38.5610190928544)) ;
#73206=CARTESIAN_POINT('Origin',(209.689777625418,593.368806589211,-43.1012690928544)) ;
#73207=CARTESIAN_POINT('',(209.689777625418,596.097556589211,-40.5297040214914)) ;
#73208=CARTESIAN_POINT('Origin',(209.814777625418,596.097556589211,-40.5297040214914)) ;
#73209=CARTESIAN_POINT('',(209.814777625418,595.972556589211,-40.5297040214914)) ;
#73210=CARTESIAN_POINT('Origin',(206.038425919154,595.972556589211,-37.9581389501285)) ;
#73211=CARTESIAN_POINT('Origin',(201.559777625419,599.847556589211,-38.5610190928544)) ;
#73212=CARTESIAN_POINT('Origin',(209.814777625417,590.347556589211,-38.5610190928544)) ;
#73213=CARTESIAN_POINT('',(209.689777625417,590.347556589211,-38.5610190928544)) ;
#73214=CARTESIAN_POINT('Origin',(209.689777625417,583.868806589211,-43.1012690928544)) ;
#73215=CARTESIAN_POINT('',(209.689777625417,586.597556589211,-40.5297040214914)) ;
#73216=CARTESIAN_POINT('Origin',(209.814777625417,586.597556589211,-40.5297040214914)) ;
#73217=CARTESIAN_POINT('',(209.814777625417,586.472556589211,-40.5297040214914)) ;
#73218=CARTESIAN_POINT('Origin',(206.038425919152,586.472556589211,-37.9581389501285)) ;
#73219=CARTESIAN_POINT('Origin',(201.559777625417,590.347556589211,-38.5610190928544)) ;
#73220=CARTESIAN_POINT('Origin',(209.814777625415,580.847556589211,-38.5610190928544)) ;
#73221=CARTESIAN_POINT('',(209.689777625415,580.847556589211,-38.5610190928544)) ;
#73222=CARTESIAN_POINT('Origin',(209.689777625415,574.368806589211,-43.1012690928544)) ;
#73223=CARTESIAN_POINT('',(209.689777625415,577.097556589211,-40.5297040214914)) ;
#73224=CARTESIAN_POINT('Origin',(209.814777625415,577.097556589211,-40.5297040214914)) ;
#73225=CARTESIAN_POINT('',(209.814777625415,576.972556589211,-40.5297040214914)) ;
#73226=CARTESIAN_POINT('Origin',(206.038425919151,576.972556589211,-37.9581389501285)) ;
#73227=CARTESIAN_POINT('Origin',(201.559777625415,580.847556589211,-38.5610190928544)) ;
#73228=CARTESIAN_POINT('Origin',(209.814777625413,571.347556589211,-38.5610190928544)) ;
#73229=CARTESIAN_POINT('',(209.689777625413,571.347556589211,-38.5610190928544)) ;
#73230=CARTESIAN_POINT('Origin',(209.689777625413,564.868806589211,-43.1012690928544)) ;
#73231=CARTESIAN_POINT('',(209.689777625413,567.59755658921,-40.5297040214914)) ;
#73232=CARTESIAN_POINT('Origin',(209.814777625413,567.59755658921,-40.5297040214914)) ;
#73233=CARTESIAN_POINT('',(209.814777625413,567.47255658921,-40.5297040214914)) ;
#73234=CARTESIAN_POINT('Origin',(206.038425919149,567.47255658921,-37.9581389501285)) ;
#73235=CARTESIAN_POINT('Origin',(201.559777625414,571.347556589211,-38.5610190928544)) ;
#73236=CARTESIAN_POINT('Origin',(209.814777625412,561.847556589211,-38.5610190928544)) ;
#73237=CARTESIAN_POINT('',(209.689777625412,561.847556589211,-38.5610190928544)) ;
#73238=CARTESIAN_POINT('Origin',(209.689777625412,555.368806589211,-43.1012690928544)) ;
#73239=CARTESIAN_POINT('',(209.689777625412,558.097556589211,-40.5297040214914)) ;
#73240=CARTESIAN_POINT('Origin',(209.814777625412,558.097556589211,-40.5297040214914)) ;
#73241=CARTESIAN_POINT('',(209.814777625412,557.97255658921,-40.5297040214914)) ;
#73242=CARTESIAN_POINT('Origin',(206.038425919147,557.97255658921,-37.9581389501285)) ;
#73243=CARTESIAN_POINT('Origin',(201.559777625412,561.847556589211,-38.5610190928544)) ;
#73244=CARTESIAN_POINT('Origin',(209.81477762541,552.347556589211,-38.5610190928544)) ;
#73245=CARTESIAN_POINT('',(209.68977762541,552.347556589211,-38.5610190928544)) ;
#73246=CARTESIAN_POINT('Origin',(209.68977762541,545.868806589211,-43.1012690928544)) ;
#73247=CARTESIAN_POINT('',(209.68977762541,548.59755658921,-40.5297040214914)) ;
#73248=CARTESIAN_POINT('Origin',(209.81477762541,548.59755658921,-40.5297040214914)) ;
#73249=CARTESIAN_POINT('',(209.81477762541,548.47255658921,-40.5297040214914)) ;
#73250=CARTESIAN_POINT('Origin',(206.038425919146,548.47255658921,-37.9581389501285)) ;
#73251=CARTESIAN_POINT('Origin',(201.55977762541,552.347556589211,-38.5610190928544)) ;
#73252=CARTESIAN_POINT('Origin',(209.814777625408,542.847556589211,-38.5610190928544)) ;
#73253=CARTESIAN_POINT('',(209.689777625408,542.847556589211,-38.5610190928544)) ;
#73254=CARTESIAN_POINT('Origin',(209.689777625408,536.368806589211,-43.1012690928544)) ;
#73255=CARTESIAN_POINT('',(209.689777625408,539.09755658921,-40.5297040214914)) ;
#73256=CARTESIAN_POINT('Origin',(209.814777625408,539.09755658921,-40.5297040214914)) ;
#73257=CARTESIAN_POINT('',(209.814777625408,538.97255658921,-40.5297040214914)) ;
#73258=CARTESIAN_POINT('Origin',(206.038425919144,538.97255658921,-37.9581389501285)) ;
#73259=CARTESIAN_POINT('Origin',(201.559777625409,542.847556589211,-38.5610190928544)) ;
#86289=UNCERTAINTY_MEASURE_WITH_UNIT(LENGTH_MEASURE(0.01),#86331,
'DISTANCE_ACCURACY_VALUE',
'Maximum model space distance between geometric entities at asserted c
onnectivities') ;
#86304=UNCERTAINTY_MEASURE_WITH_UNIT(LENGTH_MEASURE(0.01),#86331,
'DISTANCE_ACCURACY_VALUE',
'Maximum model space distance between geometric entities at asserted c
onnectivities') ;
#86315=(
GEOMETRIC_REPRESENTATION_CONTEXT(3)
GLOBAL_UNCERTAINTY_ASSIGNED_CONTEXT((#86289))
GLOBAL_UNIT_ASSIGNED_CONTEXT((#86331,#86333,#86334))
REPRESENTATION_CONTEXT('','3D')
) ;
#86330=(
GEOMETRIC_REPRESENTATION_CONTEXT(3)
GLOBAL_UNCERTAINTY_ASSIGNED_CONTEXT((#86304))
GLOBAL_UNIT_ASSIGNED_CONTEXT((#86331,#86333,#86334))
REPRESENTATION_CONTEXT('','3D')
) ;
#86331=(
LENGTH_UNIT()
NAMED_UNIT(*)
SI_UNIT(.MILLI.,.METRE.)
) ;
#86333=(
NAMED_UNIT(*)
PLANE_ANGLE_UNIT()
SI_UNIT($,.RADIAN.)
) ;
#86334=(
NAMED_UNIT(*)
SI_UNIT($,.STERADIAN.)
SOLID_ANGLE_UNIT()
) ;
#86345=SHAPE_DEFINITION_REPRESENTATION(#86385,#86461) ;
#86385=PRODUCT_DEFINITION_SHAPE('',$,#86487) ;
#86461=SHAPE_REPRESENTATION('',(#33718),#86315) ;
#86476=PRODUCT_DEFINITION_CONTEXT('part definition',#86553,'design') ;
#86487=PRODUCT_DEFINITION('Insulator','Insulator',#86512,#86476) ;
#86512=PRODUCT_DEFINITION_FORMATION('',$,#86565) ;
#86553=APPLICATION_CONTEXT(
'Core Data for Automotive Mechanical Design Process') ;
#86554=PRODUCT_CONTEXT('part definition',#86553,'mechanical') ;
#86565=PRODUCT('Insulator','Insulator',$,(#86554)) ;
#86583=PRESENTATION_STYLE_ASSIGNMENT((#86588)) ;
#86588=SURFACE_STYLE_USAGE(.BOTH.,#86593) ;
#86593=SURFACE_SIDE_STYLE('',(#86598)) ;
#86598=SURFACE_STYLE_FILL_AREA(#86603) ;
#86603=FILL_AREA_STYLE('Opaque(42,42,42)',(#86608)) ;
#86608=FILL_AREA_STYLE_COLOUR('Opaque(42,42,42)',#86613) ;
#86613=COLOUR_RGB('Opaque(42,42,42)', 0.72549020, 0.75294118, 0.79215686) ;
ENDSEC;
END-ISO-10303-21;
